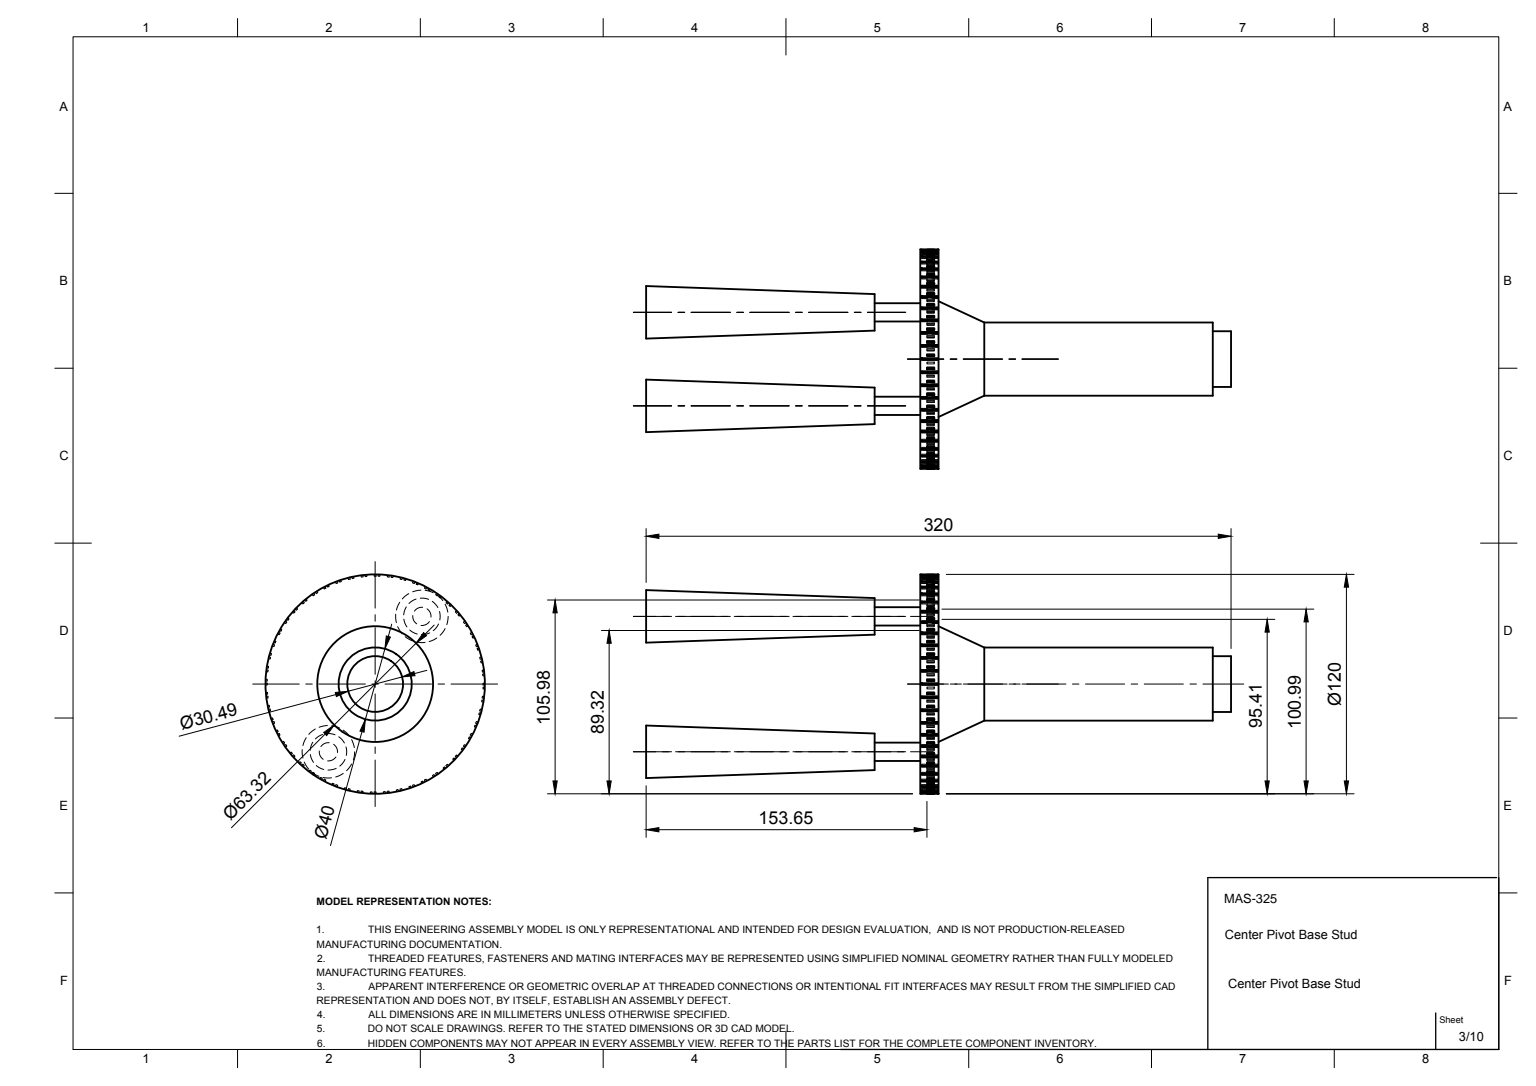
ISO-10303-21;
HEADER;
FILE_DESCRIPTION (('STEP AP214'),
    '1' );
FILE_NAME ('Center Pivot Base Stud.step',
    '2026-10-08T01:23:29',
    ( '' ),
    ( '' ),
    'SwSTEP 2.0',
    'SolidWorks 2025',
    '' );
FILE_SCHEMA (( 'AUTOMOTIVE_DESIGN' ));
ENDSEC;

DATA;
#6=EDGE_CURVE ( 'NONE', #30158, #26369, #45209, .T. ) ;
#7=DIRECTION ( 'NONE',  ( 1.000000000000000000, -0.000000000000000000, -0.000000000000000000 ) ) ;
#14=ORIENTED_EDGE ( 'NONE', *, *, #20809, .T. ) ;
#15=LINE ( 'NONE', #16057, #4072 ) ;
#25=CARTESIAN_POINT ( 'NONE',  ( -336.3521761649654422, -170.5607375887735770, 35.68215131113770155 ) ) ;
#29=DIRECTION ( 'NONE',  ( 0.000000000000000000, -0.3546048870425363986, -0.9350162426854146114 ) ) ;
#31=CARTESIAN_POINT ( 'NONE',  ( -339.1964088526558498, -131.1080185721124849, 58.50955523165764305 ) ) ;
#36=DIRECTION ( 'NONE',  ( -1.000000000000000000, -0.000000000000000000, -0.000000000000000000 ) ) ;
#38=( NAMED_UNIT ( * ) PLANE_ANGLE_UNIT ( ) SI_UNIT ( $, .RADIAN. ) );
#43=LINE ( 'NONE', #8442, #5592 ) ;
#45=ORIENTED_EDGE ( 'NONE', *, *, #35189, .T. ) ;
#47=FACE_OUTER_BOUND ( 'NONE', #8464, .T. ) ;
#52=DIRECTION ( 'NONE',  ( 0.000000000000000000, 1.341519488088730767E-14, -1.000000000000000000 ) ) ;
#54=AXIS2_PLACEMENT_3D ( 'NONE', #38179, #2187, #21657 ) ;
#55=CARTESIAN_POINT ( 'NONE',  ( -332.3517673607765914, -139.2044816956407089, -56.89493493766761389 ) ) ;
#59=CARTESIAN_POINT ( 'NONE',  ( -336.3521761649654422, -123.5000000000000284, 0.000000000000000000 ) ) ;
#60=CARTESIAN_POINT ( 'NONE',  ( -330.4913330509368166, -178.8432607619606358, 20.45418021416736565 ) ) ;
#64=ORIENTED_EDGE ( 'NONE', *, *, #9737, .T. ) ;
#65=CARTESIAN_POINT ( 'NONE',  ( -339.1964088526558498, -175.5095439275173135, 27.86139516340941213 ) ) ;
#66=CARTESIAN_POINT ( 'NONE',  ( -332.3517673607765914, -91.61526299123897843, -50.82679948493848343 ) ) ;
#69=VECTOR ( 'NONE', #22524, 1000.000000000000000 ) ;
#76=VERTEX_POINT ( 'NONE', #10211 ) ;
#77=VERTEX_POINT ( 'NONE', #49406 ) ;
#81=CARTESIAN_POINT ( 'NONE',  ( -330.4913330509368166, -183.4979166304964622, -0.4999999999999551470 ) ) ;
#87=LINE ( 'NONE', #8748, #33300 ) ;
#92=ORIENTED_EDGE ( 'NONE', *, *, #9964, .T. ) ;
#95=ORIENTED_EDGE ( 'NONE', *, *, #42836, .F. ) ;
#96=EDGE_CURVE ( 'NONE', #8568, #51994, #49908, .T. ) ;
#103=CARTESIAN_POINT ( 'NONE',  ( -336.3521761649654422, -123.5000000000000284, 0.000000000000000000 ) ) ;
#104=ORIENTED_EDGE ( 'NONE', *, *, #44978, .T. ) ;
#107=VECTOR ( 'NONE', #36864, 1000.000000000000000 ) ;
#110=DIRECTION ( 'NONE',  ( 1.000000000000000000, -0.000000000000000000, -0.000000000000000000 ) ) ;
#114=CARTESIAN_POINT ( 'NONE',  ( -339.1964088526558498, -122.9999999999993747, 59.00000000000002132 ) ) ;
#129=EDGE_LOOP ( 'NONE', ( #1022, #18617, #38243, #43508 ) ) ;
#135=ADVANCED_FACE ( 'NONE', ( #33613 ), #26232, .F. ) ;
#136=LINE ( 'NONE', #12733, #6804 ) ;
#141=EDGE_LOOP ( 'NONE', ( #33716, #13532, #31496, #14076 ) ) ;
#144=ADVANCED_FACE ( 'NONE', ( #30434 ), #14678, .T. ) ;
#146=DIRECTION ( 'NONE',  ( 0.000000000000000000, 0.000000000000000000, 1.000000000000000000 ) ) ;
#147=FACE_BOUND ( 'NONE', #3566, .T. ) ;
#149=EDGE_LOOP ( 'NONE', ( #37158, #34749, #12622, #8315 ) ) ;
#153=VERTEX_POINT ( 'NONE', #46748 ) ;
#154=CARTESIAN_POINT ( 'NONE',  ( -332.3517673607765914, -153.2494431741581025, -51.01861988938816950 ) ) ;
#155=EDGE_CURVE ( 'NONE', #5943, #22832, #22063, .T. ) ;
#160=ORIENTED_EDGE ( 'NONE', *, *, #6029, .T. ) ;
#161=LINE ( 'NONE', #28016, #26684 ) ;
#164=AXIS2_PLACEMENT_3D ( 'NONE', #24435, #20760, #36510 ) ;
#169=CARTESIAN_POINT ( 'NONE',  ( -336.3521761649654422, -161.4024510877913485, 45.24454186338643780 ) ) ;
#178=AXIS2_PLACEMENT_3D ( 'NONE', #15666, #4339, #31680 ) ;
#181=FACE_OUTER_BOUND ( 'NONE', #6191, .T. ) ;
#182=EDGE_CURVE ( 'NONE', #39742, #38924, #15463, .T. ) ;
#184=ADVANCED_FACE ( 'NONE', ( #15201 ), #27530, .F. ) ;
#186=VERTEX_POINT ( 'NONE', #51463 ) ;
#190=EDGE_LOOP ( 'NONE', ( #41506, #8467, #35219, #32996 ) ) ;
#191=AXIS2_PLACEMENT_3D ( 'NONE', #6779, #42505, #19123 ) ;
#197=ORIENTED_EDGE ( 'NONE', *, *, #15389, .T. ) ;
#198=ADVANCED_FACE ( 'NONE', ( #19392 ), #26495, .F. ) ;
#199=EDGE_LOOP ( 'NONE', ( #48171, #38497, #32246, #32492 ) ) ;
#200=DIRECTION ( 'NONE',  ( 0.000000000000000000, 0.2393156642875615969, 0.9709418174260511236 ) ) ;
#201=CARTESIAN_POINT ( 'NONE',  ( -339.1964088526558498, -180.9052250602809977, -13.63415328425247885 ) ) ;
#206=CARTESIAN_POINT ( 'NONE',  ( -332.3517673607765914, -86.34605966037949543, -45.90766452162698386 ) ) ;
#208=DIRECTION ( 'NONE',  ( 0.000000000000000000, 0.000000000000000000, 1.000000000000000000 ) ) ;
#214=CARTESIAN_POINT ( 'NONE',  ( -339.1964088526558498, -157.4273119900853146, -48.27201571435997352 ) ) ;
#216=CARTESIAN_POINT ( 'NONE',  ( -339.1964088526558498, -83.33976666098951114, 44.57752413667933666 ) ) ;
#217=ORIENTED_EDGE ( 'NONE', *, *, #6337, .T. ) ;
#222=DIRECTION ( 'NONE',  ( -0.000000000000000000, 0.2393156642875685636, 0.9709418174260492362 ) ) ;
#228=DIRECTION ( 'NONE',  ( 0.000000000000000000, 0.000000000000000000, 1.000000000000000000 ) ) ;
#232=VERTEX_POINT ( 'NONE', #18624 ) ;
#233=FACE_OUTER_BOUND ( 'NONE', #34259, .T. ) ;
#240=EDGE_CURVE ( 'NONE', #16530, #9197, #11238, .T. ) ;
#242=CYLINDRICAL_SURFACE ( 'NONE', #15746, 20.00000000000001066 ) ;
#256=DIRECTION ( 'NONE',  ( -0.000000000000000000, 0.8229838658936556861, -0.5680647467311569221 ) ) ;
#259=EDGE_CURVE ( 'NONE', #47910, #27371, #721, .T. ) ;
#260=CARTESIAN_POINT ( 'NONE',  ( -332.3517673607765914, -133.2247606357419443, -58.25253621232173629 ) ) ;
#261=ORIENTED_EDGE ( 'NONE', *, *, #51004, .T. ) ;
#264=EDGE_CURVE ( 'NONE', #15715, #30086, #23588, .T. ) ;
#269=ORIENTED_EDGE ( 'NONE', *, *, #12211, .F. ) ;
#276=ORIENTED_EDGE ( 'NONE', *, *, #30764, .F. ) ;
#284=LINE ( 'NONE', #32615, #29005 ) ;
#286=EDGE_CURVE ( 'NONE', #41564, #12706, #20162, .T. ) ;
#288=CARTESIAN_POINT ( 'NONE',  ( -332.3517673607765914, -139.4384828369889249, -57.84431488793872944 ) ) ;
#290=LINE ( 'NONE', #41018, #22829 ) ;
#298=CARTESIAN_POINT ( 'NONE',  ( -332.3517673607765914, -70.03480886230919111, 25.08789112700620194 ) ) ;
#301=ORIENTED_EDGE ( 'NONE', *, *, #17600, .T. ) ;
#304=VECTOR ( 'NONE', #6008, 999.9999999999998863 ) ;
#305=EDGE_CURVE ( 'NONE', #49014, #8114, #15730, .T. ) ;
#306=CARTESIAN_POINT ( 'NONE',  ( -305.0000000000000568, -71.64707600775140861, -30.18731974611341684 ) ) ;
#308=DIRECTION ( 'NONE',  ( -1.000000000000000000, 0.000000000000000000, 0.000000000000000000 ) ) ;
#315=LINE ( 'NONE', #15321, #378 ) ;
#316=CARTESIAN_POINT ( 'NONE',  ( -330.4913330509368166, -109.8658467157472813, -57.40522506028090532 ) ) ;
#325=DIRECTION ( 'NONE',  ( 0.000000000000000000, 0.2393156642875516049, -0.9709418174260534551 ) ) ;
#329=ORIENTED_EDGE ( 'NONE', *, *, #42921, .T. ) ;
#333=CARTESIAN_POINT ( 'NONE',  ( -330.4913330509368166, -75.22798428563987727, -33.92731199008506593 ) ) ;
#338=VECTOR ( 'NONE', #11663, 1000.000000000000000 ) ;
#339=ORIENTED_EDGE ( 'NONE', *, *, #31396, .F. ) ;
#340=CARTESIAN_POINT ( 'NONE',  ( -339.1964088526558498, -137.1341532842523065, 57.40522506028101901 ) ) ;
#343=CARTESIAN_POINT ( 'NONE',  ( -332.3517673607765914, -126.1322888500942270, -59.00000000000001421 ) ) ;
#344=DIRECTION ( 'NONE',  ( -1.000000000000000000, 0.000000000000000000, 0.000000000000000000 ) ) ;
#350=CARTESIAN_POINT ( 'NONE',  ( -332.3517673607765914, -65.24746378767824240, -9.724760635741734660 ) ) ;
#353=CARTESIAN_POINT ( 'NONE',  ( -332.3517673607765914, -135.2893155068536828, 58.83036664750491695 ) ) ;
#356=VECTOR ( 'NONE', #3324, 1000.000000000000000 ) ;
#358=ORIENTED_EDGE ( 'NONE', *, *, #16677, .F. ) ;
#359=DIRECTION ( 'NONE',  ( 1.000000000000000000, -0.000000000000000000, -0.000000000000000000 ) ) ;
#364=DIRECTION ( 'NONE',  ( -0.000000000000000000, -0.9350162426854132791, 0.3546048870425396182 ) ) ;
#365=CARTESIAN_POINT ( 'NONE',  ( -330.4913330509368166, -145.2430625708875880, -55.92172413327818958 ) ) ;
#366=DIRECTION ( 'NONE',  ( -8.718379230999707126E-17, 0.7485107481711024136, 0.6631226582407937498 ) ) ;
#368=EDGE_CURVE ( 'NONE', #39057, #30451, #5316, .T. ) ;
#369=LINE ( 'NONE', #36375, #20714 ) ;
#371=CARTESIAN_POINT ( 'NONE',  ( -336.3521761649654422, -135.0638248728647852, 57.91551518289418254 ) ) ;
#372=EDGE_LOOP ( 'NONE', ( #12308, #32950, #15983, #21673 ) ) ;
#373=ORIENTED_EDGE ( 'NONE', *, *, #33329, .T. ) ;
#374=DIRECTION ( 'NONE',  ( 0.000000000000000000, 0.7485107481711000821, -0.6631226582407965253 ) ) ;
#376=ORIENTED_EDGE ( 'NONE', *, *, #30512, .F. ) ;
#378=VECTOR ( 'NONE', #32371, 1000.000000000000114 ) ;
#379=EDGE_LOOP ( 'NONE', ( #7863, #48040, #19439, #9554 ) ) ;
#383=EDGE_LOOP ( 'NONE', ( #92, #27260, #27029, #39388 ) ) ;
#386=ORIENTED_EDGE ( 'NONE', *, *, #9915, .F. ) ;
#387=CARTESIAN_POINT ( 'NONE',  ( -339.1964088526558498, -123.5000000000000284, 0.000000000000000000 ) ) ;
#392=ORIENTED_EDGE ( 'NONE', *, *, #15989, .F. ) ;
#395=ORIENTED_EDGE ( 'NONE', *, *, #34509, .F. ) ;
#398=CARTESIAN_POINT ( 'NONE',  ( -332.3517673607765914, -174.5186198893880771, 29.74944317415823392 ) ) ;
#399=FACE_BOUND ( 'NONE', #32267, .T. ) ;
#400=DIRECTION ( 'NONE',  ( 0.000000000000000000, -0.8854560256532110207, -0.4647231720437664526 ) ) ;
#401=ORIENTED_EDGE ( 'NONE', *, *, #48751, .T. ) ;
#402=EDGE_CURVE ( 'NONE', #42461, #43377, #31986, .T. ) ;
#403=ORIENTED_EDGE ( 'NONE', *, *, #7972, .T. ) ;
#407=AXIS2_PLACEMENT_3D ( 'NONE', #634, #16408, #32423 ) ;
#412=CARTESIAN_POINT ( 'NONE',  ( -339.1964088526558498, -171.7720157143598669, 33.92731199008546383 ) ) ;
#422=DIRECTION ( 'NONE',  ( -0.000000000000000000, 0.2393156642875685636, 0.9709418174260492362 ) ) ;
#428=EDGE_CURVE ( 'NONE', #27513, #27045, #24890, .T. ) ;
#431=CARTESIAN_POINT ( 'NONE',  ( -305.0000000000000568, -104.7054247829104270, -56.98038208374144631 ) ) ;
#438=CARTESIAN_POINT ( 'NONE',  ( -332.3517673607765914, -64.87442053112221174, 12.76876783163883466 ) ) ;
#445=LINE ( 'NONE', #39606, #1079 ) ;
#446=ORIENTED_EDGE ( 'NONE', *, *, #50072, .F. ) ;
#448=VECTOR ( 'NONE', #9806, 999.9999999999998863 ) ;
#449=CIRCLE ( 'NONE', #45791, 60.00000000000000000 ) ;
#453=DIRECTION ( 'NONE',  ( -1.000000000000000000, -0.000000000000000000, 0.000000000000000000 ) ) ;
#458=LINE ( 'NONE', #21229, #24488 ) ;
#473=CARTESIAN_POINT ( 'NONE',  ( -305.0000000000000568, -150.9396941197155968, -53.35787839313373127 ) ) ;
#479=ORIENTED_EDGE ( 'NONE', *, *, #35123, .F. ) ;
#483=LINE ( 'NONE', #20735, #14074 ) ;
#491=DIRECTION ( 'NONE',  ( 0.000000000000000000, -0.4647231720437664526, 0.8854560256532110207 ) ) ;
#495=ORIENTED_EDGE ( 'NONE', *, *, #20083, .F. ) ;
#497=EDGE_CURVE ( 'NONE', #30653, #14763, #4477, .T. ) ;
#499=AXIS2_PLACEMENT_3D ( 'NONE', #42166, #25251, #24463 ) ;
#504=ORIENTED_EDGE ( 'NONE', *, *, #17516, .T. ) ;
#506=ORIENTED_EDGE ( 'NONE', *, *, #34160, .T. ) ;
#510=CARTESIAN_POINT ( 'NONE',  ( -336.3521761649654422, -87.81784868886214213, 47.06073758877343494 ) ) ;
#513=CARTESIAN_POINT ( 'NONE',  ( -330.4913330509368166, -89.82879061784696262, -49.66134974749687103 ) ) ;
#521=DIRECTION ( 'NONE',  ( 1.000000000000000000, -0.000000000000000000, -0.000000000000000000 ) ) ;
#522=AXIS2_PLACEMENT_3D ( 'NONE', #5834, #21590, #45254 ) ;
#526=LINE ( 'NONE', #16591, #33385 ) ;
#527=ORIENTED_EDGE ( 'NONE', *, *, #25028, .F. ) ;
#531=DIRECTION ( 'NONE',  ( 0.000000000000000000, 0.000000000000000000, -1.000000000000000000 ) ) ;
#534=DIRECTION ( 'NONE',  ( -1.000000000000000000, 0.000000000000000000, 0.000000000000000000 ) ) ;
#536=EDGE_LOOP ( 'NONE', ( #8280, #13076, #45536, #37068 ) ) ;
#538=ADVANCED_FACE ( 'NONE', ( #9385 ), #38000, .T. ) ;
#539=ADVANCED_FACE ( 'NONE', ( #1222 ), #33292, .T. ) ;
#544=CARTESIAN_POINT ( 'NONE',  ( -330.4913330509368166, -96.52406086224436876, -52.47426709956133806 ) ) ;
#548=DIRECTION ( 'NONE',  ( 0.000000000000000000, 1.156482317317871449E-14, 1.000000000000000000 ) ) ;
#549=CARTESIAN_POINT ( 'NONE',  ( -336.3521761649654422, -94.63601285149479736, 51.48334306143172512 ) ) ;
#552=EDGE_CURVE ( 'NONE', #15284, #26962, #8852, .T. ) ;
#557=ORIENTED_EDGE ( 'NONE', *, *, #40396, .F. ) ;
#559=EDGE_CURVE ( 'NONE', #4633, #10838, #13706, .T. ) ;
#566=AXIS2_PLACEMENT_3D ( 'NONE', #47062, #11037, #17979 ) ;
#567=VECTOR ( 'NONE', #28228, 1000.000000000000000 ) ;
#569=CARTESIAN_POINT ( 'NONE',  ( -339.1964088526558498, -84.75001853787809125, 44.49369547121489887 ) ) ;
#575=FACE_OUTER_BOUND ( 'NONE', #48196, .T. ) ;
#578=CARTESIAN_POINT ( 'NONE',  ( -330.4913330509368166, -157.4273119900845757, 48.27201571436049932 ) ) ;
#579=PLANE ( 'NONE',  #5256 ) ;
#582=VECTOR ( 'NONE', #15550, 1000.000000000000000 ) ;
#584=ORIENTED_EDGE ( 'NONE', *, *, #37671, .T. ) ;
#590=ORIENTED_EDGE ( 'NONE', *, *, #34142, .F. ) ;
#595=DIRECTION ( 'NONE',  ( -1.000000000000000000, 0.000000000000000000, -0.000000000000000000 ) ) ;
#607=CARTESIAN_POINT ( 'NONE',  ( -330.4913330509368166, -108.6560878169896256, 58.13482838284702581 ) ) ;
#617=EDGE_CURVE ( 'NONE', #30167, #21474, #51158, .T. ) ;
#619=CIRCLE ( 'NONE', #20770, 60.00000000000000000 ) ;
#620=ORIENTED_EDGE ( 'NONE', *, *, #35779, .F. ) ;
#623=CONICAL_SURFACE ( 'NONE', #29126, 10.00000000000000711, 0.03490658503988659789 ) ;
#625=EDGE_CURVE ( 'NONE', #8999, #27120, #46420, .T. ) ;
#626=EDGE_CURVE ( 'NONE', #50991, #48252, #50369, .T. ) ;
#629=DIRECTION ( 'NONE',  ( -1.000000000000000000, -0.000000000000000000, 0.000000000000000000 ) ) ;
#631=CARTESIAN_POINT ( 'NONE',  ( -365.0000000000001137, -78.50000000000002842, 0.000000000000000000 ) ) ;
#632=AXIS2_PLACEMENT_3D ( 'NONE', #7367, #43090, #14727 ) ;
#634=CARTESIAN_POINT ( 'NONE',  ( 0.000000000000000000, -162.6242368362065918, 44.16213414209531862 ) ) ;
#640=LINE ( 'NONE', #48731, #27621 ) ;
#647=DIRECTION ( 'NONE',  ( 0.000000000000000000, 0.1205366802553164696, -0.9927088740980548609 ) ) ;
#648=DIRECTION ( 'NONE',  ( 0.000000000000000000, 0.000000000000000000, -1.000000000000000000 ) ) ;
#658=ORIENTED_EDGE ( 'NONE', *, *, #5431, .T. ) ;
#660=DIRECTION ( 'NONE',  ( -0.000000000000000000, 0.6631226582407863113, -0.7485107481711089639 ) ) ;
#662=DIRECTION ( 'NONE',  ( -1.000000000000000000, 0.000000000000000000, -0.000000000000000000 ) ) ;
#663=VECTOR ( 'NONE', #44301, 1000.000000000000000 ) ;
#667=CARTESIAN_POINT ( 'NONE',  ( -330.4913330509368166, -150.4759391377553186, 52.47426709956150859 ) ) ;
#670=DIRECTION ( 'NONE',  ( -0.000000000000000000, 1.000000000000000000, -0.000000000000000000 ) ) ;
#674=VECTOR ( 'NONE', #17108, 1000.000000000000000 ) ;
#678=CARTESIAN_POINT ( 'NONE',  ( -305.0000000000000568, -123.5000000000000284, 0.000000000000000000 ) ) ;
#680=ORIENTED_EDGE ( 'NONE', *, *, #28374, .T. ) ;
#681=EDGE_CURVE ( 'NONE', #49313, #49622, #43755, .T. ) ;
#687=VECTOR ( 'NONE', #26344, 999.9999999999998863 ) ;
#693=VECTOR ( 'NONE', #26320, 1000.000000000000000 ) ;
#696=ORIENTED_EDGE ( 'NONE', *, *, #41387, .T. ) ;
#699=ORIENTED_EDGE ( 'NONE', *, *, #15129, .T. ) ;
#700=DIRECTION ( 'NONE',  ( 0.000000000000000000, -0.8854560256532093554, 0.4647231720437695057 ) ) ;
#706=CARTESIAN_POINT ( 'NONE',  ( -336.3521761649654422, -64.50000000000000000, -2.632288850093980503 ) ) ;
#711=LINE ( 'NONE', #28547, #40806 ) ;
#719=DIRECTION ( 'NONE',  ( 1.000000000000000000, 0.000000000000000000, 0.000000000000000000 ) ) ;
#720=ORIENTED_EDGE ( 'NONE', *, *, #4486, .T. ) ;
#721=LINE ( 'NONE', #24371, #22893 ) ;
#722=EDGE_LOOP ( 'NONE', ( #13255, #44779, #48049, #3646 ) ) ;
#724=AXIS2_PLACEMENT_3D ( 'NONE', #34745, #11088, #18732 ) ;
#725=VECTOR ( 'NONE', #35694, 1000.000000000000114 ) ;
#727=CARTESIAN_POINT ( 'NONE',  ( -330.4913330509368166, -131.1080185721124849, 58.50955523165764305 ) ) ;
#730=CARTESIAN_POINT ( 'NONE',  ( -332.3517673607765914, -170.5607375887735770, 35.68215131113770155 ) ) ;
#734=VECTOR ( 'NONE', #15159, 1000.000000000000000 ) ;
#739=DIRECTION ( 'NONE',  ( 1.000000000000000000, -7.719741424018441012E-17, 4.051632851310786670E-17 ) ) ;
#740=ADVANCED_FACE ( 'NONE', ( #35605 ), #3552, .F. ) ;
#748=ORIENTED_EDGE ( 'NONE', *, *, #46870, .F. ) ;
#750=EDGE_LOOP ( 'NONE', ( #47763, #48042, #43578, #36505 ) ) ;
#753=FACE_OUTER_BOUND ( 'NONE', #12516, .T. ) ;
#756=DIRECTION ( 'NONE',  ( 1.000000000000000000, -0.000000000000000000, 0.000000000000000000 ) ) ;
#759=ORIENTED_EDGE ( 'NONE', *, *, #12652, .T. ) ;
#761=CARTESIAN_POINT ( 'NONE',  ( -339.1964088526558498, -137.1341532842523065, 57.40522506028101901 ) ) ;
#764=CARTESIAN_POINT ( 'NONE',  ( -330.4913330509368166, -102.1108035431471279, 54.98865587491800255 ) ) ;
#771=LINE ( 'NONE', #21264, #26347 ) ;
#772=CARTESIAN_POINT ( 'NONE',  ( -339.1964088526558498, -79.66942718702493664, 39.49849221029193558 ) ) ;
#778=FACE_OUTER_BOUND ( 'NONE', #41872, .T. ) ;
#785=LINE ( 'NONE', #510, #16196 ) ;
#788=EDGE_CURVE ( 'NONE', #45751, #9248, #24559, .T. ) ;
#789=CARTESIAN_POINT ( 'NONE',  ( -330.4913330509368166, -183.1207326066167411, -6.735595255826296146 ) ) ;
#793=EDGE_CURVE ( 'NONE', #5683, #31493, #23789, .T. ) ;
#795=AXIS2_PLACEMENT_3D ( 'NONE', #19587, #662, #28498 ) ;
#798=VECTOR ( 'NONE', #3197, 1000.000000000000000 ) ;
#803=CARTESIAN_POINT ( 'NONE',  ( -332.3517673607765914, -100.1170788342122080, 54.23253582808833073 ) ) ;
#804=LINE ( 'NONE', #44961, #32554 ) ;
#809=VERTEX_POINT ( 'NONE', #15919 ) ;
#814=CARTESIAN_POINT ( 'NONE',  ( -339.1964088526558498, -175.9742670995615015, -26.97593913775538965 ) ) ;
#815=DIRECTION ( 'NONE',  ( -1.000000000000000000, -0.000000000000000000, -0.000000000000000000 ) ) ;
#816=ORIENTED_EDGE ( 'NONE', *, *, #28380, .T. ) ;
#820=DIRECTION ( 'NONE',  ( -0.000000000000000000, -0.9350162426854169428, -0.3546048870425300148 ) ) ;
#821=ORIENTED_EDGE ( 'NONE', *, *, #21477, .T. ) ;
#822=EDGE_CURVE ( 'NONE', #37318, #29662, #44017, .T. ) ;
#824=LINE ( 'NONE', #19745, #7267 ) ;
#825=FACE_OUTER_BOUND ( 'NONE', #25719, .T. ) ;
#826=ORIENTED_EDGE ( 'NONE', *, *, #45474, .F. ) ;
#830=CIRCLE ( 'NONE', #7550, 60.00000000000000000 ) ;
#831=LINE ( 'NONE', #36308, #22296 ) ;
#841=ORIENTED_EDGE ( 'NONE', *, *, #9249, .F. ) ;
#843=EDGE_CURVE ( 'NONE', #40953, #1071, #11946, .T. ) ;
#844=CARTESIAN_POINT ( 'NONE',  ( -336.3521761649654422, -123.5000000000000284, 0.000000000000000000 ) ) ;
#847=DIRECTION ( 'NONE',  ( 0.000000000000000000, 0.7485107481711089639, 0.6631226582407863113 ) ) ;
#852=EDGE_CURVE ( 'NONE', #6390, #47279, #33225, .T. ) ;
#855=ORIENTED_EDGE ( 'NONE', *, *, #4126, .F. ) ;
#857=EDGE_CURVE ( 'NONE', #42035, #39327, #29921, .T. ) ;
#862=VECTOR ( 'NONE', #6226, 1000.000000000000000 ) ;
#863=DIRECTION ( 'NONE',  ( 0.000000000000000000, 0.5680647467311540355, -0.8229838658936575735 ) ) ;
#865=DIRECTION ( 'NONE',  ( 0.000000000000000000, -0.8854560256532062468, 0.4647231720437755564 ) ) ;
#868=PLANE ( 'NONE',  #25728 ) ;
#872=ORIENTED_EDGE ( 'NONE', *, *, #17504, .T. ) ;
#873=FACE_OUTER_BOUND ( 'NONE', #29196, .T. ) ;
#879=FACE_BOUND ( 'NONE', #13817, .T. ) ;
#880=LINE ( 'NONE', #29514, #15543 ) ;
#884=PLANE ( 'NONE',  #11452 ) ;
#888=EDGE_LOOP ( 'NONE', ( #12030, #10347, #16731, #21899 ) ) ;
#892=DIRECTION ( 'NONE',  ( -0.000000000000000000, -0.1205366802553233113, -0.9927088740980538617 ) ) ;
#893=EDGE_LOOP ( 'NONE', ( #26823, #18504, #1153, #44757 ) ) ;
#898=VECTOR ( 'NONE', #3315, 1000.000000000000000 ) ;
#899=LINE ( 'NONE', #29006, #1687 ) ;
#900=CARTESIAN_POINT ( 'NONE',  ( -332.3517673607765914, -182.3871109312487420, -4.498567634386014369 ) ) ;
#901=EDGE_LOOP ( 'NONE', ( #1534, #46424, #46077, #38731 ) ) ;
#903=VERTEX_POINT ( 'NONE', #16950 ) ;
#907=ADVANCED_FACE ( 'NONE', ( #17209 ), #33746, .T. ) ;
#916=EDGE_CURVE ( 'NONE', #37855, #15026, #32709, .T. ) ;
#917=FACE_OUTER_BOUND ( 'NONE', #10592, .T. ) ;
#919=ORIENTED_EDGE ( 'NONE', *, *, #27607, .F. ) ;
#928=FACE_BOUND ( 'NONE', #50304, .T. ) ;
#931=ADVANCED_FACE ( 'NONE', ( #48753 ), #49009, .F. ) ;
#942=CARTESIAN_POINT ( 'NONE',  ( -365.0000000000001137, -78.50000000000002842, 0.000000000000000000 ) ) ;
#945=EDGE_LOOP ( 'NONE', ( #3380, #48657, #41462, #10623 ) ) ;
#957=AXIS2_PLACEMENT_3D ( 'NONE', #26370, #34508, #6419 ) ;
#960=ORIENTED_EDGE ( 'NONE', *, *, #47532, .T. ) ;
#965=ORIENTED_EDGE ( 'NONE', *, *, #13376, .F. ) ;
#966=EDGE_CURVE ( 'NONE', #23416, #47681, #16330, .T. ) ;
#969=VECTOR ( 'NONE', #7507, 1000.000000000000114 ) ;
#972=LINE ( 'NONE', #4397, #37714 ) ;
#977=ORIENTED_EDGE ( 'NONE', *, *, #49157, .F. ) ;
#978=VERTEX_POINT ( 'NONE', #36552 ) ;
#981=CARTESIAN_POINT ( 'NONE',  ( -339.1964088526558498, -137.3729703655840524, -58.37414404713467064 ) ) ;
#982=ADVANCED_FACE ( 'NONE', ( #8191 ), #44714, .F. ) ;
#988=VECTOR ( 'NONE', #34553, 1000.000000000000000 ) ;
#995=DIRECTION ( 'NONE',  ( -1.000000000000000000, -0.000000000000000000, -0.000000000000000000 ) ) ;
#1000=CARTESIAN_POINT ( 'NONE',  ( -336.3521761649654422, -77.59233547837267508, 37.15394033962009246 ) ) ;
#1001=VERTEX_POINT ( 'NONE', #8705 ) ;
#1003=DIRECTION ( 'NONE',  ( 0.000000000000000000, -0.7485107481711046340, -0.6631226582407911962 ) ) ;
#1008=ORIENTED_EDGE ( 'NONE', *, *, #2527, .F. ) ;
#1009=LINE ( 'NONE', #40954, #47226 ) ;
#1010=AXIS2_PLACEMENT_3D ( 'NONE', #24316, #19851, #28247 ) ;
#1016=DIRECTION ( 'NONE',  ( -0.000000000000000000, -0.6631226582407989678, -0.7485107481710977506 ) ) ;
#1021=CARTESIAN_POINT ( 'NONE',  ( -336.3521761649654422, -136.0347666902908372, 57.67619951860663718 ) ) ;
#1022=ORIENTED_EDGE ( 'NONE', *, *, #4950, .T. ) ;
#1023=AXIS2_PLACEMENT_3D ( 'NONE', #28600, #25706, #21511 ) ;
#1025=LINE ( 'NONE', #25468, #35362 ) ;
#1026=ORIENTED_EDGE ( 'NONE', *, *, #19388, .F. ) ;
#1027=EDGE_CURVE ( 'NONE', #12239, #8561, #37458, .T. ) ;
#1033=CARTESIAN_POINT ( 'NONE',  ( -336.3521761649653854, -167.3116148657362032, 40.99441916720376611 ) ) ;
#1036=DIRECTION ( 'NONE',  ( -1.000000000000000000, -0.000000000000000000, -0.000000000000000000 ) ) ;
#1046=VECTOR ( 'NONE', #42393, 999.9999999999998863 ) ;
#1049=DIRECTION ( 'NONE',  ( 1.000000000000000000, -0.000000000000000000, -0.000000000000000000 ) ) ;
#1050=CARTESIAN_POINT ( 'NONE',  ( 0.000000000000000000, -66.21443277186293130, -14.11962419296594362 ) ) ;
#1051=CARTESIAN_POINT ( 'NONE',  ( -330.4913330509368166, -138.1050951016791544, -57.16590939599326049 ) ) ;
#1053=DIRECTION ( 'NONE',  ( 0.000000000000000000, -0.9927088740980526405, 0.1205366802553337890 ) ) ;
#1054=ORIENTED_EDGE ( 'NONE', *, *, #47532, .F. ) ;
#1055=CARTESIAN_POINT ( 'NONE',  ( -330.4913330509368166, -162.9984922102926532, -43.83057281297441676 ) ) ;
#1056=ORIENTED_EDGE ( 'NONE', *, *, #35004, .T. ) ;
#1061=EDGE_CURVE ( 'NONE', #49231, #23542, #43, .T. ) ;
#1064=CYLINDRICAL_SURFACE ( 'NONE', #42444, 5.000000000000001776 ) ;
#1068=CARTESIAN_POINT ( 'NONE',  ( -339.1964088526558498, -64.50000000000000000, -0.5000000000000457412 ) ) ;
#1071=VERTEX_POINT ( 'NONE', #12382 ) ;
#1075=DIRECTION ( 'NONE',  ( 1.000000000000000000, 0.000000000000000000, -0.000000000000000000 ) ) ;
#1079=VECTOR ( 'NONE', #40641, 1000.000000000000000 ) ;
#1081=EDGE_CURVE ( 'NONE', #19973, #15758, #3891, .T. ) ;
#1085=FACE_OUTER_BOUND ( 'NONE', #1756, .T. ) ;
#1089=EDGE_CURVE ( 'NONE', #49077, #5683, #4772, .T. ) ;
#1091=ADVANCED_FACE ( 'NONE', ( #36295 ), #4248, .F. ) ;
#1096=AXIS2_PLACEMENT_3D ( 'NONE', #11928, #27966, #43997 ) ;
#1097=ORIENTED_EDGE ( 'NONE', *, *, #46194, .T. ) ;
#1100=CARTESIAN_POINT ( 'NONE',  ( -336.3521761649654422, -105.0395444947681369, -56.09938080879045685 ) ) ;
#1102=ORIENTED_EDGE ( 'NONE', *, *, #37849, .T. ) ;
#1103=EDGE_LOOP ( 'NONE', ( #16367, #2047, #5944, #42627, #29836, #15506, #24590, #45361, #42114, #27008, #14441, #17020 ) ) ;
#1105=EDGE_CURVE ( 'NONE', #9161, #6831, #824, .T. ) ;
#1107=DIRECTION ( 'NONE',  ( -0.000000000000000000, -0.2393156642875615969, -0.9709418174260511236 ) ) ;
#1113=AXIS2_PLACEMENT_3D ( 'NONE', #40879, #12244, #40608 ) ;
#1114=CARTESIAN_POINT ( 'NONE',  ( 0.000000000000000000, -89.98417994286192823, -48.55604808772582004 ) ) ;
#1128=VECTOR ( 'NONE', #19899, 1000.000000000000000 ) ;
#1133=CARTESIAN_POINT ( 'NONE',  ( -336.3521761649654422, -87.28260048324005993, 47.83617848703422482 ) ) ;
#1134=DIRECTION ( 'NONE',  ( 0.000000000000000000, 0.000000000000000000, 1.000000000000000000 ) ) ;
#1140=CARTESIAN_POINT ( 'NONE',  ( -332.3517673607765914, -158.3591674452439122, -47.62880233550485087 ) ) ;
#1143=PLANE ( 'NONE',  #12243 ) ;
#1145=LINE ( 'NONE', #9828, #29943 ) ;
#1148=CARTESIAN_POINT ( 'NONE',  ( -336.3521761649654422, -86.34605966037949543, -45.90766452162698386 ) ) ;
#1149=EDGE_CURVE ( 'NONE', #43162, #33480, #21057, .T. ) ;
#1152=ORIENTED_EDGE ( 'NONE', *, *, #33748, .T. ) ;
#1153=ORIENTED_EDGE ( 'NONE', *, *, #48129, .F. ) ;
#1154=EDGE_CURVE ( 'NONE', #5750, #45751, #25513, .T. ) ;
#1157=ORIENTED_EDGE ( 'NONE', *, *, #23110, .F. ) ;
#1158=EDGE_CURVE ( 'NONE', #13843, #41304, #13691, .T. ) ;
#1161=DIRECTION ( 'NONE',  ( 1.000000000000000000, -0.000000000000000000, -0.000000000000000000 ) ) ;
#1163=VERTEX_POINT ( 'NONE', #29709 ) ;
#1165=EDGE_LOOP ( 'NONE', ( #35019, #7711, #18752, #10228 ) ) ;
#1168=AXIS2_PLACEMENT_3D ( 'NONE', #5085, #48965, #865 ) ;
#1170=PLANE ( 'NONE',  #26072 ) ;
#1172=ORIENTED_EDGE ( 'NONE', *, *, #26251, .T. ) ;
#1173=ORIENTED_EDGE ( 'NONE', *, *, #32356, .T. ) ;
#1183=CARTESIAN_POINT ( 'NONE',  ( -339.1964088526558498, -179.7763290203209863, -20.80804632820157352 ) ) ;
#1188=EDGE_CURVE ( 'NONE', #36786, #30970, #9749, .T. ) ;
#1193=ORIENTED_EDGE ( 'NONE', *, *, #96, .F. ) ;
#1197=ORIENTED_EDGE ( 'NONE', *, *, #13985, .T. ) ;
#1199=EDGE_CURVE ( 'NONE', #48562, #22978, #48420, .T. ) ;
#1201=ORIENTED_EDGE ( 'NONE', *, *, #11281, .F. ) ;
#1202=ADVANCED_FACE ( 'NONE', ( #12902 ), #28923, .F. ) ;
#1203=VECTOR ( 'NONE', #7902, 1000.000000000000114 ) ;
#1204=VECTOR ( 'NONE', #27394, 1000.000000000000000 ) ;
#1205=CARTESIAN_POINT ( 'NONE',  ( -339.1964088526558498, -64.99044476834235695, 7.608018572112245970 ) ) ;
#1206=CARTESIAN_POINT ( 'NONE',  ( -330.4913330509368166, -102.6919536717981742, -56.27632902032085838 ) ) ;
#1207=CARTESIAN_POINT ( 'NONE',  ( -336.3521761649654422, -174.5186198893880771, 29.74944317415823392 ) ) ;
#1208=EDGE_CURVE ( 'NONE', #14314, #3375, #7100, .T. ) ;
#1209=DIRECTION ( 'NONE',  ( -0.000000000000000000, 0.9350162426854194964, 0.3546048870425235200 ) ) ;
#1210=CARTESIAN_POINT ( 'NONE',  ( -332.3517673607765914, -164.5945333327934463, -42.41660376256285048 ) ) ;
#1222=FACE_OUTER_BOUND ( 'NONE', #32568, .T. ) ;
#1227=DIRECTION ( 'NONE',  ( -0.000000000000000000, 0.9709418174260553425, 0.2393156642875449158 ) ) ;
#1231=ORIENTED_EDGE ( 'NONE', *, *, #40377, .F. ) ;
#1235=LINE ( 'NONE', #25936, #47834 ) ;
#1242=VECTOR ( 'NONE', #4530, 1000.000000000000000 ) ;
#1249=DIRECTION ( 'NONE',  ( -1.000000000000000000, 0.000000000000000000, 0.000000000000000000 ) ) ;
#1251=VERTEX_POINT ( 'NONE', #10783 ) ;
#1252=VECTOR ( 'NONE', #11527, 1000.000000000000000 ) ;
#1253=ORIENTED_EDGE ( 'NONE', *, *, #24527, .T. ) ;
#1257=EDGE_CURVE ( 'NONE', #33644, #3411, #30240, .T. ) ;
#1259=ADVANCED_FACE ( 'NONE', ( #22618 ), #14476, .T. ) ;
#1261=CARTESIAN_POINT ( 'NONE',  ( -339.1964088526558498, -84.75001853787809125, 44.49369547121489887 ) ) ;
#1266=EDGE_CURVE ( 'NONE', #28257, #8870, #18418, .T. ) ;
#1270=DIRECTION ( 'NONE',  ( 0.000000000000000000, -7.725301879683381348E-14, -1.000000000000000000 ) ) ;
#1271=CARTESIAN_POINT ( 'NONE',  ( 0.000000000000000000, -84.37576316379256980, 44.16213414209452992 ) ) ;
#1274=DIRECTION ( 'NONE',  ( 1.000000000000000000, -0.000000000000000000, -0.000000000000000000 ) ) ;
#1276=DIRECTION ( 'NONE',  ( 1.000000000000000000, -0.000000000000000000, -0.000000000000000000 ) ) ;
#1278=DIRECTION ( 'NONE',  ( 1.000000000000000000, 8.465038975556407387E-17, 2.086444717177515993E-17 ) ) ;
#1279=CARTESIAN_POINT ( 'NONE',  ( -336.3521761649654422, -152.3639871485048900, -51.48334306143194539 ) ) ;
#1283=ADVANCED_FACE ( 'NONE', ( #31006 ), #43091, .F. ) ;
#1285=AXIS2_PLACEMENT_3D ( 'NONE', #35926, #11741, #11484 ) ;
#1289=ORIENTED_EDGE ( 'NONE', *, *, #2143, .F. ) ;
#1293=EDGE_CURVE ( 'NONE', #32812, #28636, #36675, .T. ) ;
#1297=PLANE ( 'NONE',  #40483 ) ;
#1299=CIRCLE ( 'NONE', #39875, 60.00000000000000000 ) ;
#1308=VECTOR ( 'NONE', #44248, 1000.000000000000000 ) ;
#1310=ORIENTED_EDGE ( 'NONE', *, *, #47140, .T. ) ;
#1313=LINE ( 'NONE', #21035, #20954 ) ;
#1314=FACE_OUTER_BOUND ( 'NONE', #49501, .T. ) ;
#1318=ORIENTED_EDGE ( 'NONE', *, *, #36446, .T. ) ;
#1323=CARTESIAN_POINT ( 'NONE',  ( -332.3517673607765914, -180.4803820837415458, -18.79457521708939183 ) ) ;
#1325=CIRCLE ( 'NONE', #49993, 60.00000000000000000 ) ;
#1327=ADVANCED_FACE ( 'NONE', ( #28604 ), #15503, .F. ) ;
#1332=EDGE_LOOP ( 'NONE', ( #38979, #26674, #17451, #47872 ) ) ;
#1334=CARTESIAN_POINT ( 'NONE',  ( -339.1964088526558498, -109.8658467157473666, -57.40522506028092664 ) ) ;
#1335=LINE ( 'NONE', #41270, #48338 ) ;
#1338=DIRECTION ( 'NONE',  ( -1.000000000000000000, 0.000000000000000000, -0.000000000000000000 ) ) ;
#1342=CARTESIAN_POINT ( 'NONE',  ( -339.1964088526558498, -167.9936954712156592, -38.74998146212110584 ) ) ;
#1344=AXIS2_PLACEMENT_3D ( 'NONE', #32340, #36546, #548 ) ;
#1345=CARTESIAN_POINT ( 'NONE',  ( -332.3517673607765914, -133.2247606357419443, -58.25253621232173629 ) ) ;
#1348=CARTESIAN_POINT ( 'NONE',  ( -339.1964088526558498, -90.39567187580801999, 48.84008046109089918 ) ) ;
#1351=CARTESIAN_POINT ( 'NONE',  ( -336.3521761649654422, -125.1322888500942270, -59.00000000000002132 ) ) ;
#1354=DIRECTION ( 'NONE',  ( -0.000000000000000000, 0.7485107481711089639, 0.6631226582407863113 ) ) ;
#1359=DIRECTION ( 'NONE',  ( -0.000000000000000000, 0.9709418174260544543, 0.2393156642875482465 ) ) ;
#1360=DIRECTION ( 'NONE',  ( 0.000000000000000000, 0.000000000000000000, 1.000000000000000000 ) ) ;
#1361=DIRECTION ( 'NONE',  ( 0.000000000000000000, -0.5680647467311625842, -0.8229838658936516893 ) ) ;
#1366=PLANE ( 'NONE',  #33333 ) ;
#1367=DIRECTION ( 'NONE',  ( 0.000000000000000000, 0.000000000000000000, -1.000000000000000000 ) ) ;
#1373=ORIENTED_EDGE ( 'NONE', *, *, #19823, .T. ) ;
#1395=EDGE_CURVE ( 'NONE', #22171, #8674, #44653, .T. ) ;
#1396=VECTOR ( 'NONE', #49263, 1000.000000000000000 ) ;
#1401=ORIENTED_EDGE ( 'NONE', *, *, #39450, .F. ) ;
#1405=FACE_BOUND ( 'NONE', #49064, .T. ) ;
#1408=CARTESIAN_POINT ( 'NONE',  ( -330.4913330509368166, -70.14212160686619768, -27.43969411971537298 ) ) ;
#1412=VECTOR ( 'NONE', #14848, 1000.000000000000114 ) ;
#1429=LINE ( 'NONE', #46361, #45515 ) ;
#1436=VERTEX_POINT ( 'NONE', #7861 ) ;
#1439=DIRECTION ( 'NONE',  ( 1.000000000000000000, -0.000000000000000000, 0.000000000000000000 ) ) ;
#1440=DIRECTION ( 'NONE',  ( 1.000000000000000000, -0.000000000000000000, -0.000000000000000000 ) ) ;
#1445=ORIENTED_EDGE ( 'NONE', *, *, #36918, .F. ) ;
#1449=CARTESIAN_POINT ( 'NONE',  ( -336.3521761649654422, -158.3591674452439122, -47.62880233550485087 ) ) ;
#1450=DIRECTION ( 'NONE',  ( 0.000000000000000000, -0.6631226582408039638, -0.7485107481710934207 ) ) ;
#1453=VECTOR ( 'NONE', #27230, 1000.000000000000000 ) ;
#1457=EDGE_CURVE ( 'NONE', #13383, #6473, #40682, .T. ) ;
#1462=ORIENTED_EDGE ( 'NONE', *, *, #7208, .F. ) ;
#1463=DIRECTION ( 'NONE',  ( 1.043714542225393697E-14, 0.2393156642875652051, 0.9709418174260502354 ) ) ;
#1467=EDGE_CURVE ( 'NONE', #44354, #3275, #3933, .T. ) ;
#1468=DIRECTION ( 'NONE',  ( 1.000000000000000000, -0.000000000000000000, 0.000000000000000000 ) ) ;
#1470=CARTESIAN_POINT ( 'NONE',  ( -339.1964088526558498, -180.6659093959932250, 14.60509510167942437 ) ) ;
#1471=CARTESIAN_POINT ( 'NONE',  ( -305.0000000000000568, -136.2687678316390532, 58.62557946887775273 ) ) ;
#1475=EDGE_LOOP ( 'NONE', ( #14015, #32657, #16736, #7496 ) ) ;
#1477=VECTOR ( 'NONE', #36099, 1000.000000000000227 ) ;
#1481=AXIS2_PLACEMENT_3D ( 'NONE', #844, #9003, #25805 ) ;
#1483=DIRECTION ( 'NONE',  ( 0.000000000000000000, -0.9927088740980548609, -0.1205366802553164696 ) ) ;
#1487=DIRECTION ( 'NONE',  ( -0.000000000000000000, -1.000000000000000000, 3.491481338843133355E-15 ) ) ;
#1489=VECTOR ( 'NONE', #48761, 1000.000000000000000 ) ;
#1494=ORIENTED_EDGE ( 'NONE', *, *, #1571, .T. ) ;
#1495=AXIS2_PLACEMENT_3D ( 'NONE', #23370, #3637, #3381 ) ;
#1498=CARTESIAN_POINT ( 'NONE',  ( -332.3517673607765914, -123.5000000000000284, 0.000000000000000000 ) ) ;
#1505=VERTEX_POINT ( 'NONE', #7204 ) ;
#1506=DIRECTION ( 'NONE',  ( -0.000000000000000000, -0.9927088740980530845, 0.1205366802553303057 ) ) ;
#1507=AXIS2_PLACEMENT_3D ( 'NONE', #18467, #14795, #22151 ) ;
#1510=ORIENTED_EDGE ( 'NONE', *, *, #25715, .F. ) ;
#1514=LINE ( 'NONE', #48837, #36407 ) ;
#1520=DIRECTION ( 'NONE',  ( 0.000000000000000000, 1.137978600240785454E-13, -1.000000000000000000 ) ) ;
#1521=ORIENTED_EDGE ( 'NONE', *, *, #13723, .T. ) ;
#1522=DIRECTION ( 'NONE',  ( 0.000000000000000000, 0.000000000000000000, 1.000000000000000000 ) ) ;
#1525=VERTEX_POINT ( 'NONE', #6945 ) ;
#1527=VERTEX_POINT ( 'NONE', #43193 ) ;
#1531=ADVANCED_FACE ( 'NONE', ( #19302 ), #22974, .F. ) ;
#1534=ORIENTED_EDGE ( 'NONE', *, *, #21442, .F. ) ;
#1535=DIRECTION ( 'NONE',  ( 0.000000000000000000, 0.000000000000000000, -1.000000000000000000 ) ) ;
#1538=ORIENTED_EDGE ( 'NONE', *, *, #40564, .T. ) ;
#1541=FACE_OUTER_BOUND ( 'NONE', #22455, .T. ) ;
#1549=DIRECTION ( 'NONE',  ( 0.000000000000000000, 3.561965537339043690E-14, 1.000000000000000000 ) ) ;
#1552=VERTEX_POINT ( 'NONE', #11387 ) ;
#1553=VECTOR ( 'NONE', #42887, 1000.000000000000114 ) ;
#1560=ORIENTED_EDGE ( 'NONE', *, *, #31455, .F. ) ;
#1562=ORIENTED_EDGE ( 'NONE', *, *, #29542, .F. ) ;
#1563=EDGE_CURVE ( 'NONE', #29872, #35764, #38985, .T. ) ;
#1564=AXIS2_PLACEMENT_3D ( 'NONE', #7827, #453, #36733 ) ;
#1571=EDGE_CURVE ( 'NONE', #13360, #44682, #27937, .T. ) ;
#1573=EDGE_CURVE ( 'NONE', #16038, #8568, #35063, .T. ) ;
#1574=CARTESIAN_POINT ( 'NONE',  ( -339.1964088526558498, -182.5000000000000568, 0.5000000000000457412 ) ) ;
#1576=EDGE_CURVE ( 'NONE', #38828, #26805, #47678, .T. ) ;
#1578=CARTESIAN_POINT ( 'NONE',  ( -336.3521761649654422, -163.8460225846223466, -43.07972642080364523 ) ) ;
#1582=EDGE_CURVE ( 'NONE', #28072, #40574, #34159, .T. ) ;
#1586=EDGE_CURVE ( 'NONE', #7784, #2629, #11903, .T. ) ;
#1588=DIRECTION ( 'NONE',  ( -0.000000000000000000, 0.000000000000000000, 1.000000000000000000 ) ) ;
#1590=CARTESIAN_POINT ( 'NONE',  ( -330.4913330509368166, -101.7569374291120710, 55.92172413327804037 ) ) ;
#1591=CARTESIAN_POINT ( 'NONE',  ( -339.1964088526558498, -123.5000000000000284, 0.000000000000000000 ) ) ;
#1595=AXIS2_PLACEMENT_3D ( 'NONE', #25690, #45671, #48842 ) ;
#1597=ORIENTED_EDGE ( 'NONE', *, *, #23576, .F. ) ;
#1598=CARTESIAN_POINT ( 'NONE',  ( -339.1964088526558498, -138.1050951016792681, -57.16590939599323917 ) ) ;
#1604=CARTESIAN_POINT ( 'NONE',  ( -339.1964088526558498, -183.4979166304964622, 0.5000000000000457412 ) ) ;
#1606=VERTEX_POINT ( 'NONE', #4286 ) ;
#1607=ADVANCED_FACE ( 'NONE', ( #45295 ), #28189, .F. ) ;
#1625=CARTESIAN_POINT ( 'NONE',  ( -339.1964088526558498, -116.8846903019852164, -58.63009191191289915 ) ) ;
#1635=VECTOR ( 'NONE', #40333, 1000.000000000000114 ) ;
#1636=VERTEX_POINT ( 'NONE', #81 ) ;
#1646=ORIENTED_EDGE ( 'NONE', *, *, #11005, .T. ) ;
#1653=PLANE ( 'NONE',  #16580 ) ;
#1662=DIRECTION ( 'NONE',  ( 0.000000000000000000, 0.000000000000000000, -1.000000000000000000 ) ) ;
#1663=EDGE_CURVE ( 'NONE', #6375, #21742, #5341, .T. ) ;
#1674=ORIENTED_EDGE ( 'NONE', *, *, #37092, .F. ) ;
#1675=DIRECTION ( 'NONE',  ( 1.000000000000000000, 0.000000000000000000, -0.000000000000000000 ) ) ;
#1676=ORIENTED_EDGE ( 'NONE', *, *, #27684, .T. ) ;
#1679=FACE_OUTER_BOUND ( 'NONE', #11462, .T. ) ;
#1687=VECTOR ( 'NONE', #13517, 999.9999999999998863 ) ;
#1689=EDGE_LOOP ( 'NONE', ( #8500, #18459, #42674, #33934 ) ) ;
#1695=EDGE_CURVE ( 'NONE', #32525, #6745, #4548, .T. ) ;
#1701=PLANE ( 'NONE',  #14933 ) ;
#1704=CARTESIAN_POINT ( 'NONE',  ( -339.1964088526558498, -162.2499814621209850, 44.49369547121574442 ) ) ;
#1707=LINE ( 'NONE', #33763, #11529 ) ;
#1708=CARTESIAN_POINT ( 'NONE',  ( -336.3521761649654422, -135.0638248728647852, 57.91551518289418254 ) ) ;
#1709=ADVANCED_FACE ( 'NONE', ( #24267 ), #623, .T. ) ;
#1714=VECTOR ( 'NONE', #20843, 1000.000000000000114 ) ;
#1717=DIRECTION ( 'NONE',  ( 1.000000000000000000, 0.000000000000000000, 0.000000000000000000 ) ) ;
#1719=ORIENTED_EDGE ( 'NONE', *, *, #6024, .F. ) ;
#1722=CARTESIAN_POINT ( 'NONE',  ( -332.3517673607765914, -164.5945333327934463, -42.41660376256285048 ) ) ;
#1737=CARTESIAN_POINT ( 'NONE',  ( -336.3521761649654422, -67.40061919120938683, 18.46045550523129819 ) ) ;
#1744=ORIENTED_EDGE ( 'NONE', *, *, #17339, .T. ) ;
#1746=VERTEX_POINT ( 'NONE', #45540 ) ;
#1750=ADVANCED_FACE ( 'NONE', ( #6121 ), #6370, .F. ) ;
#1752=DIRECTION ( 'NONE',  ( 0.000000000000000000, -0.5680647467311626952, -0.8229838658936516893 ) ) ;
#1756=EDGE_LOOP ( 'NONE', ( #15179, #20096, #4669, #44013 ) ) ;
#1759=ORIENTED_EDGE ( 'NONE', *, *, #9446, .T. ) ;
#1760=ORIENTED_EDGE ( 'NONE', *, *, #31097, .T. ) ;
#1765=DIRECTION ( 'NONE',  ( 0.000000000000000000, 0.4647231720437604574, -0.8854560256532141294 ) ) ;
#1766=CARTESIAN_POINT ( 'NONE',  ( -305.0000000000000568, -63.99980407363855761, 7.728304129923848187 ) ) ;
#1767=DIRECTION ( 'NONE',  ( -0.000000000000000000, -3.491481338843133355E-15, -1.000000000000000000 ) ) ;
#1768=ORIENTED_EDGE ( 'NONE', *, *, #15904, .T. ) ;
#1769=CARTESIAN_POINT ( 'NONE',  ( -336.3521761649654422, -148.5878911270064009, 53.46519113769075204 ) ) ;
#1770=DIRECTION ( 'NONE',  ( 1.000000000000000000, 0.000000000000000000, 0.000000000000000000 ) ) ;
#1779=CARTESIAN_POINT ( 'NONE',  ( -305.0000000000000568, -183.0001959263613855, 7.728304129924832289 ) ) ;
#1784=VECTOR ( 'NONE', #46616, 1000.000000000000000 ) ;
#1788=VECTOR ( 'NONE', #41619, 1000.000000000000000 ) ;
#1789=LINE ( 'NONE', #50165, #49053 ) ;
#1801=ORIENTED_EDGE ( 'NONE', *, *, #43259, .F. ) ;
#1802=AXIS2_PLACEMENT_3D ( 'NONE', #13725, #45792, #25814 ) ;
#1809=ORIENTED_EDGE ( 'NONE', *, *, #19299, .F. ) ;
#1810=EDGE_CURVE ( 'NONE', #4093, #30219, #10056, .T. ) ;
#1812=EDGE_CURVE ( 'NONE', #51297, #50020, #30526, .T. ) ;
#1813=CARTESIAN_POINT ( 'NONE',  ( -336.3521761649654422, -74.01670616005314685, 32.17247266903214609 ) ) ;
#1815=AXIS2_PLACEMENT_3D ( 'NONE', #21198, #8582, #37481 ) ;
#1834=DIRECTION ( 'NONE',  ( 1.000000000000000000, -0.000000000000000000, -0.000000000000000000 ) ) ;
#1835=ORIENTED_EDGE ( 'NONE', *, *, #45833, .F. ) ;
#1837=DIRECTION ( 'NONE',  ( 0.000000000000000000, -0.9709418174260553425, -0.2393156642875449158 ) ) ;
#1839=CARTESIAN_POINT ( 'NONE',  ( -336.3521761649654422, -72.48138011061176655, -29.74944317415788930 ) ) ;
#1841=DIRECTION ( 'NONE',  ( 1.000000000000000000, -0.000000000000000000, 0.000000000000000000 ) ) ;
#1842=CARTESIAN_POINT ( 'NONE',  ( -339.1964088526558498, -123.5000000000000284, 0.000000000000000000 ) ) ;
#1846=CARTESIAN_POINT ( 'NONE',  ( -339.1964088526558498, -71.02573290043878274, -26.97593913775585506 ) ) ;
#1851=DIRECTION ( 'NONE',  ( 1.000000000000000000, 0.000000000000000000, -1.043714542225393381E-14 ) ) ;
#1855=LINE ( 'NONE', #17898, #8115 ) ;
#1856=ADVANCED_FACE ( 'NONE', ( #21628 ), #1653, .F. ) ;
#1859=ADVANCED_FACE ( 'NONE', ( #35241 ), #42873, .F. ) ;
#1861=DIRECTION ( 'NONE',  ( -1.000000000000000000, 0.000000000000000000, 0.000000000000000000 ) ) ;
#1864=VECTOR ( 'NONE', #21546, 1000.000000000000000 ) ;
#1867=CARTESIAN_POINT ( 'NONE',  ( -336.3521761649653854, -179.0013928959018301, 22.79463504017430253 ) ) ;
#1868=ADVANCED_FACE ( 'NONE', ( #3439 ), #7408, .F. ) ;
#1870=CARTESIAN_POINT ( 'NONE',  ( -332.3517673607765914, -73.44864141332200802, 31.34948880313848107 ) ) ;
#1871=CARTESIAN_POINT ( 'NONE',  ( -332.3517673607765914, -77.59233547837267508, 37.15394033962009246 ) ) ;
#1878=AXIS2_PLACEMENT_3D ( 'NONE', #2232, #25370, #49811 ) ;
#1879=EDGE_CURVE ( 'NONE', #46919, #4457, #35494, .T. ) ;
#1883=ORIENTED_EDGE ( 'NONE', *, *, #7669, .F. ) ;
#1886=EDGE_CURVE ( 'NONE', #28559, #24027, #39439, .T. ) ;
#1904=DIRECTION ( 'NONE',  ( -0.000000000000000000, 0.8854560256532157947, 0.4647231720437573488 ) ) ;
#1908=CARTESIAN_POINT ( 'NONE',  ( -336.3521761649654422, -93.75055682584159911, 51.01861988938794923 ) ) ;
#1912=EDGE_CURVE ( 'NONE', #27843, #10230, #39684, .T. ) ;
#1913=AXIS2_PLACEMENT_3D ( 'NONE', #1737, #10140, #42450 ) ;
#1916=CARTESIAN_POINT ( 'NONE',  ( -339.1964088526558498, -123.5000000000000284, 0.000000000000000000 ) ) ;
#1920=EDGE_CURVE ( 'NONE', #17726, #14905, #18228, .T. ) ;
#1923=LINE ( 'NONE', #21903, #35115 ) ;
#1927=EDGE_CURVE ( 'NONE', #47587, #12138, #10824, .T. ) ;
#1928=ORIENTED_EDGE ( 'NONE', *, *, #26949, .T. ) ;
#1929=DIRECTION ( 'NONE',  ( -1.000000000000000000, 0.000000000000000000, 0.000000000000000000 ) ) ;
#1930=EDGE_LOOP ( 'NONE', ( #40310, #22970, #23601, #11830 ) ) ;
#1936=LINE ( 'NONE', #46607, #14327 ) ;
#1939=LINE ( 'NONE', #2902, #37484 ) ;
#1940=VECTOR ( 'NONE', #19020, 1000.000000000000000 ) ;
#1947=VERTEX_POINT ( 'NONE', #15814 ) ;
#1948=ADVANCED_FACE ( 'NONE', ( #34993 ), #19234, .T. ) ;
#1950=AXIS2_PLACEMENT_3D ( 'NONE', #27832, #15510, #34947 ) ;
#1951=CIRCLE ( 'NONE', #31311, 60.00000000000000000 ) ;
#1953=CARTESIAN_POINT ( 'NONE',  ( 0.000000000000000000, -157.0158200571384555, -48.55604808772557845 ) ) ;
#1954=AXIS2_PLACEMENT_3D ( 'NONE', #18171, #34197, #50244 ) ;
#1956=DIRECTION ( 'NONE',  ( 0.000000000000000000, -0.6631226582408016323, -0.7485107481710953081 ) ) ;
#1959=FACE_OUTER_BOUND ( 'NONE', #33108, .T. ) ;
#1962=DIRECTION ( 'NONE',  ( 0.000000000000000000, -0.7485107481711069655, -0.6631226582407885317 ) ) ;
#1965=ORIENTED_EDGE ( 'NONE', *, *, #42964, .T. ) ;
#1970=VECTOR ( 'NONE', #18162, 1000.000000000000000 ) ;
#1973=VERTEX_POINT ( 'NONE', #25 ) ;
#1974=CARTESIAN_POINT ( 'NONE',  ( -332.3517673607765914, -155.3847370087607374, 50.82679948493869659 ) ) ;
#1977=PLANE ( 'NONE',  #35888 ) ;
#1979=ADVANCED_FACE ( 'NONE', ( #44168 ), #48117, .F. ) ;
#1980=LINE ( 'NONE', #18021, #12520 ) ;
#1981=EDGE_CURVE ( 'NONE', #42791, #45363, #44962, .T. ) ;
#1983=LINE ( 'NONE', #50091, #17513 ) ;
#1987=VECTOR ( 'NONE', #34606, 1000.000000000000000 ) ;
#1999=AXIS2_PLACEMENT_3D ( 'NONE', #25208, #41218, #22033 ) ;
#2000=ORIENTED_EDGE ( 'NONE', *, *, #44753, .F. ) ;
#2002=EDGE_LOOP ( 'NONE', ( #49489, #38026, #38115, #8416 ) ) ;
#2004=ADVANCED_FACE ( 'NONE', ( #8171 ), #21038, .T. ) ;
#2005=CARTESIAN_POINT ( 'NONE',  ( -336.3521761649654422, -148.5878911270064009, 53.46519113769075204 ) ) ;
#2007=CARTESIAN_POINT ( 'NONE',  ( -305.0000000000000568, -73.21199843436539823, 32.72792230702599170 ) ) ;
#2008=VERTEX_POINT ( 'NONE', #24990 ) ;
#2009=CARTESIAN_POINT ( 'NONE',  ( -336.3521761649654422, -123.5000000000000284, 0.000000000000000000 ) ) ;
#2010=EDGE_CURVE ( 'NONE', #11472, #15531, #36026, .T. ) ;
#2011=DIRECTION ( 'NONE',  ( -1.000000000000000000, -0.000000000000000000, -0.000000000000000000 ) ) ;
#2013=DIRECTION ( 'NONE',  ( -0.000000000000000000, 0.8854560256532093554, -0.4647231720437695057 ) ) ;
#2021=DIRECTION ( 'NONE',  ( 0.000000000000000000, 0.000000000000000000, -1.000000000000000000 ) ) ;
#2022=ORIENTED_EDGE ( 'NONE', *, *, #31396, .T. ) ;
#2023=EDGE_CURVE ( 'NONE', #10439, #23203, #48650, .T. ) ;
#2029=DIRECTION ( 'NONE',  ( 1.000000000000000000, 0.000000000000000000, -0.000000000000000000 ) ) ;
#2033=ORIENTED_EDGE ( 'NONE', *, *, #3479, .F. ) ;
#2034=VECTOR ( 'NONE', #30484, 1000.000000000000000 ) ;
#2047=ORIENTED_EDGE ( 'NONE', *, *, #28252, .T. ) ;
#2048=DIRECTION ( 'NONE',  ( -0.000000000000000000, 0.4647231720437755564, 0.8854560256532062468 ) ) ;
#2057=DIRECTION ( 'NONE',  ( -1.000000000000000000, 0.000000000000000000, 0.000000000000000000 ) ) ;
#2059=EDGE_CURVE ( 'NONE', #15758, #21929, #28386, .T. ) ;
#2060=DIRECTION ( 'NONE',  ( -1.000000000000000000, 0.000000000000000000, 0.000000000000000000 ) ) ;
#2074=PLANE ( 'NONE',  #46633 ) ;
#2075=ORIENTED_EDGE ( 'NONE', *, *, #7715, .F. ) ;
#2078=STYLED_ITEM ( 'NONE', ( #51484 ), #2369 ) ;
#2092=ORIENTED_EDGE ( 'NONE', *, *, #21148, .F. ) ;
#2093=EDGE_CURVE ( 'NONE', #37313, #33085, #526, .T. ) ;
#2095=CARTESIAN_POINT ( 'NONE',  ( -330.4913330509368166, -71.49045607248213230, 27.86139516340826461 ) ) ;
#2104=AXIS2_PLACEMENT_3D ( 'NONE', #5999, #22023, #30171 ) ;
#2111=VECTOR ( 'NONE', #28589, 1000.000000000000000 ) ;
#2113=VECTOR ( 'NONE', #18607, 1000.000000000000000 ) ;
#2115=LINE ( 'NONE', #17402, #1970 ) ;
#2119=EDGE_LOOP ( 'NONE', ( #36419, #24935 ) ) ;
#2120=PLANE ( 'NONE',  #5513 ) ;
#2121=DIRECTION ( 'NONE',  ( 0.000000000000000000, 3.491481338843133355E-15, 1.000000000000000000 ) ) ;
#2133=CARTESIAN_POINT ( 'NONE',  ( -336.3521761649654422, -66.60506506233235768, -15.70448169564047092 ) ) ;
#2143=EDGE_CURVE ( 'NONE', #31995, #28202, #33114, .T. ) ;
#2145=EDGE_CURVE ( 'NONE', #34105, #6023, #6050, .T. ) ;
#2150=PLANE ( 'NONE',  #41044 ) ;
#2154=ORIENTED_EDGE ( 'NONE', *, *, #14509, .T. ) ;
#2155=EDGE_CURVE ( 'NONE', #39056, #30801, #46817, .T. ) ;
#2157=EDGE_CURVE ( 'NONE', #34413, #28554, #5812, .T. ) ;
#2159=DIRECTION ( 'NONE',  ( -1.000000000000000000, 0.000000000000000000, 0.000000000000000000 ) ) ;
#2161=CARTESIAN_POINT ( 'NONE',  ( -330.4913330509368166, -63.50208336950359467, -0.4999999999999549249 ) ) ;
#2162=ORIENTED_EDGE ( 'NONE', *, *, #16135, .T. ) ;
#2163=CARTESIAN_POINT ( 'NONE',  ( -339.1964088526558498, -66.33409060400650503, 14.60509510167813474 ) ) ;
#2164=ADVANCED_FACE ( 'NONE', ( #21825 ), #9473, .F. ) ;
#2165=AXIS2_PLACEMENT_3D ( 'NONE', #19048, #2497, #27168 ) ;
#2167=PLANE ( 'NONE',  #13173 ) ;
#2168=ADVANCED_FACE ( 'NONE', ( #26260 ), #45735, .F. ) ;
#2171=VERTEX_POINT ( 'NONE', #49677 ) ;
#2179=FACE_BOUND ( 'NONE', #2531, .T. ) ;
#2185=VECTOR ( 'NONE', #26743, 1000.000000000000000 ) ;
#2187=DIRECTION ( 'NONE',  ( 1.000000000000000000, 0.000000000000000000, -0.000000000000000000 ) ) ;
#2188=ORIENTED_EDGE ( 'NONE', *, *, #47808, .F. ) ;
#2191=LINE ( 'NONE', #19002, #2203 ) ;
#2192=DIRECTION ( 'NONE',  ( 0.000000000000000000, 0.000000000000000000, 1.000000000000000000 ) ) ;
#2196=DIRECTION ( 'NONE',  ( -0.000000000000000000, -0.2393156642875516049, 0.9709418174260534551 ) ) ;
#2199=CARTESIAN_POINT ( 'NONE',  ( -180.0000000000000568, -108.2550424820446295, 0.000000000000000000 ) ) ;
#2200=CARTESIAN_POINT ( 'NONE',  ( -339.1964088526558498, -68.51134412508183402, -21.38919645685240312 ) ) ;
#2201=DIRECTION ( 'NONE',  ( 1.000000000000000000, 0.000000000000000000, 0.000000000000000000 ) ) ;
#2202=ORIENTED_EDGE ( 'NONE', *, *, #39930, .F. ) ;
#2203=VECTOR ( 'NONE', #18484, 1000.000000000000000 ) ;
#2210=CARTESIAN_POINT ( 'NONE',  ( -336.3521761649653854, -69.63373947859463442, 26.42775013958025454 ) ) ;
#2211=ORIENTED_EDGE ( 'NONE', *, *, #30393, .T. ) ;
#2216=EDGE_CURVE ( 'NONE', #24027, #4633, #37320, .T. ) ;
#2221=DIRECTION ( 'NONE',  ( -8.718379230999705894E-17, 0.1205366802553233113, 0.9927088740980539727 ) ) ;
#2225=VERTEX_POINT ( 'NONE', #45231 ) ;
#2226=LINE ( 'NONE', #18267, #50162 ) ;
#2229=VECTOR ( 'NONE', #51703, 999.9999999999998863 ) ;
#2231=EDGE_CURVE ( 'NONE', #3375, #11938, #14976, .T. ) ;
#2232=CARTESIAN_POINT ( 'NONE',  ( -336.3521761649654422, -123.5000000000000284, 0.000000000000000000 ) ) ;
#2233=CARTESIAN_POINT ( 'NONE',  ( -330.4913330509368166, -171.7720157143599238, 33.92731199008539278 ) ) ;
#2238=EDGE_CURVE ( 'NONE', #49593, #17654, #22597, .T. ) ;
#2240=DIRECTION ( 'NONE',  ( -0.000000000000000000, 0.8854560256532141294, 0.4647231720437604574 ) ) ;
#2241=VERTEX_POINT ( 'NONE', #14708 ) ;
#2245=VECTOR ( 'NONE', #49696, 1000.000000000000000 ) ;
#2250=CARTESIAN_POINT ( 'NONE',  ( -330.4913330509368166, -74.65991953890876687, -33.10432812419148263 ) ) ;
#2252=ORIENTED_EDGE ( 'NONE', *, *, #23754, .F. ) ;
#2255=ORIENTED_EDGE ( 'NONE', *, *, #31948, .T. ) ;
#2260=DIRECTION ( 'NONE',  ( 1.000000000000000000, -0.000000000000000000, -0.000000000000000000 ) ) ;
#2265=CARTESIAN_POINT ( 'NONE',  ( -336.3521761649654422, -65.12692710742291524, -8.732051761643681687 ) ) ;
#2270=VECTOR ( 'NONE', #4526, 1000.000000000000000 ) ;
#2271=LINE ( 'NONE', #34324, #9966 ) ;
#2273=VECTOR ( 'NONE', #50562, 999.9999999999998863 ) ;
#2278=VECTOR ( 'NONE', #33516, 1000.000000000000114 ) ;
#2283=CARTESIAN_POINT ( 'NONE',  ( -339.1964088526558498, -181.8741440471348483, -13.87297036558331520 ) ) ;
#2286=ADVANCED_FACE ( 'NONE', ( #31495 ), #6574, .F. ) ;
#2289=CARTESIAN_POINT ( 'NONE',  ( -336.3521761649654422, -126.1322888500942270, -59.00000000000001421 ) ) ;
#2291=EDGE_LOOP ( 'NONE', ( #40818, #35669, #44827, #5786 ) ) ;
#2294=VECTOR ( 'NONE', #6582, 1000.000000000000114 ) ;
#2297=LINE ( 'NONE', #45937, #22604 ) ;
#2300=ORIENTED_EDGE ( 'NONE', *, *, #37534, .T. ) ;
#2301=FACE_OUTER_BOUND ( 'NONE', #27373, .T. ) ;
#2302=ORIENTED_EDGE ( 'NONE', *, *, #8732, .T. ) ;
#2304=ORIENTED_EDGE ( 'NONE', *, *, #9191, .T. ) ;
#2308=FACE_OUTER_BOUND ( 'NONE', #28245, .T. ) ;
#2315=CARTESIAN_POINT ( 'NONE',  ( -336.3521761649654422, -182.5000000000000568, 2.632288850093980503 ) ) ;
#2326=DIRECTION ( 'NONE',  ( 1.000000000000000000, -0.000000000000000000, -0.000000000000000000 ) ) ;
#2329=CARTESIAN_POINT ( 'NONE',  ( -330.4913330509368166, -175.5095439275173419, 27.86139516340933042 ) ) ;
#2330=CARTESIAN_POINT ( 'NONE',  ( -336.3521761649654422, -182.5000000000000568, 1.632288850093980725 ) ) ;
#2331=CARTESIAN_POINT ( 'NONE',  ( -336.3521761649654422, -65.58448481710581746, 11.56382487286456140 ) ) ;
#2333=AXIS2_PLACEMENT_3D ( 'NONE', #48336, #4193, #32029 ) ;
#2335=LINE ( 'NONE', #18363, #24656 ) ;
#2346=CARTESIAN_POINT ( 'NONE',  ( 0.000000000000000000, -79.33786585790510060, -39.12423683620700388 ) ) ;
#2347=VECTOR ( 'NONE', #35707, 1000.000000000000000 ) ;
#2349=DIRECTION ( 'NONE',  ( -0.000000000000000000, -0.7485107481711046340, -0.6631226582407911962 ) ) ;
#2351=DIRECTION ( 'NONE',  ( -0.000000000000000000, 0.000000000000000000, -1.000000000000000000 ) ) ;
#2352=EDGE_CURVE ( 'NONE', #2690, #11626, #43071, .T. ) ;
#2353=DIRECTION ( 'NONE',  ( -1.000000000000000000, -4.850383327711956209E-15, -9.241633304753555563E-15 ) ) ;
#2354=ORIENTED_EDGE ( 'NONE', *, *, #19015, .F. ) ;
#2355=DIRECTION ( 'NONE',  ( 0.000000000000000000, 0.7485107481711046340, 0.6631226582407911962 ) ) ;
#2357=DIRECTION ( 'NONE',  ( 0.000000000000000000, -0.5680647467311540355, 0.8229838658936575735 ) ) ;
#2362=CARTESIAN_POINT ( 'NONE',  ( -332.3517673607765914, -182.5000000000000568, 1.632288850093980725 ) ) ;
#2364=ORIENTED_EDGE ( 'NONE', *, *, #28169, .F. ) ;
#2369=MANIFOLD_SOLID_BREP ( 'CirPattern2', #43848 ) ;
#2373=ORIENTED_EDGE ( 'NONE', *, *, #28707, .F. ) ;
#2375=DIRECTION ( 'NONE',  ( 0.000000000000000000, 0.3546048870425267951, -0.9350162426854181641 ) ) ;
#2379=DIRECTION ( 'NONE',  ( -0.000000000000000000, 0.8854560256532093554, -0.4647231720437695057 ) ) ;
#2382=FACE_OUTER_BOUND ( 'NONE', #48470, .T. ) ;
#2386=CARTESIAN_POINT ( 'NONE',  ( -332.3517673607765914, -142.8954717479169574, 55.74477592174805096 ) ) ;
#2387=FACE_OUTER_BOUND ( 'NONE', #33565, .T. ) ;
#2399=CARTESIAN_POINT ( 'NONE',  ( -339.1964088526558498, -172.3400804610910200, 33.10432812419180948 ) ) ;
#2400=CARTESIAN_POINT ( 'NONE',  ( -330.4913330509368166, -96.06030588028409056, 53.35787839313353231 ) ) ;
#2401=EDGE_CURVE ( 'NONE', #5376, #7178, #22844, .T. ) ;
#2406=ADVANCED_FACE ( 'NONE', ( #24150 ), #28328, .F. ) ;
#2408=CARTESIAN_POINT ( 'NONE',  ( -339.1964088526558498, -123.5000000000000284, 0.000000000000000000 ) ) ;
#2411=EDGE_CURVE ( 'NONE', #44450, #14966, #12990, .T. ) ;
#2412=DIRECTION ( 'NONE',  ( -0.000000000000000000, 0.9709418174260519008, -0.2393156642875582940 ) ) ;
#2413=ADVANCED_FACE ( 'NONE', ( #20189 ), #44382, .F. ) ;
#2415=ORIENTED_EDGE ( 'NONE', *, *, #3504, .T. ) ;
#2416=VECTOR ( 'NONE', #22994, 1000.000000000000000 ) ;
#2417=ORIENTED_EDGE ( 'NONE', *, *, #27189, .T. ) ;
#2419=VECTOR ( 'NONE', #49094, 1000.000000000000000 ) ;
#2423=DIRECTION ( 'NONE',  ( 0.000000000000000000, 0.000000000000000000, 1.000000000000000000 ) ) ;
#2434=ORIENTED_EDGE ( 'NONE', *, *, #47338, .T. ) ;
#2435=PLANE ( 'NONE',  #3718 ) ;
#2438=LINE ( 'NONE', #50784, #43914 ) ;
#2444=ORIENTED_EDGE ( 'NONE', *, *, #2059, .F. ) ;
#2447=ORIENTED_EDGE ( 'NONE', *, *, #9720, .T. ) ;
#2448=FACE_BOUND ( 'NONE', #44907, .T. ) ;
#2452=EDGE_LOOP ( 'NONE', ( #5930, #14011, #3673, #38104 ) ) ;
#2453=VECTOR ( 'NONE', #3108, 1000.000000000000000 ) ;
#2455=CARTESIAN_POINT ( 'NONE',  ( -305.0000000000000568, -177.7994952405510389, -25.52576769896207409 ) ) ;
#2458=LINE ( 'NONE', #26361, #47528 ) ;
#2461=DIRECTION ( 'NONE',  ( -0.000000000000000000, 0.8229838658936556861, -0.5680647467311569221 ) ) ;
#2468=CARTESIAN_POINT ( 'NONE',  ( -365.0000000000001137, -78.50000000000002842, 10.00000000000000711 ) ) ;
#2469=EDGE_LOOP ( 'NONE', ( #25496, #25820, #13141, #4705 ) ) ;
#2470=ORIENTED_EDGE ( 'NONE', *, *, #37212, .F. ) ;
#2473=ADVANCED_FACE ( 'NONE', ( #8618 ), #40662, .F. ) ;
#2475=LINE ( 'NONE', #10869, #39680 ) ;
#2484=CARTESIAN_POINT ( 'NONE',  ( -332.3517673607765914, -153.2494431741581025, -51.01861988938816950 ) ) ;
#2491=DIRECTION ( 'NONE',  ( -1.000000000000000000, 0.000000000000000000, 0.000000000000000000 ) ) ;
#2495=VERTEX_POINT ( 'NONE', #7839 ) ;
#2496=ORIENTED_EDGE ( 'NONE', *, *, #2352, .F. ) ;
#2497=DIRECTION ( 'NONE',  ( 1.000000000000000000, 0.000000000000000000, -0.000000000000000000 ) ) ;
#2500=DIRECTION ( 'NONE',  ( -1.000000000000000000, -0.000000000000000000, 0.000000000000000000 ) ) ;
#2503=DIRECTION ( 'NONE',  ( -1.000000000000000000, 0.000000000000000000, 0.000000000000000000 ) ) ;
#2507=VERTEX_POINT ( 'NONE', #4961 ) ;
#2514=PLANE ( 'NONE',  #44018 ) ;
#2518=ADVANCED_FACE ( 'NONE', ( #33831 ), #25949, .F. ) ;
#2519=CARTESIAN_POINT ( 'NONE',  ( -336.3521761649654422, -181.1761995186066088, -12.53476669029101842 ) ) ;
#2525=ORIENTED_EDGE ( 'NONE', *, *, #11768, .T. ) ;
#2527=EDGE_CURVE ( 'NONE', #44388, #35955, #51650, .T. ) ;
#2530=CARTESIAN_POINT ( 'NONE',  ( -339.1964088526558498, -123.5000000000000284, 0.000000000000000000 ) ) ;
#2531=EDGE_LOOP ( 'NONE', ( #1201, #45244, #13783, #20748 ) ) ;
#2534=PLANE ( 'NONE',  #11165 ) ;
#2537=ADVANCED_FACE ( 'NONE', ( #49871 ), #18068, .F. ) ;
#2543=VECTOR ( 'NONE', #46906, 1000.000000000000000 ) ;
#2549=DIRECTION ( 'NONE',  ( 0.000000000000000000, 0.5680647467311510379, -0.8229838658936596829 ) ) ;
#2556=CARTESIAN_POINT ( 'NONE',  ( -330.4913330509368166, -116.8846903019842927, 58.63009191191280678 ) ) ;
#2562=LINE ( 'NONE', #50400, #3133 ) ;
#2573=LINE ( 'NONE', #2329, #4743 ) ;
#2574=DIRECTION ( 'NONE',  ( -0.000000000000000000, -1.000000000000000000, -0.000000000000000000 ) ) ;
#2576=EDGE_CURVE ( 'NONE', #32690, #4224, #9411, .T. ) ;
#2577=LINE ( 'NONE', #30677, #17965 ) ;
#2578=DIRECTION ( 'NONE',  ( 0.000000000000000000, 0.9350162426854107256, -0.3546048870425463906 ) ) ;
#2582=VECTOR ( 'NONE', #32320, 1000.000000000000000 ) ;
#2585=EDGE_CURVE ( 'NONE', #48198, #41229, #13603, .T. ) ;
#2586=FACE_OUTER_BOUND ( 'NONE', #750, .T. ) ;
#2588=CARTESIAN_POINT ( 'NONE',  ( -339.1964088526558498, -175.9742670995610752, 26.97593913775620678 ) ) ;
#2594=AXIS2_PLACEMENT_3D ( 'NONE', #32463, #36929, #16183 ) ;
#2597=LINE ( 'NONE', #42796, #48093 ) ;
#2599=LINE ( 'NONE', #25996, #3345 ) ;
#2601=EDGE_CURVE ( 'NONE', #25289, #18828, #36550, .T. ) ;
#2602=CARTESIAN_POINT ( 'NONE',  ( -336.3521761649654422, -168.7445418633863596, -37.90245108779149064 ) ) ;
#2603=ORIENTED_EDGE ( 'NONE', *, *, #4774, .T. ) ;
#2604=DIRECTION ( 'NONE',  ( -1.000000000000000000, 0.000000000000000000, 0.000000000000000000 ) ) ;
#2615=LINE ( 'NONE', #18652, #31489 ) ;
#2622=VERTEX_POINT ( 'NONE', #10697 ) ;
#2629=VERTEX_POINT ( 'NONE', #26977 ) ;
#2633=LINE ( 'NONE', #10265, #5839 ) ;
#2635=VERTEX_POINT ( 'NONE', #26455 ) ;
#2639=CARTESIAN_POINT ( 'NONE',  ( -336.3521761649654422, -178.6135371030394481, 23.71704087764532431 ) ) ;
#2648=VECTOR ( 'NONE', #51030, 1000.000000000000114 ) ;
#2657=DIRECTION ( 'NONE',  ( 0.000000000000000000, 1.000000000000000000, -3.491481338843133355E-15 ) ) ;
#2662=CARTESIAN_POINT ( 'NONE',  ( -330.4913330509368166, -131.1080185721124849, 58.50955523165764305 ) ) ;
#2670=DIRECTION ( 'NONE',  ( 1.000000000000000000, 0.000000000000000000, -0.000000000000000000 ) ) ;
#2672=LINE ( 'NONE', #10058, #24754 ) ;
#2676=VERTEX_POINT ( 'NONE', #27498 ) ;
#2682=VECTOR ( 'NONE', #38905, 1000.000000000000000 ) ;
#2685=CARTESIAN_POINT ( 'NONE',  ( -305.0000000000000568, -123.5000000000000284, 15.24495751795539000 ) ) ;
#2688=DIRECTION ( 'NONE',  ( -0.000000000000000000, -0.3546048870425363986, -0.9350162426854146114 ) ) ;
#2689=DIRECTION ( 'NONE',  ( 0.000000000000000000, 0.3546048870425300148, -0.9350162426854169428 ) ) ;
#2690=VERTEX_POINT ( 'NONE', #38557 ) ;
#2692=FACE_BOUND ( 'NONE', #13303, .T. ) ;
#2693=VECTOR ( 'NONE', #29787, 1000.000000000000000 ) ;
#2699=EDGE_CURVE ( 'NONE', #32359, #21474, #10428, .T. ) ;
#2702=CARTESIAN_POINT ( 'NONE',  ( -332.3517673607765914, -104.1045282520827300, -55.74477592174792306 ) ) ;
#2703=ORIENTED_EDGE ( 'NONE', *, *, #43271, .F. ) ;
#2706=DIRECTION ( 'NONE',  ( -0.000000000000000000, -0.9709418174260502354, 0.2393156642875652051 ) ) ;
#2714=ORIENTED_EDGE ( 'NONE', *, *, #182, .F. ) ;
#2715=AXIS2_PLACEMENT_3D ( 'NONE', #26473, #6527, #22557 ) ;
#2717=CARTESIAN_POINT ( 'NONE',  ( -330.4913330509368166, -130.1153096980145563, 58.63009191191294178 ) ) ;
#2719=LINE ( 'NONE', #15092, #1940 ) ;
#2722=ORIENTED_EDGE ( 'NONE', *, *, #49646, .F. ) ;
#2727=ORIENTED_EDGE ( 'NONE', *, *, #17980, .F. ) ;
#2730=CIRCLE ( 'NONE', #21197, 60.00000000000000000 ) ;
#2735=VECTOR ( 'NONE', #3422, 1000.000000000000000 ) ;
#2737=LINE ( 'NONE', #18274, #6269 ) ;
#2743=CARTESIAN_POINT ( 'NONE',  ( -336.3521761649653854, -75.06648993880729392, -35.41461708323759439 ) ) ;
#2746=DIRECTION ( 'NONE',  ( 0.000000000000000000, -0.2393156642875449158, 0.9709418174260553425 ) ) ;
#2747=CARTESIAN_POINT ( 'NONE',  ( -339.1964088526558498, -71.49045607248255862, -27.86139516340906397 ) ) ;
#2749=DIRECTION ( 'NONE',  ( 1.000000000000000000, 0.000000000000000000, -0.000000000000000000 ) ) ;
#2757=VECTOR ( 'NONE', #51275, 1000.000000000000114 ) ;
#2760=EDGE_CURVE ( 'NONE', #39742, #26732, #3330, .T. ) ;
#2761=DIRECTION ( 'NONE',  ( 0.000000000000000000, 1.000000000000000000, -3.491481338843133355E-15 ) ) ;
#2767=CARTESIAN_POINT ( 'NONE',  ( -336.3521761649654422, -132.2320517616439020, -58.37307289257706344 ) ) ;
#2770=ORIENTED_EDGE ( 'NONE', *, *, #43974, .T. ) ;
#2771=VECTOR ( 'NONE', #46047, 1000.000000000000000 ) ;
#2774=ORIENTED_EDGE ( 'NONE', *, *, #45659, .F. ) ;
#2779=CARTESIAN_POINT ( 'NONE',  ( -332.3517673607765914, -181.4155151828941825, -11.56382487286496463 ) ) ;
#2782=FACE_OUTER_BOUND ( 'NONE', #43636, .T. ) ;
#2784=CARTESIAN_POINT ( 'NONE',  ( -305.0000000000000568, -138.3439121830091665, 58.13482838284733845 ) ) ;
#2785=VECTOR ( 'NONE', #43097, 999.9999999999998863 ) ;
#2787=LINE ( 'NONE', #42474, #39957 ) ;
#2788=ORIENTED_EDGE ( 'NONE', *, *, #21136, .T. ) ;
#2791=ORIENTED_EDGE ( 'NONE', *, *, #22489, .F. ) ;
#2792=DIRECTION ( 'NONE',  ( 1.000000000000000000, 0.000000000000000000, -0.000000000000000000 ) ) ;
#2793=CARTESIAN_POINT ( 'NONE',  ( -330.4913330509368166, -71.02573290043841325, 26.97593913775512320 ) ) ;
#2799=EDGE_CURVE ( 'NONE', #6394, #32153, #22260, .T. ) ;
#2801=VECTOR ( 'NONE', #39200, 1000.000000000000000 ) ;
#2806=ORIENTED_EDGE ( 'NONE', *, *, #30325, .T. ) ;
#2807=CIRCLE ( 'NONE', #7828, 60.00000000000000000 ) ;
#2811=ADVANCED_FACE ( 'NONE', ( #7537 ), #11726, .T. ) ;
#2813=PLANE ( 'NONE',  #4386 ) ;
#2817=CARTESIAN_POINT ( 'NONE',  ( -332.3517673607765914, -81.78065195202965754, 43.12187378178632002 ) ) ;
#2820=EDGE_LOOP ( 'NONE', ( #11563, #23286, #40592, #821 ) ) ;
#2823=ADVANCED_FACE ( 'NONE', ( #3582 ), #36685, .F. ) ;
#2831=DIRECTION ( 'NONE',  ( 0.000000000000000000, 0.000000000000000000, 1.000000000000000000 ) ) ;
#2832=CARTESIAN_POINT ( 'NONE',  ( -339.1964088526558498, -123.5000000000000284, 0.000000000000000000 ) ) ;
#2836=VECTOR ( 'NONE', #47077, 1000.000000000000000 ) ;
#2841=ORIENTED_EDGE ( 'NONE', *, *, #31650, .F. ) ;
#2848=DIRECTION ( 'NONE',  ( -1.000000000000000000, 0.000000000000000000, 0.000000000000000000 ) ) ;
#2849=CARTESIAN_POINT ( 'NONE',  ( -336.3521761649654422, -141.9604555052315220, 56.09938080879057765 ) ) ;
#2853=DIRECTION ( 'NONE',  ( -1.000000000000000000, 0.000000000000000000, 0.000000000000000000 ) ) ;
#2856=VECTOR ( 'NONE', #32400, 1000.000000000000000 ) ;
#2859=ADVANCED_FACE ( 'NONE', ( #16198 ), #32214, .F. ) ;
#2860=EDGE_CURVE ( 'NONE', #33085, #41706, #44322, .T. ) ;
#2863=CARTESIAN_POINT ( 'NONE',  ( -330.4913330509368166, -64.99044476834247064, -7.608018572113060429 ) ) ;
#2867=FILL_AREA_STYLE ('',( #38863 ) ) ;
#2876=CARTESIAN_POINT ( 'NONE',  ( -339.1964088526558498, -79.66942718702493664, 39.49849221029193558 ) ) ;
#2877=FACE_OUTER_BOUND ( 'NONE', #9899, .T. ) ;
#2879=AXIS2_PLACEMENT_3D ( 'NONE', #4892, #20919, #8809 ) ;
#2880=ORIENTED_EDGE ( 'NONE', *, *, #42682, .T. ) ;
#2881=LINE ( 'NONE', #18913, #13957 ) ;
#2884=PLANE ( 'NONE',  #25669 ) ;
#2885=ADVANCED_FACE ( 'NONE', ( #5413 ), #49565, .F. ) ;
#2888=PLANE ( 'NONE',  #9864 ) ;
#2891=PLANE ( 'NONE',  #28210 ) ;
#2899=DIRECTION ( 'NONE',  ( -0.000000000000000000, 1.047444401652940007E-14, 1.000000000000000000 ) ) ;
#2902=CARTESIAN_POINT ( 'NONE',  ( -339.1964088526558498, -95.63860483659040312, 52.00954392751717847 ) ) ;
#2906=EDGE_LOOP ( 'NONE', ( #26695, #12208, #32985, #5534, #29970 ) ) ;
#2907=VECTOR ( 'NONE', #5897, 1000.000000000000000 ) ;
#2911=CARTESIAN_POINT ( 'NONE',  ( -339.1964088526558498, -103.0458197858333165, -55.34326076196084188 ) ) ;
#2918=ORIENTED_EDGE ( 'NONE', *, *, #27844, .F. ) ;
#2920=EDGE_LOOP ( 'NONE', ( #46963, #47101, #2188, #41222 ) ) ;
#2921=DIRECTION ( 'NONE',  ( 1.000000000000000000, 0.000000000000000000, 0.000000000000000000 ) ) ;
#2922=EDGE_CURVE ( 'NONE', #24837, #50461, #41647, .T. ) ;
#2925=VERTEX_POINT ( 'NONE', #37971 ) ;
#2927=DIRECTION ( 'NONE',  ( -0.000000000000000000, 0.9709418174260492362, -0.2393156642875685636 ) ) ;
#2930=ORIENTED_EDGE ( 'NONE', *, *, #39774, .F. ) ;
#2932=AXIS2_PLACEMENT_3D ( 'NONE', #1000, #49620, #17055 ) ;
#2942=ORIENTED_EDGE ( 'NONE', *, *, #20563, .F. ) ;
#2945=ORIENTED_EDGE ( 'NONE', *, *, #37713, .F. ) ;
#2951=ORIENTED_EDGE ( 'NONE', *, *, #48129, .T. ) ;
#2952=FACE_BOUND ( 'NONE', #22178, .T. ) ;
#2953=AXIS2_PLACEMENT_3D ( 'NONE', #41258, #5284, #5543 ) ;
#2958=LINE ( 'NONE', #18994, #12322 ) ;
#2959=VERTEX_POINT ( 'NONE', #1183 ) ;
#2960=PLANE ( 'NONE',  #14770 ) ;
#2962=ORIENTED_EDGE ( 'NONE', *, *, #49101, .T. ) ;
#2964=PLANE ( 'NONE',  #28054 ) ;
#2968=VECTOR ( 'NONE', #11030, 1000.000000000000000 ) ;
#2971=DIRECTION ( 'NONE',  ( 0.000000000000000000, 0.2393156642875652051, 0.9709418174260502354 ) ) ;
#2972=VERTEX_POINT ( 'NONE', #1974 ) ;
#2978=ORIENTED_EDGE ( 'NONE', *, *, #37892, .F. ) ;
#2981=VECTOR ( 'NONE', #18582, 1000.000000000000114 ) ;
#2983=CARTESIAN_POINT ( 'NONE',  ( -332.3517673607765914, -64.50000000000000000, -2.632288850093980503 ) ) ;
#2989=LINE ( 'NONE', #43463, #43400 ) ;
#2990=ORIENTED_EDGE ( 'NONE', *, *, #34656, .F. ) ;
#2992=ORIENTED_EDGE ( 'NONE', *, *, #24458, .F. ) ;
#2995=CARTESIAN_POINT ( 'NONE',  ( -339.1964088526558498, -156.6043281241909426, 48.84008046109164525 ) ) ;
#3000=ADVANCED_FACE ( 'NONE', ( #37720 ), #5154, .F. ) ;
#3001=CARTESIAN_POINT ( 'NONE',  ( -339.1964088526558498, -79.00630452878414189, 38.74998146212082162 ) ) ;
#3004=AXIS2_PLACEMENT_3D ( 'NONE', #32821, #20744, #45447 ) ;
#3007=ADVANCED_FACE ( 'NONE', ( #13808 ), #18015, .F. ) ;
#3008=DIRECTION ( 'NONE',  ( -0.000000000000000000, 0.4647231720437664526, -0.8854560256532110207 ) ) ;
#3010=VECTOR ( 'NONE', #24179, 1000.000000000000000 ) ;
#3015=CARTESIAN_POINT ( 'NONE',  ( -339.1964088526558498, -144.8891964568517778, 54.98865587491845730 ) ) ;
#3020=VERTEX_POINT ( 'NONE', #29824 ) ;
#3027=LINE ( 'NONE', #42189, #16908 ) ;
#3033=EDGE_CURVE ( 'NONE', #43448, #13360, #9867, .T. ) ;
#3037=EDGE_CURVE ( 'NONE', #14966, #49846, #4895, .T. ) ;
#3041=VERTEX_POINT ( 'NONE', #7658 ) ;
#3043=DIRECTION ( 'NONE',  ( -0.000000000000000000, -0.4647231720437604574, 0.8854560256532141294 ) ) ;
#3045=CARTESIAN_POINT ( 'NONE',  ( -332.3517673607765914, -107.5615171630107056, 57.84431488793861575 ) ) ;
#3047=EDGE_CURVE ( 'NONE', #43162, #44157, #43415, .T. ) ;
#3048=CARTESIAN_POINT ( 'NONE',  ( -305.0000000000000568, -140.4009141470556870, -57.57047073799078873 ) ) ;
#3049=LINE ( 'NONE', #34835, #29053 ) ;
#3056=VECTOR ( 'NONE', #23259, 1000.000000000000000 ) ;
#3066=ORIENTED_EDGE ( 'NONE', *, *, #38478, .F. ) ;
#3071=AXIS2_PLACEMENT_3D ( 'NONE', #45732, #46260, #18129 ) ;
#3084=CARTESIAN_POINT ( 'NONE',  ( -339.1964088526558498, -137.1341532842523065, 57.40522506028101901 ) ) ;
#3085=ORIENTED_EDGE ( 'NONE', *, *, #25013, .F. ) ;
#3086=CARTESIAN_POINT ( 'NONE',  ( -332.3517673607765914, -94.63601285149479736, 51.48334306143172512 ) ) ;
#3089=DIRECTION ( 'NONE',  ( 0.000000000000000000, 0.2393156642875449158, -0.9709418174260553425 ) ) ;
#3091=ORIENTED_EDGE ( 'NONE', *, *, #39404, .T. ) ;
#3094=PLANE ( 'NONE',  #22383 ) ;
#3095=ORIENTED_EDGE ( 'NONE', *, *, #6975, .T. ) ;
#3102=EDGE_CURVE ( 'NONE', #15715, #19072, #27102, .T. ) ;
#3106=ORIENTED_EDGE ( 'NONE', *, *, #33863, .F. ) ;
#3107=VECTOR ( 'NONE', #25503, 1000.000000000000000 ) ;
#3108=DIRECTION ( 'NONE',  ( -0.000000000000000000, 0.4647231720437664526, -0.8854560256532110207 ) ) ;
#3115=EDGE_CURVE ( 'NONE', #7946, #37313, #3452, .T. ) ;
#3118=AXIS2_PLACEMENT_3D ( 'NONE', #4623, #48537, #24855 ) ;
#3120=ADVANCED_FACE ( 'NONE', ( #15052 ), #51302, .F. ) ;
#3125=CARTESIAN_POINT ( 'NONE',  ( -330.4913330509368166, -150.4759391377553186, 52.47426709956150859 ) ) ;
#3131=VECTOR ( 'NONE', #15151, 1000.000000000000000 ) ;
#3133=VECTOR ( 'NONE', #14392, 1000.000000000000000 ) ;
#3140=VERTEX_POINT ( 'NONE', #19736 ) ;
#3141=LINE ( 'NONE', #2095, #48429 ) ;
#3143=ORIENTED_EDGE ( 'NONE', *, *, #36585, .F. ) ;
#3148=CARTESIAN_POINT ( 'NONE',  ( -336.3521761649653854, -73.21199843436539823, 32.72792230702599170 ) ) ;
#3153=DIRECTION ( 'NONE',  ( 1.000000000000000000, 0.000000000000000000, -0.000000000000000000 ) ) ;
#3154=CARTESIAN_POINT ( 'NONE',  ( -332.3517673607765914, -107.7955183043589500, 56.89493493766750731 ) ) ;
#3155=VERTEX_POINT ( 'NONE', #10122 ) ;
#3161=ORIENTED_EDGE ( 'NONE', *, *, #35392, .F. ) ;
#3165=CARTESIAN_POINT ( 'NONE',  ( -332.3517673607765914, -104.7054247829104270, -56.98038208374144631 ) ) ;
#3171=CARTESIAN_POINT ( 'NONE',  ( -336.3521761649654422, -152.3639871485048900, -51.48334306143194539 ) ) ;
#3173=EDGE_CURVE ( 'NONE', #28688, #50802, #8052, .T. ) ;
#3175=EDGE_CURVE ( 'NONE', #22773, #77, #32382, .T. ) ;
#3177=CARTESIAN_POINT ( 'NONE',  ( -336.3521761649654422, -121.8677111499054320, 59.00000000000001421 ) ) ;
#3181=DIRECTION ( 'NONE',  ( 0.000000000000000000, 0.8229838658936556861, -0.5680647467311569221 ) ) ;
#3182=AXIS2_PLACEMENT_3D ( 'NONE', #14593, #2749, #7219 ) ;
#3184=EDGE_CURVE ( 'NONE', #13909, #51040, #17118, .T. ) ;
#3186=EDGE_CURVE ( 'NONE', #41791, #50590, #40225, .T. ) ;
#3189=ORIENTED_EDGE ( 'NONE', *, *, #22689, .F. ) ;
#3190=EDGE_CURVE ( 'NONE', #39518, #23810, #284, .T. ) ;
#3192=CARTESIAN_POINT ( 'NONE',  ( -332.3517673607765914, -119.0014323656137947, -58.88711093124865670 ) ) ;
#3197=DIRECTION ( 'NONE',  ( -1.000000000000000000, 0.000000000000000000, 0.000000000000000000 ) ) ;
#3198=PLANE ( 'NONE',  #46230 ) ;
#3199=( GEOMETRIC_REPRESENTATION_CONTEXT ( 3 ) GLOBAL_UNCERTAINTY_ASSIGNED_CONTEXT ( ( #15360 ) ) GLOBAL_UNIT_ASSIGNED_CONTEXT ( ( #35774, #38, #28405 ) ) REPRESENTATION_CONTEXT ( 'NONE', 'WORKASPACE' ) );
#3200=CARTESIAN_POINT ( 'NONE',  ( -330.4913330509368166, -103.0458197858332312, -55.34326076196081345 ) ) ;
#3201=CARTESIAN_POINT ( 'NONE',  ( -339.1964088526558498, -156.6043281241916816, -48.84008046109114076 ) ) ;
#3207=AXIS2_PLACEMENT_3D ( 'NONE', #40724, #13407, #49155 ) ;
#3209=LINE ( 'NONE', #43136, #41701 ) ;
#3211=DIRECTION ( 'NONE',  ( 1.000000000000000000, 0.000000000000000000, 0.000000000000000000 ) ) ;
#3219=DIRECTION ( 'NONE',  ( -1.000000000000000000, 0.000000000000000000, 0.000000000000000000 ) ) ;
#3225=FACE_BOUND ( 'NONE', #17860, .T. ) ;
#3226=CARTESIAN_POINT ( 'NONE',  ( -339.1964088526558498, -68.15673923803898049, 20.45418021416614351 ) ) ;
#3249=CIRCLE ( 'NONE', #41845, 60.00000000000000000 ) ;
#3252=DIRECTION ( 'NONE',  ( 0.000000000000000000, -0.5680647467311596976, -0.8229838658936536877 ) ) ;
#3254=CIRCLE ( 'NONE', #29282, 15.24495751795539000 ) ;
#3257=EDGE_LOOP ( 'NONE', ( #43605, #39198, #6591, #16806 ) ) ;
#3260=CARTESIAN_POINT ( 'NONE',  ( -336.3521761649654422, -88.64083255475578937, 47.62880233550460218 ) ) ;
#3264=ADVANCED_FACE ( 'NONE', ( #21048 ), #1064, .T. ) ;
#3265=ORIENTED_EDGE ( 'NONE', *, *, #14125, .T. ) ;
#3266=VECTOR ( 'NONE', #51190, 1000.000000000000000 ) ;
#3267=DIRECTION ( 'NONE',  ( -0.000000000000000000, -0.8854560256532062468, 0.4647231720437755564 ) ) ;
#3268=CARTESIAN_POINT ( 'NONE',  ( -330.4913330509368166, -84.00150778970767362, -43.83057281297470098 ) ) ;
#3270=LINE ( 'NONE', #35561, #11916 ) ;
#3275=VERTEX_POINT ( 'NONE', #45242 ) ;
#3276=EDGE_LOOP ( 'NONE', ( #38813, #42717, #9615, #49268 ) ) ;
#3279=VECTOR ( 'NONE', #7, 1000.000000000000000 ) ;
#3283=CARTESIAN_POINT ( 'NONE',  ( -339.1964088526558498, -178.8432607619609485, -20.45418021416653076 ) ) ;
#3284=PLANE ( 'NONE',  #41894 ) ;
#3285=ORIENTED_EDGE ( 'NONE', *, *, #6170, .F. ) ;
#3286=CARTESIAN_POINT ( 'NONE',  ( -339.1964088526558498, -182.1300919119128423, 6.615309698015510165 ) ) ;
#3289=AXIS2_PLACEMENT_3D ( 'NONE', #28565, #4663, #36726 ) ;
#3291=EDGE_LOOP ( 'NONE', ( #31198, #37745, #12549, #584 ) ) ;
#3292=CARTESIAN_POINT ( 'NONE',  ( -305.0000000000000568, -96.06030588028410477, 53.35787839313353942 ) ) ;
#3293=CARTESIAN_POINT ( 'NONE',  ( -336.3521761649654422, -182.6878972721721084, 9.838334030658060669 ) ) ;
#3294=CARTESIAN_POINT ( 'NONE',  ( -339.1964088526558498, -116.8846903019842927, 58.63009191191280678 ) ) ;
#3299=EDGE_LOOP ( 'NONE', ( #46716, #35466, #17869, #16288 ) ) ;
#3302=PLANE ( 'NONE',  #30453 ) ;
#3303=ORIENTED_EDGE ( 'NONE', *, *, #47683, .T. ) ;
#3304=ORIENTED_EDGE ( 'NONE', *, *, #26166, .T. ) ;
#3306=PLANE ( 'NONE',  #9209 ) ;
#3307=ORIENTED_EDGE ( 'NONE', *, *, #46155, .T. ) ;
#3308=VECTOR ( 'NONE', #30906, 1000.000000000000000 ) ;
#3310=DIRECTION ( 'NONE',  ( -1.000000000000000000, 9.758900497077107825E-15, -3.701062773504986041E-15 ) ) ;
#3311=ADVANCED_FACE ( 'NONE', ( #34170 ), #29699, .F. ) ;
#3315=DIRECTION ( 'NONE',  ( -0.000000000000000000, -0.4647231720437631775, 0.8854560256532126861 ) ) ;
#3319=ORIENTED_EDGE ( 'NONE', *, *, #29800, .T. ) ;
#3320=FACE_OUTER_BOUND ( 'NONE', #40402, .T. ) ;
#3324=DIRECTION ( 'NONE',  ( -1.000000000000000000, 0.000000000000000000, 0.000000000000000000 ) ) ;
#3328=CARTESIAN_POINT ( 'NONE',  ( -339.1964088526558498, -68.15673923803898049, 20.45418021416614351 ) ) ;
#3330=LINE ( 'NONE', #19362, #48305 ) ;
#3341=EDGE_CURVE ( 'NONE', #49982, #31272, #38096, .T. ) ;
#3345=VECTOR ( 'NONE', #2353, 1000.000000000000000 ) ;
#3350=DIRECTION ( 'NONE',  ( 0.000000000000000000, -9.251858538542971828E-16, -1.000000000000000000 ) ) ;
#3362=DIRECTION ( 'NONE',  ( 0.000000000000000000, -0.9350162426854132791, 0.3546048870425396182 ) ) ;
#3366=DIRECTION ( 'NONE',  ( 1.000000000000000000, 0.000000000000000000, 0.000000000000000000 ) ) ;
#3371=EDGE_LOOP ( 'NONE', ( #48236, #17245, #46757, #11428 ) ) ;
#3375=VERTEX_POINT ( 'NONE', #22334 ) ;
#3380=ORIENTED_EDGE ( 'NONE', *, *, #42330, .T. ) ;
#3381=DIRECTION ( 'NONE',  ( 0.000000000000000000, 0.1205366802553130001, -0.9927088740980551940 ) ) ;
#3383=VERTEX_POINT ( 'NONE', #1604 ) ;
#3387=EDGE_LOOP ( 'NONE', ( #6035, #27977, #39490, #33390 ) ) ;
#3388=ADVANCED_FACE ( 'NONE', ( #17640 ), #33647, .F. ) ;
#3390=CARTESIAN_POINT ( 'NONE',  ( -339.1964088526558498, -68.15673923803898049, 20.45418021416614351 ) ) ;
#3393=DIRECTION ( 'NONE',  ( 0.000000000000000000, 1.047444401652940007E-14, 1.000000000000000000 ) ) ;
#3395=AXIS2_PLACEMENT_3D ( 'NONE', #12085, #47612, #11592 ) ;
#3396=VECTOR ( 'NONE', #43940, 1000.000000000000000 ) ;
#3399=DIRECTION ( 'NONE',  ( -0.000000000000000000, 0.9350162426854146114, -0.3546048870425363986 ) ) ;
#3401=DIRECTION ( 'NONE',  ( 1.000000000000000000, 0.000000000000000000, 0.000000000000000000 ) ) ;
#3404=FACE_OUTER_BOUND ( 'NONE', #15358, .T. ) ;
#3406=EDGE_CURVE ( 'NONE', #46459, #8474, #36736, .T. ) ;
#3408=DIRECTION ( 'NONE',  ( 1.000000000000000000, 0.000000000000000000, 0.000000000000000000 ) ) ;
#3411=VERTEX_POINT ( 'NONE', #49945 ) ;
#3416=ADVANCED_FACE ( 'NONE', ( #2877 ), #34673, .F. ) ;
#3421=ORIENTED_EDGE ( 'NONE', *, *, #12545, .F. ) ;
#3422=DIRECTION ( 'NONE',  ( -0.000000000000000000, -0.4647231720437604574, 0.8854560256532141294 ) ) ;
#3426=VECTOR ( 'NONE', #34753, 999.9999999999998863 ) ;
#3427=ORIENTED_EDGE ( 'NONE', *, *, #27561, .F. ) ;
#3431=ORIENTED_EDGE ( 'NONE', *, *, #7986, .T. ) ;
#3436=CARTESIAN_POINT ( 'NONE',  ( -330.4913330509368166, -64.99044476834235695, 7.608018572112246858 ) ) ;
#3437=PLANE ( 'NONE',  #41171 ) ;
#3439=FACE_OUTER_BOUND ( 'NONE', #15433, .T. ) ;
#3447=EDGE_CURVE ( 'NONE', #978, #42791, #38875, .T. ) ;
#3451=DIRECTION ( 'NONE',  ( 0.000000000000000000, 0.000000000000000000, -1.000000000000000000 ) ) ;
#3452=LINE ( 'NONE', #47624, #35728 ) ;
#3459=EDGE_CURVE ( 'NONE', #28559, #14905, #39387, .T. ) ;
#3461=AXIS2_PLACEMENT_3D ( 'NONE', #44854, #17534, #33547 ) ;
#3464=LINE ( 'NONE', #15838, #49439 ) ;
#3465=ADVANCED_FACE ( 'NONE', ( #7851 ), #14716, .F. ) ;
#3468=ORIENTED_EDGE ( 'NONE', *, *, #40786, .F. ) ;
#3472=CARTESIAN_POINT ( 'NONE',  ( -336.3521761649654422, -64.61288906875131488, 4.498567634385603142 ) ) ;
#3474=ADVANCED_FACE ( 'NONE', ( #26791 ), #27813, .F. ) ;
#3477=LINE ( 'NONE', #31077, #20716 ) ;
#3479=EDGE_CURVE ( 'NONE', #20894, #30266, #11543, .T. ) ;
#3480=CARTESIAN_POINT ( 'NONE',  ( -339.1964088526558498, -123.5000000000000284, 0.000000000000000000 ) ) ;
#3481=VECTOR ( 'NONE', #19868, 1000.000000000000000 ) ;
#3487=LINE ( 'NONE', #35538, #45911 ) ;
#3489=CARTESIAN_POINT ( 'NONE',  ( -336.3521761649654422, -123.5000000000000284, 0.000000000000000000 ) ) ;
#3490=EDGE_LOOP ( 'NONE', ( #22008, #24921, #2727, #5005 ) ) ;
#3491=ORIENTED_EDGE ( 'NONE', *, *, #37226, .T. ) ;
#3494=CARTESIAN_POINT ( 'NONE',  ( -330.4913330509368166, -168.7406467949208491, -39.41172259083864304 ) ) ;
#3496=AXIS2_PLACEMENT_3D ( 'NONE', #50222, #31000, #46789 ) ;
#3500=ORIENTED_EDGE ( 'NONE', *, *, #50402, .F. ) ;
#3502=VECTOR ( 'NONE', #15020, 1000.000000000000000 ) ;
#3504=EDGE_CURVE ( 'NONE', #17026, #15537, #23119, .T. ) ;
#3513=EDGE_CURVE ( 'NONE', #8223, #41791, #3650, .T. ) ;
#3516=LINE ( 'NONE', #15363, #4729 ) ;
#3524=DIRECTION ( 'NONE',  ( 0.000000000000000000, 0.000000000000000000, 1.000000000000000000 ) ) ;
#3526=ORIENTED_EDGE ( 'NONE', *, *, #49473, .T. ) ;
#3527=CARTESIAN_POINT ( 'NONE',  ( -330.4913330509368166, -123.5000000000000284, 0.000000000000000000 ) ) ;
#3529=FACE_OUTER_BOUND ( 'NONE', #18600, .T. ) ;
#3530=ORIENTED_EDGE ( 'NONE', *, *, #3037, .T. ) ;
#3532=ORIENTED_EDGE ( 'NONE', *, *, #5088, .T. ) ;
#3533=CARTESIAN_POINT ( 'NONE',  ( -330.4913330509368166, -172.3400804610915031, -33.10432812419114157 ) ) ;
#3538=EDGE_CURVE ( 'NONE', #40265, #21496, #4186, .T. ) ;
#3540=DIRECTION ( 'NONE',  ( 0.000000000000000000, 0.000000000000000000, -1.000000000000000000 ) ) ;
#3545=CARTESIAN_POINT ( 'NONE',  ( -305.0000000000000568, -102.6919536717979184, -56.27632902032075890 ) ) ;
#3547=VERTEX_POINT ( 'NONE', #32552 ) ;
#3548=CARTESIAN_POINT ( 'NONE',  ( -339.1964088526558498, -131.1080185721124849, 58.50955523165764305 ) ) ;
#3550=EDGE_LOOP ( 'NONE', ( #720, #32785, #16918, #35231 ) ) ;
#3551=ORIENTED_EDGE ( 'NONE', *, *, #4791, .T. ) ;
#3552=PLANE ( 'NONE',  #34659 ) ;
#3553=VECTOR ( 'NONE', #33873, 1000.000000000000000 ) ;
#3554=AXIS2_PLACEMENT_3D ( 'NONE', #23508, #629, #4057 ) ;
#3558=ORIENTED_EDGE ( 'NONE', *, *, #26310, .F. ) ;
#3559=DIRECTION ( 'NONE',  ( -0.000000000000000000, -0.5680647467311569221, -0.8229838658936556861 ) ) ;
#3562=CARTESIAN_POINT ( 'NONE',  ( -339.1964088526558498, -143.9541802141663709, 55.34326076196097688 ) ) ;
#3563=DIRECTION ( 'NONE',  ( 1.000000000000000000, 0.000000000000000000, -0.000000000000000000 ) ) ;
#3566=EDGE_LOOP ( 'NONE', ( #46580, #2918, #43455, #41000 ) ) ;
#3567=EDGE_LOOP ( 'NONE', ( #42805, #46246, #43625, #13778 ) ) ;
#3575=VECTOR ( 'NONE', #48792, 1000.000000000000114 ) ;
#3578=EDGE_CURVE ( 'NONE', #18160, #44807, #12042, .T. ) ;
#3581=EDGE_LOOP ( 'NONE', ( #29738, #22166, #15045, #4362 ) ) ;
#3582=FACE_OUTER_BOUND ( 'NONE', #7751, .T. ) ;
#3596=DIRECTION ( 'NONE',  ( -0.000000000000000000, 0.7485107481711089639, 0.6631226582407863113 ) ) ;
#3605=ORIENTED_EDGE ( 'NONE', *, *, #18593, .F. ) ;
#3607=DIRECTION ( 'NONE',  ( 1.000000000000000000, -0.000000000000000000, 0.000000000000000000 ) ) ;
#3608=EDGE_CURVE ( 'NONE', #8376, #42588, #35046, .T. ) ;
#3614=ORIENTED_EDGE ( 'NONE', *, *, #26310, .T. ) ;
#3620=LINE ( 'NONE', #28312, #46412 ) ;
#3626=VERTEX_POINT ( 'NONE', #8892 ) ;
#3628=VECTOR ( 'NONE', #8719, 1000.000000000000000 ) ;
#3629=EDGE_LOOP ( 'NONE', ( #49421, #45910, #36646, #26374 ) ) ;
#3634=PLANE ( 'NONE',  #30093 ) ;
#3637=DIRECTION ( 'NONE',  ( 0.000000000000000000, -0.9927088740980551940, -0.1205366802553130001 ) ) ;
#3638=( NAMED_UNIT ( * ) PLANE_ANGLE_UNIT ( ) SI_UNIT ( $, .RADIAN. ) );
#3640=EDGE_CURVE ( 'NONE', #21717, #19973, #48601, .T. ) ;
#3646=ORIENTED_EDGE ( 'NONE', *, *, #45292, .T. ) ;
#3649=PLANE ( 'NONE',  #39999 ) ;
#3650=LINE ( 'NONE', #19677, #34226 ) ;
#3653=CARTESIAN_POINT ( 'NONE',  ( -336.3521761649654422, -173.5513585866778214, -31.34948880313881503 ) ) ;
#3655=DIRECTION ( 'NONE',  ( -1.000000000000000000, 0.000000000000000000, -0.000000000000000000 ) ) ;
#3657=EDGE_CURVE ( 'NONE', #16597, #12335, #31708, .T. ) ;
#3662=ADVANCED_FACE ( 'NONE', ( #12832 ), #32277, .F. ) ;
#3665=VECTOR ( 'NONE', #41584, 1000.000000000000000 ) ;
#3672=DIRECTION ( 'NONE',  ( 0.000000000000000000, 0.9927088740980530845, -0.1205366802553303057 ) ) ;
#3673=ORIENTED_EDGE ( 'NONE', *, *, #11166, .F. ) ;
#3676=CARTESIAN_POINT ( 'NONE',  ( -332.3517673607765914, -97.52665284734005979, -53.00046796564681983 ) ) ;
#3677=CARTESIAN_POINT ( 'NONE',  ( -336.3521761649653854, -97.07224986041923387, -53.86626052140510978 ) ) ;
#3679=DIRECTION ( 'NONE',  ( 0.000000000000000000, 0.000000000000000000, 1.000000000000000000 ) ) ;
#3680=VECTOR ( 'NONE', #49391, 999.9999999999998863 ) ;
#3693=VERTEX_POINT ( 'NONE', #28853 ) ;
#3699=DIRECTION ( 'NONE',  ( 0.000000000000000000, -0.8229838658936596829, -0.5680647467311510379 ) ) ;
#3707=DIRECTION ( 'NONE',  ( -0.000000000000000000, -0.9350162426854121689, 0.3546048870425426158 ) ) ;
#3711=ORIENTED_EDGE ( 'NONE', *, *, #34319, .T. ) ;
#3712=PLANE ( 'NONE',  #39068 ) ;
#3714=CARTESIAN_POINT ( 'NONE',  ( 0.000000000000000000, 0.000000000000000000, 0.000000000000000000 ) ) ;
#3716=LINE ( 'NONE', #23690, #24076 ) ;
#3717=CARTESIAN_POINT ( 'NONE',  ( -336.3521761649654422, -81.08339623743702873, -41.09453333279329712 ) ) ;
#3718=AXIS2_PLACEMENT_3D ( 'NONE', #6883, #50523, #22662 ) ;
#3727=ORIENTED_EDGE ( 'NONE', *, *, #36804, .F. ) ;
#3728=DIRECTION ( 'NONE',  ( 0.000000000000000000, -7.100801428331730794E-14, -1.000000000000000000 ) ) ;
#3729=PLANE ( 'NONE',  #33747 ) ;
#3735=DIRECTION ( 'NONE',  ( 0.000000000000000000, 0.3546048870425300148, -0.9350162426854169428 ) ) ;
#3738=ORIENTED_EDGE ( 'NONE', *, *, #17339, .F. ) ;
#3739=EDGE_CURVE ( 'NONE', #33568, #23872, #49883, .T. ) ;
#3740=EDGE_LOOP ( 'NONE', ( #42913, #12181, #40442, #47807 ) ) ;
#3741=EDGE_CURVE ( 'NONE', #48449, #15810, #25449, .T. ) ;
#3745=CARTESIAN_POINT ( 'NONE',  ( -339.1964088526558498, -103.0458197858324496, 55.34326076196052213 ) ) ;
#3746=EDGE_LOOP ( 'NONE', ( #32481, #9702, #34359, #32484 ) ) ;
#3747=VERTEX_POINT ( 'NONE', #41736 ) ;
#3748=VECTOR ( 'NONE', #26090, 1000.000000000000000 ) ;
#3750=FACE_OUTER_BOUND ( 'NONE', #23349, .T. ) ;
#3757=CARTESIAN_POINT ( 'NONE',  ( -332.3517673607765914, -85.59754891220836726, -45.24454186338619621 ) ) ;
#3763=FACE_OUTER_BOUND ( 'NONE', #33948, .T. ) ;
#3764=LINE ( 'NONE', #15351, #11756 ) ;
#3765=DIRECTION ( 'NONE',  ( 1.000000000000000000, -0.000000000000000000, 0.000000000000000000 ) ) ;
#3766=EDGE_CURVE ( 'NONE', #44930, #38472, #30060, .T. ) ;
#3773=ADVANCED_FACE ( 'NONE', ( #34367 ), #46026, .T. ) ;
#3774=PRODUCT_DEFINITION_CONTEXT ( 'detailed design', #13556, 'design' ) ;
#3776=CARTESIAN_POINT ( 'NONE',  ( -332.3517673607765914, -64.73342574900661361, 5.491276508483657892 ) ) ;
#3777=CARTESIAN_POINT ( 'NONE',  ( -305.0000000000000568, -78.25935320507912252, 39.41172259083855778 ) ) ;
#3782=DIRECTION ( 'NONE',  ( -0.000000000000000000, 0.9709418174260519008, -0.2393156642875582940 ) ) ;
#3784=LINE ( 'NONE', #50857, #18185 ) ;
#3785=DIRECTION ( 'NONE',  ( -0.000000000000000000, 0.000000000000000000, 1.000000000000000000 ) ) ;
#3786=DIRECTION ( 'NONE',  ( 0.000000000000000000, -0.9927088740980548609, -0.1205366802553164696 ) ) ;
#3787=VERTEX_POINT ( 'NONE', #13615 ) ;
#3788=DIRECTION ( 'NONE',  ( -1.000000000000000000, -0.000000000000000000, 0.000000000000000000 ) ) ;
#3790=ORIENTED_EDGE ( 'NONE', *, *, #42697, .T. ) ;
#3795=CARTESIAN_POINT ( 'NONE',  ( -336.3521761649654422, -66.51961791625839737, 18.79457521708899392 ) ) ;
#3802=LINE ( 'NONE', #114, #45082 ) ;
#3804=ORIENTED_EDGE ( 'NONE', *, *, #20858, .F. ) ;
#3812=ORIENTED_EDGE ( 'NONE', *, *, #28375, .T. ) ;
#3814=EDGE_CURVE ( 'NONE', #32843, #16440, #7545, .T. ) ;
#3818=DIRECTION ( 'NONE',  ( 0.000000000000000000, -0.9709418174260492362, 0.2393156642875685636 ) ) ;
#3826=ADVANCED_FACE ( 'NONE', ( #27240 ), #39336, .F. ) ;
#3827=CARTESIAN_POINT ( 'NONE',  ( -336.3521761649654422, -123.5000000000000284, 0.000000000000000000 ) ) ;
#3828=ORIENTED_EDGE ( 'NONE', *, *, #10318, .F. ) ;
#3834=ORIENTED_EDGE ( 'NONE', *, *, #35036, .F. ) ;
#3843=AXIS2_PLACEMENT_3D ( 'NONE', #29254, #10068, #21108 ) ;
#3844=LINE ( 'NONE', #11451, #3481 ) ;
#3847=VECTOR ( 'NONE', #21598, 1000.000000000000000 ) ;
#3857=CARTESIAN_POINT ( 'NONE',  ( -339.1964088526558498, -79.00630452878473875, -38.74998146212148953 ) ) ;
#3865=ADVANCED_FACE ( 'NONE', ( #26986 ), #26733, .T. ) ;
#3874=PLANE ( 'NONE',  #10434 ) ;
#3875=DIRECTION ( 'NONE',  ( 1.043714542225393697E-14, 0.3546048870425426158, 0.9350162426854121689 ) ) ;
#3877=VERTEX_POINT ( 'NONE', #2817 ) ;
#3879=CIRCLE ( 'NONE', #34113, 60.00000000000000000 ) ;
#3880=DIRECTION ( 'NONE',  ( 1.043714542225393381E-14, -0.9927088740980535286, 0.1205366802553268502 ) ) ;
#3885=VERTEX_POINT ( 'NONE', #14928 ) ;
#3889=DIRECTION ( 'NONE',  ( 0.000000000000000000, 0.000000000000000000, -1.000000000000000000 ) ) ;
#3891=CIRCLE ( 'NONE', #24856, 60.00000000000000000 ) ;
#3897=FACE_OUTER_BOUND ( 'NONE', #9797, .T. ) ;
#3903=EDGE_CURVE ( 'NONE', #4422, #49846, #20395, .T. ) ;
#3907=LINE ( 'NONE', #27556, #19184 ) ;
#3912=ORIENTED_EDGE ( 'NONE', *, *, #17738, .F. ) ;
#3913=CIRCLE ( 'NONE', #23241, 60.00000000000000000 ) ;
#3917=ORIENTED_EDGE ( 'NONE', *, *, #822, .F. ) ;
#3918=PLANE ( 'NONE',  #28953 ) ;
#3919=VERTEX_POINT ( 'NONE', #4129 ) ;
#3923=DIRECTION ( 'NONE',  ( 0.000000000000000000, -0.8854560256532126861, -0.4647231720437631775 ) ) ;
#3924=DIRECTION ( 'NONE',  ( 0.000000000000000000, 3.469446951953614189E-15, -1.000000000000000000 ) ) ;
#3925=ORIENTED_EDGE ( 'NONE', *, *, #31055, .T. ) ;
#3927=LINE ( 'NONE', #8384, #19475 ) ;
#3932=CARTESIAN_POINT ( 'NONE',  ( -330.4913330509368166, -156.6043281241909995, 48.84008046109159551 ) ) ;
#3933=LINE ( 'NONE', #11554, #34979 ) ;
#3939=CIRCLE ( 'NONE', #23224, 5.000000000000001776 ) ;
#3941=DIRECTION ( 'NONE',  ( -1.000000000000000000, 0.000000000000000000, -0.000000000000000000 ) ) ;
#3942=CIRCLE ( 'NONE', #21583, 60.00000000000000000 ) ;
#3947=LINE ( 'NONE', #36501, #12339 ) ;
#3949=EDGE_CURVE ( 'NONE', #41391, #40574, #51970, .T. ) ;
#3951=EDGE_LOOP ( 'NONE', ( #7313, #36599, #49069, #20628 ) ) ;
#3952=AXIS2_PLACEMENT_3D ( 'NONE', #33214, #44528, #648 ) ;
#3955=CARTESIAN_POINT ( 'NONE',  ( -339.1964088526558498, -167.9936954712150339, 38.74998146212178796 ) ) ;
#3958=ORIENTED_EDGE ( 'NONE', *, *, #28314, .F. ) ;
#3960=ORIENTED_EDGE ( 'NONE', *, *, #41705, .F. ) ;
#3962=VECTOR ( 'NONE', #17438, 1000.000000000000000 ) ;
#3964=ADVANCED_FACE ( 'NONE', ( #8825 ), #28530, .F. ) ;
#3967=VECTOR ( 'NONE', #19528, 1000.000000000000000 ) ;
#3969=AXIS2_PLACEMENT_3D ( 'NONE', #12831, #756, #4696 ) ;
#3974=VERTEX_POINT ( 'NONE', #15958 ) ;
#3981=FACE_OUTER_BOUND ( 'NONE', #22537, .T. ) ;
#3982=LINE ( 'NONE', #49944, #44221 ) ;
#3986=VECTOR ( 'NONE', #35379, 1000.000000000000000 ) ;
#3993=AXIS2_PLACEMENT_3D ( 'NONE', #29672, #23539, #2351 ) ;
#3998=CARTESIAN_POINT ( 'NONE',  ( -339.1964088526558498, -172.3400804610910200, 33.10432812419180948 ) ) ;
#4001=CARTESIAN_POINT ( 'NONE',  ( -330.4913330509368166, -64.50000000000000000, -0.4999999999999549249 ) ) ;
#4002=ORIENTED_EDGE ( 'NONE', *, *, #29985, .T. ) ;
#4003=VECTOR ( 'NONE', #22707, 1000.000000000000114 ) ;
#4004=CARTESIAN_POINT ( 'NONE',  ( -332.3517673607765914, -123.5000000000000284, 0.000000000000000000 ) ) ;
#4005=VECTOR ( 'NONE', #12619, 1000.000000000000000 ) ;
#4007=VECTOR ( 'NONE', #22208, 1000.000000000000114 ) ;
#4010=DIRECTION ( 'NONE',  ( 0.000000000000000000, 0.4647231720437573488, -0.8854560256532157947 ) ) ;
#4013=EDGE_CURVE ( 'NONE', #19121, #23268, #161, .T. ) ;
#4015=VECTOR ( 'NONE', #50518, 1000.000000000000000 ) ;
#4019=CARTESIAN_POINT ( 'NONE',  ( -336.3521761649654422, -182.2665742509934148, -5.491276508484069119 ) ) ;
#4024=ORIENTED_EDGE ( 'NONE', *, *, #40394, .F. ) ;
#4027=EDGE_LOOP ( 'NONE', ( #37946, #446, #36105, #51740 ) ) ;
#4028=ORIENTED_EDGE ( 'NONE', *, *, #1089, .T. ) ;
#4029=ADVANCED_FACE ( 'NONE', ( #24597 ), #36954, .F. ) ;
#4034=CARTESIAN_POINT ( 'NONE',  ( -330.4913330509368166, -151.3613951634091848, -52.00954392751743427 ) ) ;
#4036=VERTEX_POINT ( 'NONE', #35919 ) ;
#4038=CARTESIAN_POINT ( 'NONE',  ( -336.3521761649654422, -104.1045282520827300, -55.74477592174792306 ) ) ;
#4043=CARTESIAN_POINT ( 'NONE',  ( -339.1964088526558498, -151.8251501453687808, -52.89315522108996248 ) ) ;
#4044=ORIENTED_EDGE ( 'NONE', *, *, #51658, .F. ) ;
#4047=CARTESIAN_POINT ( 'NONE',  ( -339.1964088526558498, -183.4979166304964622, -0.4999999999999543698 ) ) ;
#4049=VECTOR ( 'NONE', #44692, 1000.000000000000000 ) ;
#4053=DIRECTION ( 'NONE',  ( 0.000000000000000000, 0.5680647467311656929, 0.8229838658936495799 ) ) ;
#4056=CARTESIAN_POINT ( 'NONE',  ( -339.1964088526558498, -123.5000000000000284, 0.000000000000000000 ) ) ;
#4057=DIRECTION ( 'NONE',  ( 0.000000000000000000, 0.000000000000000000, 1.000000000000000000 ) ) ;
#4064=CARTESIAN_POINT ( 'NONE',  ( -339.1964088526558498, -151.3613951634092700, -52.00954392751739164 ) ) ;
#4072=VECTOR ( 'NONE', #47339, 1000.000000000000000 ) ;
#4078=EDGE_CURVE ( 'NONE', #11822, #17726, #24863, .T. ) ;
#4081=ORIENTED_EDGE ( 'NONE', *, *, #19897, .F. ) ;
#4085=DIRECTION ( 'NONE',  ( 0.000000000000000000, 1.410908427127803051E-14, 1.000000000000000000 ) ) ;
#4092=CARTESIAN_POINT ( 'NONE',  ( -332.3517673607765914, -72.48138011061176655, -29.74944317415788930 ) ) ;
#4093=VERTEX_POINT ( 'NONE', #18023 ) ;
#4094=DIRECTION ( 'NONE',  ( 0.000000000000000000, -0.5680647467311596976, -0.8229838658936536877 ) ) ;
#4099=CARTESIAN_POINT ( 'NONE',  ( -339.1964088526558498, -151.3613951634092700, -52.00954392751739164 ) ) ;
#4108=VECTOR ( 'NONE', #7835, 1000.000000000000114 ) ;
#4110=FACE_BOUND ( 'NONE', #36909, .T. ) ;
#4111=DIRECTION ( 'NONE',  ( -0.000000000000000000, 0.5680647467311540355, -0.8229838658936575735 ) ) ;
#4115=EDGE_CURVE ( 'NONE', #28748, #46482, #22532, .T. ) ;
#4119=AXIS2_PLACEMENT_3D ( 'NONE', #32780, #48825, #12794 ) ;
#4124=DIRECTION ( 'NONE',  ( -1.000000000000000000, -0.000000000000000000, 0.000000000000000000 ) ) ;
#4126=EDGE_CURVE ( 'NONE', #29121, #21483, #42624, .T. ) ;
#4129=CARTESIAN_POINT ( 'NONE',  ( -330.4913330509368166, -181.8741440471348483, -13.87297036558341112 ) ) ;
#4132=AXIS2_PLACEMENT_3D ( 'NONE', #9612, #29833, #6464 ) ;
#4133=EDGE_LOOP ( 'NONE', ( #40928, #699, #8104, #34171 ) ) ;
#4136=DIRECTION ( 'NONE',  ( 1.000000000000000000, 8.654812430365571674E-17, -1.050884489711693973E-17 ) ) ;
#4141=VERTEX_POINT ( 'NONE', #49044 ) ;
#4142=LINE ( 'NONE', #23837, #1128 ) ;
#4146=VERTEX_POINT ( 'NONE', #21711 ) ;
#4148=AXIS2_PLACEMENT_3D ( 'NONE', #38844, #43572, #3889 ) ;
#4150=VECTOR ( 'NONE', #32730, 1000.000000000000000 ) ;
#4151=CARTESIAN_POINT ( 'NONE',  ( -332.3517673607765914, -93.75055682584159911, 51.01861988938794923 ) ) ;
#4159=CARTESIAN_POINT ( 'NONE',  ( -330.4913330509368166, -178.4886558749184076, -21.38919645685194837 ) ) ;
#4161=CARTESIAN_POINT ( 'NONE',  ( -330.4913330509368166, -180.6659093959934523, -14.60509510167853442 ) ) ;
#4163=EDGE_LOOP ( 'NONE', ( #18885, #29308, #26466, #37742 ) ) ;
#4168=CARTESIAN_POINT ( 'NONE',  ( -336.3521761649654422, -155.6724726690323450, 49.48329383994676078 ) ) ;
#4169=CARTESIAN_POINT ( 'NONE',  ( -336.3521761649654422, -153.2494431741581025, -51.01861988938816950 ) ) ;
#4170=CARTESIAN_POINT ( 'NONE',  ( 0.000000000000000000, -150.9186671505818822, 52.24190551353965617 ) ) ;
#4173=FACE_OUTER_BOUND ( 'NONE', #5086, .T. ) ;
#4181=EDGE_CURVE ( 'NONE', #31384, #23160, #1983, .T. ) ;
#4186=LINE ( 'NONE', #44115, #32528 ) ;
#4188=EDGE_CURVE ( 'NONE', #23304, #17396, #31382, .T. ) ;
#4192=DIRECTION ( 'NONE',  ( 1.000000000000000000, 0.000000000000000000, 0.000000000000000000 ) ) ;
#4193=DIRECTION ( 'NONE',  ( 1.000000000000000000, 0.000000000000000000, 0.000000000000000000 ) ) ;
#4194=DIRECTION ( 'NONE',  ( 0.000000000000000000, -0.2393156642875547968, 0.9709418174260527890 ) ) ;
#4195=PLANE ( 'NONE',  #35643 ) ;
#4198=CARTESIAN_POINT ( 'NONE',  ( -339.1964088526558498, -123.9999999999993747, 59.00000000000002132 ) ) ;
#4199=CARTESIAN_POINT ( 'NONE',  ( -336.3521761649654422, -142.8954717479169574, 55.74477592174805096 ) ) ;
#4205=EDGE_CURVE ( 'NONE', #41934, #19363, #10382, .T. ) ;
#4208=ORIENTED_EDGE ( 'NONE', *, *, #40350, .F. ) ;
#4212=PLANE ( 'NONE',  #19223 ) ;
#4213=VECTOR ( 'NONE', #10804, 1000.000000000000114 ) ;
#4216=LINE ( 'NONE', #28626, #28711 ) ;
#4224=VERTEX_POINT ( 'NONE', #3286 ) ;
#4227=LINE ( 'NONE', #24714, #24207 ) ;
#4236=EDGE_CURVE ( 'NONE', #14358, #34438, #19058, .T. ) ;
#4240=CARTESIAN_POINT ( 'NONE',  ( -336.3521761649654422, -107.7955183043589500, 56.89493493766750731 ) ) ;
#4242=ORIENTED_EDGE ( 'NONE', *, *, #33719, .T. ) ;
#4248=PLANE ( 'NONE',  #39140 ) ;
#4252=CARTESIAN_POINT ( 'NONE',  ( -339.1964088526558498, -108.6560878169904640, -58.13482838284724608 ) ) ;
#4255=ORIENTED_EDGE ( 'NONE', *, *, #21099, .F. ) ;
#4262=PLANE ( 'NONE',  #50931 ) ;
#4263=EDGE_CURVE ( 'NONE', #5724, #16640, #38747, .T. ) ;
#4267=LINE ( 'NONE', #36316, #24740 ) ;
#4269=ORIENTED_EDGE ( 'NONE', *, *, #4188, .F. ) ;
#4273=VERTEX_POINT ( 'NONE', #43213 ) ;
#4278=PLANE ( 'NONE',  #37027 ) ;
#4286=CARTESIAN_POINT ( 'NONE',  ( -339.1964088526558498, -183.0001959263613287, 7.728304129925186672 ) ) ;
#4295=EDGE_CURVE ( 'NONE', #49438, #12239, #42955, .T. ) ;
#4300=ORIENTED_EDGE ( 'NONE', *, *, #25418, .T. ) ;
#4305=VECTOR ( 'NONE', #35872, 1000.000000000000000 ) ;
#4319=VERTEX_POINT ( 'NONE', #18287 ) ;
#4320=CARTESIAN_POINT ( 'NONE',  ( -330.4913330509368166, -144.8891964568525452, -54.98865587491815177 ) ) ;
#4321=DIRECTION ( 'NONE',  ( 0.000000000000000000, 0.000000000000000000, -1.000000000000000000 ) ) ;
#4328=LINE ( 'NONE', #20351, #23513 ) ;
#4329=LINE ( 'NONE', #49270, #21945 ) ;
#4336=CARTESIAN_POINT ( 'NONE',  ( -339.1964088526558498, -162.2499814621216672, -44.49369547121515467 ) ) ;
#4338=DIRECTION ( 'NONE',  ( 0.000000000000000000, 0.000000000000000000, -1.000000000000000000 ) ) ;
#4339=DIRECTION ( 'NONE',  ( 1.000000000000000000, 0.000000000000000000, -0.000000000000000000 ) ) ;
#4344=ADVANCED_FACE ( 'NONE', ( #16680 ), #32685, .T. ) ;
#4345=LINE ( 'NONE', #48515, #27752 ) ;
#4349=ORIENTED_EDGE ( 'NONE', *, *, #21738, .T. ) ;
#4354=CARTESIAN_POINT ( 'NONE',  ( -330.4913330509368166, -182.0095552316576573, -7.608018572112656308 ) ) ;
#4355=FACE_BOUND ( 'NONE', #45889, .T. ) ;
#4362=ORIENTED_EDGE ( 'NONE', *, *, #38670, .F. ) ;
#4366=LINE ( 'NONE', #20391, #29171 ) ;
#4368=DIRECTION ( 'NONE',  ( 0.000000000000000000, -0.8229838658936516893, 0.5680647467311626952 ) ) ;
#4369=DIRECTION ( 'NONE',  ( -1.000000000000000000, -0.000000000000000000, -0.000000000000000000 ) ) ;
#4370=ORIENTED_EDGE ( 'NONE', *, *, #4499, .F. ) ;
#4371=DIRECTION ( 'NONE',  ( -0.000000000000000000, 0.3546048870425463906, 0.9350162426854107256 ) ) ;
#4373=VERTEX_POINT ( 'NONE', #39525 ) ;
#4377=LINE ( 'NONE', #33006, #40397 ) ;
#4379=DIRECTION ( 'NONE',  ( 1.000000000000000000, 0.000000000000000000, 0.000000000000000000 ) ) ;
#4381=CARTESIAN_POINT ( 'NONE',  ( -305.0000000000000568, -123.9999999999999147, -59.99791663049643375 ) ) ;
#4382=ORIENTED_EDGE ( 'NONE', *, *, #3186, .F. ) ;
#4385=VECTOR ( 'NONE', #9772, 1000.000000000000000 ) ;
#4386=AXIS2_PLACEMENT_3D ( 'NONE', #7790, #30934, #19117 ) ;
#4387=CARTESIAN_POINT ( 'NONE',  ( -339.1964088526558498, -168.0775241366794717, 40.16023333901038228 ) ) ;
#4389=ORIENTED_EDGE ( 'NONE', *, *, #37153, .F. ) ;
#4390=AXIS2_PLACEMENT_3D ( 'NONE', #34627, #2578, #42782 ) ;
#4392=DIRECTION ( 'NONE',  ( -0.000000000000000000, 0.6631226582407937498, -0.7485107481711024136 ) ) ;
#4393=PLANE ( 'NONE',  #39546 ) ;
#4394=EDGE_LOOP ( 'NONE', ( #11410, #25988, #2714, #17981 ) ) ;
#4397=CARTESIAN_POINT ( 'NONE',  ( -305.0000000000000568, -181.8741440471347630, -13.87297036558366692 ) ) ;
#4403=EDGE_CURVE ( 'NONE', #6831, #15659, #4570, .T. ) ;
#4404=ADVANCED_FACE ( 'NONE', ( #44262 ), #11679, .F. ) ;
#4407=ADVANCED_FACE ( 'NONE', ( #43992 ), #31905, .T. ) ;
#4408=VECTOR ( 'NONE', #25531, 1000.000000000000000 ) ;
#4409=ORIENTED_EDGE ( 'NONE', *, *, #16364, .F. ) ;
#4416=ADVANCED_FACE ( 'NONE', ( #16407 ), #39772, .F. ) ;
#4418=VECTOR ( 'NONE', #25132, 1000.000000000000000 ) ;
#4419=EDGE_CURVE ( 'NONE', #49836, #2507, #12698, .T. ) ;
#4420=FACE_OUTER_BOUND ( 'NONE', #20953, .T. ) ;
#4422=VERTEX_POINT ( 'NONE', #24023 ) ;
#4423=CARTESIAN_POINT ( 'NONE',  ( -339.1964088526558498, -162.9984922102927385, -43.83057281297435992 ) ) ;
#4424=CARTESIAN_POINT ( 'NONE',  ( -330.4913330509368166, -162.2499814621210419, 44.49369547121568758 ) ) ;
#4428=ORIENTED_EDGE ( 'NONE', *, *, #47132, .T. ) ;
#4429=EDGE_CURVE ( 'NONE', #32690, #1606, #40037, .T. ) ;
#4433=VERTEX_POINT ( 'NONE', #20081 ) ;
#4435=LINE ( 'NONE', #473, #44798 ) ;
#4439=LINE ( 'NONE', #44114, #37558 ) ;
#4443=CARTESIAN_POINT ( 'NONE',  ( -332.3517673607765914, -129.1091364105427317, 59.73723787327234191 ) ) ;
#4446=DIRECTION ( 'NONE',  ( -1.000000000000000000, -0.000000000000000000, 0.000000000000000000 ) ) ;
#4449=FACE_OUTER_BOUND ( 'NONE', #50031, .T. ) ;
#4452=DIRECTION ( 'NONE',  ( 0.000000000000000000, 0.3546048870425363986, 0.9350162426854146114 ) ) ;
#4454=LINE ( 'NONE', #44408, #25664 ) ;
#4456=CARTESIAN_POINT ( 'NONE',  ( -336.3521761649654422, -93.75055682584159911, 51.01861988938794923 ) ) ;
#4457=VERTEX_POINT ( 'NONE', #9299 ) ;
#4464=ORIENTED_EDGE ( 'NONE', *, *, #49929, .F. ) ;
#4468=AXIS2_PLACEMENT_3D ( 'NONE', #59, #48159, #7934 ) ;
#4472=VERTEX_POINT ( 'NONE', #30041 ) ;
#4475=FACE_OUTER_BOUND ( 'NONE', #11489, .T. ) ;
#4476=EDGE_CURVE ( 'NONE', #29838, #9298, #37669, .T. ) ;
#4477=CIRCLE ( 'NONE', #19586, 20.00000000000001776 ) ;
#4482=EDGE_LOOP ( 'NONE', ( #15533, #11596, #13300, #16661 ) ) ;
#4486=EDGE_CURVE ( 'NONE', #24719, #7018, #21114, .T. ) ;
#4488=LINE ( 'NONE', #27619, #7412 ) ;
#4495=ORIENTED_EDGE ( 'NONE', *, *, #20183, .F. ) ;
#4496=FACE_OUTER_BOUND ( 'NONE', #12150, .T. ) ;
#4498=ORIENTED_EDGE ( 'NONE', *, *, #37863, .T. ) ;
#4499=EDGE_CURVE ( 'NONE', #15154, #22921, #1923, .T. ) ;
#4505=ORIENTED_EDGE ( 'NONE', *, *, #46571, .F. ) ;
#4506=EDGE_CURVE ( 'NONE', #26366, #37592, #10776, .T. ) ;
#4514=VERTEX_POINT ( 'NONE', #1133 ) ;
#4521=DIRECTION ( 'NONE',  ( -0.000000000000000000, -0.8229838658936516893, 0.5680647467311626952 ) ) ;
#4526=DIRECTION ( 'NONE',  ( -0.000000000000000000, -0.5680647467311485954, 0.8229838658936613482 ) ) ;
#4528=CARTESIAN_POINT ( 'NONE',  ( -336.3521761649654422, -82.40546666720629787, 42.41660376256258047 ) ) ;
#4529=DIRECTION ( 'NONE',  ( -0.000000000000000000, -0.5680647467311485954, 0.8229838658936613482 ) ) ;
#4530=DIRECTION ( 'NONE',  ( 0.000000000000000000, 0.7485107481710977506, -0.6631226582407989678 ) ) ;
#4531=CARTESIAN_POINT ( 'NONE',  ( -336.3521761649654422, -160.6539403396202772, 45.90766452162722544 ) ) ;
#4535=ADVANCED_FACE ( 'NONE', ( #49247, #33974, #879, #13242, #21376, #16922, #25323, #50023, #29260, #5359, #24801, #1405, #17460, #6900, #38168, #31321, #22676, #2179, #26089, #42117, #35266, #6141, #39216, #6395, #42379, #43153, #18221, #3225, #42893, #34492, #38688, #26351, #2448, #10328, #38943, #22422, #51316, #34243, #38441, #2952, #26861, #19259, #46341, #22158, #26612, #2692, #7158, #35015, #18991, #42646, #46862, #47111 ), #23198, .T. ) ;
#4543=CARTESIAN_POINT ( 'NONE',  ( -336.3521761649654422, -105.0395444947681369, -56.09938080879045685 ) ) ;
#4545=ORIENTED_EDGE ( 'NONE', *, *, #37759, .T. ) ;
#4547=CARTESIAN_POINT ( 'NONE',  ( -332.3517673607765914, -107.7955183043589500, 56.89493493766750731 ) ) ;
#4548=LINE ( 'NONE', #4822, #47602 ) ;
#4559=DIRECTION ( 'NONE',  ( 0.000000000000000000, 2.937465085987393136E-14, 1.000000000000000000 ) ) ;
#4560=VECTOR ( 'NONE', #2706, 1000.000000000000000 ) ;
#4566=ORIENTED_EDGE ( 'NONE', *, *, #35933, .T. ) ;
#4570=LINE ( 'NONE', #19563, #48567 ) ;
#4573=ORIENTED_EDGE ( 'NONE', *, *, #32378, .F. ) ;
#4574=LINE ( 'NONE', #48729, #43361 ) ;
#4582=DIRECTION ( 'NONE',  ( 0.000000000000000000, -0.7485107481711024136, -0.6631226582407937498 ) ) ;
#4589=EDGE_LOOP ( 'NONE', ( #20479, #13086, #51843, #40986 ) ) ;
#4591=VECTOR ( 'NONE', #1016, 1000.000000000000000 ) ;
#4594=EDGE_CURVE ( 'NONE', #32153, #3411, #16686, .T. ) ;
#4595=VECTOR ( 'NONE', #46478, 1000.000000000000000 ) ;
#4596=LINE ( 'NONE', #21926, #6966 ) ;
#4597=CARTESIAN_POINT ( 'NONE',  ( -339.1964088526558498, -172.3400804610915600, -33.10432812419107051 ) ) ;
#4602=LINE ( 'NONE', #20907, #1489 ) ;
#4604=DIRECTION ( 'NONE',  ( -0.000000000000000000, -0.6631226582407885317, 0.7485107481711069655 ) ) ;
#4605=VECTOR ( 'NONE', #50778, 1000.000000000000000 ) ;
#4607=EDGE_LOOP ( 'NONE', ( #39024, #8177, #27221, #7287 ) ) ;
#4610=DIRECTION ( 'NONE',  ( 0.000000000000000000, 0.000000000000000000, -1.000000000000000000 ) ) ;
#4613=FACE_BOUND ( 'NONE', #18387, .T. ) ;
#4614=FACE_BOUND ( 'NONE', #41051, .T. ) ;
#4618=DIRECTION ( 'NONE',  ( -0.000000000000000000, -0.7485107481711046340, -0.6631226582407911962 ) ) ;
#4619=ORIENTED_EDGE ( 'NONE', *, *, #50811, .F. ) ;
#4623=CARTESIAN_POINT ( 'NONE',  ( -339.1964088526558498, -68.51134412508183402, -21.38919645685240312 ) ) ;
#4627=CARTESIAN_POINT ( 'NONE',  ( -305.0000000000000568, -155.3847370087607374, 50.82679948493869659 ) ) ;
#4632=VECTOR ( 'NONE', #44351, 999.9999999999998863 ) ;
#4633=VERTEX_POINT ( 'NONE', #6657 ) ;
#4634=CARTESIAN_POINT ( 'NONE',  ( -332.3517673607765914, -179.5993808087905279, -18.46045550523168899 ) ) ;
#4636=FACE_OUTER_BOUND ( 'NONE', #47867, .T. ) ;
#4638=AXIS2_PLACEMENT_3D ( 'NONE', #49799, #33507, #41372 ) ;
#4639=LINE ( 'NONE', #16478, #7950 ) ;
#4642=DIRECTION ( 'NONE',  ( -0.000000000000000000, -0.2393156642875516049, 0.9709418174260534551 ) ) ;
#4643=VERTEX_POINT ( 'NONE', #30816 ) ;
#4644=VECTOR ( 'NONE', #42288, 1000.000000000000000 ) ;
#4645=CARTESIAN_POINT ( 'NONE',  ( -339.1964088526558498, -180.9052250602809977, -13.63415328425247885 ) ) ;
#4646=DIRECTION ( 'NONE',  ( -0.000000000000000000, 0.7485107481710934207, -0.6631226582408039638 ) ) ;
#4649=VECTOR ( 'NONE', #10999, 1000.000000000000000 ) ;
#4655=VERTEX_POINT ( 'NONE', #47367 ) ;
#4662=AXIS2_PLACEMENT_3D ( 'NONE', #15567, #15839, #16088 ) ;
#4663=DIRECTION ( 'NONE',  ( -1.000000000000000000, 0.000000000000000000, 0.000000000000000000 ) ) ;
#4665=ORIENTED_EDGE ( 'NONE', *, *, #21636, .T. ) ;
#4666=AXIS2_PLACEMENT_3D ( 'NONE', #1916, #13748, #50018 ) ;
#4669=ORIENTED_EDGE ( 'NONE', *, *, #10521, .T. ) ;
#4678=CARTESIAN_POINT ( 'NONE',  ( -336.3521761649654422, -64.73342574900661361, 5.491276508483657892 ) ) ;
#4682=CARTESIAN_POINT ( 'NONE',  ( -330.4913330509368166, -179.7763290203206452, 20.80804632820240840 ) ) ;
#4684=ORIENTED_EDGE ( 'NONE', *, *, #49713, .F. ) ;
#4686=CARTESIAN_POINT ( 'NONE',  ( -339.1964088526558498, -143.9541802141663709, 55.34326076196097688 ) ) ;
#4689=PLANE ( 'NONE',  #26504 ) ;
#4691=DIRECTION ( 'NONE',  ( 0.000000000000000000, -0.9709418174260492362, 0.2393156642875685636 ) ) ;
#4692=ORIENTED_EDGE ( 'NONE', *, *, #26584, .F. ) ;
#4696=DIRECTION ( 'NONE',  ( 0.000000000000000000, -9.251858538542971828E-16, 1.000000000000000000 ) ) ;
#4699=ORIENTED_EDGE ( 'NONE', *, *, #29231, .T. ) ;
#4700=LINE ( 'NONE', #29123, #19513 ) ;
#4703=CARTESIAN_POINT ( 'NONE',  ( -339.1964088526558498, -64.50000000000000000, -0.5000000000000457412 ) ) ;
#4705=ORIENTED_EDGE ( 'NONE', *, *, #45842, .F. ) ;
#4707=LINE ( 'NONE', #25204, #27232 ) ;
#4709=EDGE_CURVE ( 'NONE', #31272, #15810, #3464, .T. ) ;
#4717=VERTEX_POINT ( 'NONE', #36298 ) ;
#4720=VECTOR ( 'NONE', #364, 1000.000000000000000 ) ;
#4721=LINE ( 'NONE', #16563, #47899 ) ;
#4724=ORIENTED_EDGE ( 'NONE', *, *, #6680, .F. ) ;
#4729=VECTOR ( 'NONE', #46648, 1000.000000000000000 ) ;
#4730=CARTESIAN_POINT ( 'NONE',  ( -332.3517673607765914, -70.03480886230919111, 25.08789112700620194 ) ) ;
#4732=CARTESIAN_POINT ( 'NONE',  ( -336.3521761649654422, -72.48138011061176655, -29.74944317415788930 ) ) ;
#4733=CARTESIAN_POINT ( 'NONE',  ( -340.0000000000000568, -123.5000000000000284, 0.000000000000000000 ) ) ;
#4739=ORIENTED_EDGE ( 'NONE', *, *, #37885, .F. ) ;
#4740=CARTESIAN_POINT ( 'NONE',  ( -336.3521761649654422, -88.64083255475578937, 47.62880233550460218 ) ) ;
#4742=AXIS2_PLACEMENT_3D ( 'NONE', #33545, #12531, #48556 ) ;
#4743=VECTOR ( 'NONE', #2048, 1000.000000000000000 ) ;
#4746=VECTOR ( 'NONE', #34437, 1000.000000000000000 ) ;
#4747=DIRECTION ( 'NONE',  ( 0.000000000000000000, 0.000000000000000000, -1.000000000000000000 ) ) ;
#4748=DIRECTION ( 'NONE',  ( 1.043714542225393381E-14, -0.9350162426854132791, 0.3546048870425396182 ) ) ;
#4749=DIRECTION ( 'NONE',  ( 0.000000000000000000, 0.6631226582407964143, 0.7485107481710999711 ) ) ;
#4752=AXIS2_PLACEMENT_3D ( 'NONE', #6958, #27953, #7985 ) ;
#4757=ORIENTED_EDGE ( 'NONE', *, *, #32273, .F. ) ;
#4759=DIRECTION ( 'NONE',  ( -0.000000000000000000, 0.000000000000000000, -1.000000000000000000 ) ) ;
#4763=DIRECTION ( 'NONE',  ( -0.000000000000000000, 0.8229838658936556861, -0.5680647467311569221 ) ) ;
#4764=EDGE_LOOP ( 'NONE', ( #51388, #22551, #42688, #31227 ) ) ;
#4769=PLANE ( 'NONE',  #29868 ) ;
#4772=LINE ( 'NONE', #28407, #13118 ) ;
#4774=EDGE_CURVE ( 'NONE', #8596, #50621, #39970, .T. ) ;
#4782=VECTOR ( 'NONE', #48998, 1000.000000000000000 ) ;
#4784=CARTESIAN_POINT ( 'NONE',  ( -332.3517673607765914, -123.5000000000000284, 0.000000000000000000 ) ) ;
#4787=AXIS2_PLACEMENT_3D ( 'NONE', #19284, #26641, #39241 ) ;
#4791=EDGE_CURVE ( 'NONE', #30259, #26571, #13373, .T. ) ;
#4793=DIRECTION ( 'NONE',  ( -0.000000000000000000, -0.9709418174260534551, -0.2393156642875516327 ) ) ;
#4796=VECTOR ( 'NONE', #24671, 999.9999999999998863 ) ;
#4797=CARTESIAN_POINT ( 'NONE',  ( -339.1964088526558498, -108.8949048983204051, 57.16590939599314680 ) ) ;
#4805=LINE ( 'NONE', #48946, #27467 ) ;
#4807=ADVANCED_FACE ( 'NONE', ( #13892 ), #33597, .F. ) ;
#4808=VECTOR ( 'NONE', #44705, 1000.000000000000000 ) ;
#4809=LINE ( 'NONE', #1100, #18779 ) ;
#4815=DIRECTION ( 'NONE',  ( 0.000000000000000000, -1.410908427127803051E-14, -1.000000000000000000 ) ) ;
#4816=ORIENTED_EDGE ( 'NONE', *, *, #14898, .T. ) ;
#4817=VERTEX_POINT ( 'NONE', #17587 ) ;
#4822=CARTESIAN_POINT ( 'NONE',  ( -339.1964088526558498, -178.4886558749180949, 21.38919645685277970 ) ) ;
#4828=VECTOR ( 'NONE', #26503, 999.9999999999998863 ) ;
#4829=ORIENTED_EDGE ( 'NONE', *, *, #39321, .T. ) ;
#4830=DIRECTION ( 'NONE',  ( 1.000000000000000000, -0.000000000000000000, 0.000000000000000000 ) ) ;
#4835=ORIENTED_EDGE ( 'NONE', *, *, #22337, .F. ) ;
#4843=EDGE_CURVE ( 'NONE', #8199, #2225, #2573, .T. ) ;
#4847=CIRCLE ( 'NONE', #42604, 60.00000000000000000 ) ;
#4848=CARTESIAN_POINT ( 'NONE',  ( -305.0000000000000568, -115.7716958700755470, -59.50019592636139265 ) ) ;
#4853=CARTESIAN_POINT ( 'NONE',  ( -330.4913330509368166, -123.5000000000000284, 0.000000000000000000 ) ) ;
#4855=CARTESIAN_POINT ( 'NONE',  ( -332.3517673607765914, -92.15051119686104641, -50.05135858667769355 ) ) ;
#4856=ORIENTED_EDGE ( 'NONE', *, *, #1266, .T. ) ;
#4859=CARTESIAN_POINT ( 'NONE',  ( -332.3517673607765914, -65.65568511206123503, -15.93848283698870105 ) ) ;
#4860=CARTESIAN_POINT ( 'NONE',  ( -305.0000000000000568, -182.6878972721721084, 9.838334030658062446 ) ) ;
#4863=ORIENTED_EDGE ( 'NONE', *, *, #5697, .T. ) ;
#4873=DIRECTION ( 'NONE',  ( -1.000000000000000000, 7.812315528781795159E-15, -6.921107616850865492E-15 ) ) ;
#4878=PLANE ( 'NONE',  #18889 ) ;
#4879=VERTEX_POINT ( 'NONE', #6003 ) ;
#4882=PLANE ( 'NONE',  #2594 ) ;
#4884=ORIENTED_EDGE ( 'NONE', *, *, #40643, .T. ) ;
#4886=ORIENTED_EDGE ( 'NONE', *, *, #21660, .F. ) ;
#4892=CARTESIAN_POINT ( 'NONE',  ( -339.1964088526558498, -178.8432607619606358, 20.45418021416736565 ) ) ;
#4895=LINE ( 'NONE', #24852, #44983 ) ;
#4909=DIRECTION ( 'NONE',  ( -1.000000000000000000, 0.000000000000000000, 0.000000000000000000 ) ) ;
#4910=ORIENTED_EDGE ( 'NONE', *, *, #2601, .F. ) ;
#4914=DIRECTION ( 'NONE',  ( -0.000000000000000000, 0.9927088740980556381, 0.1205366802553095307 ) ) ;
#4919=EDGE_LOOP ( 'NONE', ( #12716, #6157, #18491, #35139 ) ) ;
#4920=DIRECTION ( 'NONE',  ( 0.000000000000000000, 0.000000000000000000, 1.000000000000000000 ) ) ;
#4921=LINE ( 'NONE', #1210, #47546 ) ;
#4922=AXIS2_PLACEMENT_3D ( 'NONE', #30473, #1841, #17884 ) ;
#4923=DIRECTION ( 'NONE',  ( 1.000000000000000000, 0.000000000000000000, 0.000000000000000000 ) ) ;
#4926=ORIENTED_EDGE ( 'NONE', *, *, #7852, .T. ) ;
#4929=ORIENTED_EDGE ( 'NONE', *, *, #49046, .T. ) ;
#4935=FACE_OUTER_BOUND ( 'NONE', #16729, .T. ) ;
#4937=VECTOR ( 'NONE', #15751, 1000.000000000000000 ) ;
#4939=LINE ( 'NONE', #20962, #32135 ) ;
#4942=EDGE_CURVE ( 'NONE', #48950, #1552, #14663, .T. ) ;
#4944=ORIENTED_EDGE ( 'NONE', *, *, #48824, .F. ) ;
#4946=ORIENTED_EDGE ( 'NONE', *, *, #21031, .F. ) ;
#4948=AXIS2_PLACEMENT_3D ( 'NONE', #17035, #49079, #41441 ) ;
#4950=EDGE_CURVE ( 'NONE', #43377, #19283, #10971, .T. ) ;
#4956=EDGE_CURVE ( 'NONE', #26038, #49256, #18606, .T. ) ;
#4957=CARTESIAN_POINT ( 'NONE',  ( -332.3517673607765914, -169.4076645216271402, -37.15394033962039089 ) ) ;
#4958=LINE ( 'NONE', #29104, #40756 ) ;
#4961=CARTESIAN_POINT ( 'NONE',  ( -336.3521761649653854, -143.2422018649890276, 56.65902810251888155 ) ) ;
#4967=VERTEX_POINT ( 'NONE', #3086 ) ;
#4968=DIRECTION ( 'NONE',  ( 0.000000000000000000, -0.2393156642875482742, 0.9709418174260544543 ) ) ;
#4977=CARTESIAN_POINT ( 'NONE',  ( -339.1964088526558498, -150.9396941197147726, 53.35787839313415759 ) ) ;
#4978=VECTOR ( 'NONE', #26764, 1000.000000000000000 ) ;
#4979=CARTESIAN_POINT ( 'NONE',  ( -332.3517673607765914, -153.6873197461136442, -51.85292399224849902 ) ) ;
#4982=VECTOR ( 'NONE', #45100, 999.9999999999998863 ) ;
#4988=LINE ( 'NONE', #24678, #50854 ) ;
#4990=VECTOR ( 'NONE', #12276, 1000.000000000000000 ) ;
#4993=ADVANCED_FACE ( 'NONE', ( #47765 ), #11740, .F. ) ;
#4999=ORIENTED_EDGE ( 'NONE', *, *, #11407, .F. ) ;
#5000=VECTOR ( 'NONE', #51137, 1000.000000000000000 ) ;
#5005=ORIENTED_EDGE ( 'NONE', *, *, #41431, .T. ) ;
#5006=DIRECTION ( 'NONE',  ( 0.000000000000000000, 5.157911135237706217E-14, -1.000000000000000000 ) ) ;
#5007=ORIENTED_EDGE ( 'NONE', *, *, #31948, .F. ) ;
#5009=ORIENTED_EDGE ( 'NONE', *, *, #21442, .T. ) ;
#5017=DIRECTION ( 'NONE',  ( -0.000000000000000000, 0.6631226582408039638, 0.7485107481710934207 ) ) ;
#5022=ORIENTED_EDGE ( 'NONE', *, *, #10158, .F. ) ;
#5028=EDGE_CURVE ( 'NONE', #21361, #25289, #6784, .T. ) ;
#5032=ORIENTED_EDGE ( 'NONE', *, *, #46874, .T. ) ;
#5033=EDGE_CURVE ( 'NONE', #16704, #49741, #45003, .T. ) ;
#5034=VECTOR ( 'NONE', #8037, 1000.000000000000000 ) ;
#5035=CARTESIAN_POINT ( 'NONE',  ( -336.3521761649654422, -179.2447759217480154, -19.39547174791710660 ) ) ;
#5045=ORIENTED_EDGE ( 'NONE', *, *, #44887, .F. ) ;
#5051=CARTESIAN_POINT ( 'NONE',  ( -332.3517673607765914, -71.15086438280971493, -29.31839013542551342 ) ) ;
#5056=LINE ( 'NONE', #21863, #37115 ) ;
#5059=EDGE_LOOP ( 'NONE', ( #46114, #4300, #33440, #28529 ) ) ;
#5060=LINE ( 'NONE', #41835, #19892 ) ;
#5061=AXIS2_PLACEMENT_3D ( 'NONE', #2995, #18005, #10886 ) ;
#5065=EDGE_LOOP ( 'NONE', ( #16560, #8801, #35858, #4829 ) ) ;
#5071=ADVANCED_FACE ( 'NONE', ( #51200 ), #15186, .F. ) ;
#5076=EDGE_CURVE ( 'NONE', #32067, #22651, #3879, .T. ) ;
#5077=CARTESIAN_POINT ( 'NONE',  ( -332.3517673607765914, -182.6878972721721084, 9.838334030658062446 ) ) ;
#5085=CARTESIAN_POINT ( 'NONE',  ( -339.1964088526558498, -175.5095439275173135, 27.86139516340941213 ) ) ;
#5086=EDGE_LOOP ( 'NONE', ( #11415, #8588, #17385, #34730 ) ) ;
#5088=EDGE_CURVE ( 'NONE', #45420, #36303, #16214, .T. ) ;
#5089=DIRECTION ( 'NONE',  ( -0.000000000000000000, 0.9709418174260553425, 0.2393156642875449158 ) ) ;
#5092=ORIENTED_EDGE ( 'NONE', *, *, #20266, .T. ) ;
#5110=LINE ( 'NONE', #12965, #22060 ) ;
#5118=EDGE_LOOP ( 'NONE', ( #17205, #8368, #34996, #10046 ) ) ;
#5121=EDGE_LOOP ( 'NONE', ( #8622, #11437, #47841, #17475 ) ) ;
#5123=CARTESIAN_POINT ( 'NONE',  ( -330.4913330509368166, -89.00580675195338642, -49.09328500076577484 ) ) ;
#5124=CARTESIAN_POINT ( 'NONE',  ( -336.3521761649654422, -148.5878911270064009, 53.46519113769075204 ) ) ;
#5129=LINE ( 'NONE', #9070, #13684 ) ;
#5141=DIRECTION ( 'NONE',  ( -1.000000000000000000, 0.000000000000000000, 0.000000000000000000 ) ) ;
#5142=ORIENTED_EDGE ( 'NONE', *, *, #18952, .F. ) ;
#5144=EDGE_CURVE ( 'NONE', #45713, #51152, #11993, .T. ) ;
#5145=CIRCLE ( 'NONE', #35319, 20.00000000000000355 ) ;
#5147=FACE_OUTER_BOUND ( 'NONE', #18775, .T. ) ;
#5149=CARTESIAN_POINT ( 'NONE',  ( -330.0000000000000568, -91.84230854612501105, 0.000000000000000000 ) ) ;
#5150=FACE_BOUND ( 'NONE', #22354, .T. ) ;
#5153=ORIENTED_EDGE ( 'NONE', *, *, #34955, .T. ) ;
#5154=PLANE ( 'NONE',  #39095 ) ;
#5156=ORIENTED_EDGE ( 'NONE', *, *, #44885, .T. ) ;
#5157=CIRCLE ( 'NONE', #1802, 60.00000000000000000 ) ;
#5164=CARTESIAN_POINT ( 'NONE',  ( -336.3521761649654422, -179.5993808087905279, -18.46045550523168899 ) ) ;
#5167=ORIENTED_EDGE ( 'NONE', *, *, #25581, .T. ) ;
#5170=CARTESIAN_POINT ( 'NONE',  ( -305.0000000000000568, -146.2946350401741711, -55.50139289590185854 ) ) ;
#5172=DIRECTION ( 'NONE',  ( -0.000000000000000000, -0.2393156642875482742, 0.9709418174260544543 ) ) ;
#5174=CIRCLE ( 'NONE', #25305, 60.00000000000000000 ) ;
#5175=CARTESIAN_POINT ( 'NONE',  ( -330.4913330509368166, -67.57827586672146936, 21.74306257088659677 ) ) ;
#5178=ORIENTED_EDGE ( 'NONE', *, *, #1586, .F. ) ;
#5179=DIRECTION ( 'NONE',  ( 1.000000000000000000, -0.000000000000000000, -0.000000000000000000 ) ) ;
#5180=VECTOR ( 'NONE', #422, 1000.000000000000114 ) ;
#5189=ORIENTED_EDGE ( 'NONE', *, *, #626, .F. ) ;
#5190=DIRECTION ( 'NONE',  ( 0.000000000000000000, 0.8229838658936633466, 0.5680647467311457088 ) ) ;
#5191=ORIENTED_EDGE ( 'NONE', *, *, #32233, .F. ) ;
#5194=VECTOR ( 'NONE', #34847, 1000.000000000000000 ) ;
#5195=CARTESIAN_POINT ( 'NONE',  ( -332.3517673607765914, -73.44864141332200802, 31.34948880313848107 ) ) ;
#5200=CARTESIAN_POINT ( 'NONE',  ( -332.3517673607765914, -180.1556192733800117, 16.67542351306693149 ) ) ;
#5205=DIRECTION ( 'NONE',  ( 0.000000000000000000, 0.000000000000000000, 1.000000000000000000 ) ) ;
#5213=VECTOR ( 'NONE', #38448, 1000.000000000000000 ) ;
#5215=LINE ( 'NONE', #4957, #51948 ) ;
#5216=LINE ( 'NONE', #52014, #34867 ) ;
#5217=VERTEX_POINT ( 'NONE', #42850 ) ;
#5218=LINE ( 'NONE', #32797, #29886 ) ;
#5219=DIRECTION ( 'NONE',  ( 1.043714542225393697E-14, -0.2393156642875516604, 0.9709418174260535661 ) ) ;
#5220=ORIENTED_EDGE ( 'NONE', *, *, #7819, .T. ) ;
#5221=EDGE_LOOP ( 'NONE', ( #40776, #24432, #19603, #46434 ) ) ;
#5222=ADVANCED_FACE ( 'NONE', ( #27337 ), #22887, .F. ) ;
#5224=ORIENTED_EDGE ( 'NONE', *, *, #5328, .T. ) ;
#5225=PLANE ( 'NONE',  #49132 ) ;
#5233=EDGE_CURVE ( 'NONE', #43120, #38762, #11934, .T. ) ;
#5244=CARTESIAN_POINT ( 'NONE',  ( -336.3521761649654422, -123.5000000000000284, 0.000000000000000000 ) ) ;
#5246=DIRECTION ( 'NONE',  ( 1.000000000000000000, 0.000000000000000000, -0.000000000000000000 ) ) ;
#5251=DIRECTION ( 'NONE',  ( 0.000000000000000000, -0.9927088740980553050, -0.1205366802553130001 ) ) ;
#5256=AXIS2_PLACEMENT_3D ( 'NONE', #17671, #32640, #12658 ) ;
#5259=LINE ( 'NONE', #4732, #22004 ) ;
#5260=FACE_OUTER_BOUND ( 'NONE', #16892, .T. ) ;
#5261=DIRECTION ( 'NONE',  ( -0.000000000000000000, 0.1205366802553199113, -0.9927088740980544168 ) ) ;
#5266=VECTOR ( 'NONE', #38907, 1000.000000000000000 ) ;
#5274=ORIENTED_EDGE ( 'NONE', *, *, #21158, .F. ) ;
#5278=PLANE ( 'NONE',  #23544 ) ;
#5280=CARTESIAN_POINT ( 'NONE',  ( -336.3521761649654422, -176.9651911376907094, -25.08789112700655721 ) ) ;
#5282=ORIENTED_EDGE ( 'NONE', *, *, #15225, .T. ) ;
#5284=DIRECTION ( 'NONE',  ( 0.000000000000000000, 0.8854560256532141294, 0.4647231720437604574 ) ) ;
#5287=AXIS2_PLACEMENT_3D ( 'NONE', #21960, #26408, #22496 ) ;
#5302=FACE_OUTER_BOUND ( 'NONE', #28951, .T. ) ;
#5308=LINE ( 'NONE', #8711, #34163 ) ;
#5310=VECTOR ( 'NONE', #4793, 1000.000000000000114 ) ;
#5311=DIRECTION ( 'NONE',  ( 0.000000000000000000, 0.9350162426854157216, 0.3546048870425330679 ) ) ;
#5314=EDGE_CURVE ( 'NONE', #26602, #39066, #8773, .T. ) ;
#5315=CARTESIAN_POINT ( 'NONE',  ( -330.4913330509368166, -90.39567187580871632, -48.84008046109136814 ) ) ;
#5316=CIRCLE ( 'NONE', #20407, 60.00000000000000000 ) ;
#5318=EDGE_CURVE ( 'NONE', #47080, #28486, #44526, .T. ) ;
#5320=DIRECTION ( 'NONE',  ( -1.000000000000000000, 0.000000000000000000, 0.000000000000000000 ) ) ;
#5322=ORIENTED_EDGE ( 'NONE', *, *, #31274, .T. ) ;
#5323=VECTOR ( 'NONE', #29453, 1000.000000000000000 ) ;
#5328=EDGE_CURVE ( 'NONE', #13273, #42367, #22369, .T. ) ;
#5329=AXIS2_PLACEMENT_3D ( 'NONE', #33932, #40778, #1367 ) ;
#5337=CARTESIAN_POINT ( 'NONE',  ( -339.1964088526558498, -178.8432607619609485, -20.45418021416653076 ) ) ;
#5340=CARTESIAN_POINT ( 'NONE',  ( -339.1964088526558498, -123.5000000000000284, 0.000000000000000000 ) ) ;
#5341=LINE ( 'NONE', #37117, #50980 ) ;
#5342=ORIENTED_EDGE ( 'NONE', *, *, #36627, .T. ) ;
#5344=LINE ( 'NONE', #6123, #5449 ) ;
#5348=CARTESIAN_POINT ( 'NONE',  ( -330.4913330509368166, -115.7716958700747085, 59.50019592636128607 ) ) ;
#5350=DIRECTION ( 'NONE',  ( 0.000000000000000000, 0.4647231720437789981, 0.8854560256532044704 ) ) ;
#5352=ORIENTED_EDGE ( 'NONE', *, *, #51010, .T. ) ;
#5355=VERTEX_POINT ( 'NONE', #4859 ) ;
#5357=AXIS2_PLACEMENT_3D ( 'NONE', #21003, #5246, #1549 ) ;
#5359=FACE_BOUND ( 'NONE', #39863, .T. ) ;
#5360=CARTESIAN_POINT ( 'NONE',  ( -336.3521761649654422, -140.1754235130667610, -56.65561927338005432 ) ) ;
#5363=DIRECTION ( 'NONE',  ( 0.000000000000000000, 0.000000000000000000, 1.000000000000000000 ) ) ;
#5364=EDGE_LOOP ( 'NONE', ( #44418, #14828, #27757, #36654 ) ) ;
#5369=FACE_OUTER_BOUND ( 'NONE', #39839, .T. ) ;
#5373=EDGE_CURVE ( 'NONE', #49836, #42173, #32943, .T. ) ;
#5376=VERTEX_POINT ( 'NONE', #44004 ) ;
#5379=ORIENTED_EDGE ( 'NONE', *, *, #33037, .F. ) ;
#5383=ADVANCED_FACE ( 'NONE', ( #48996 ), #12972, .F. ) ;
#5384=EDGE_LOOP ( 'NONE', ( #26424, #5498, #21444, #49488 ) ) ;
#5389=ORIENTED_EDGE ( 'NONE', *, *, #23139, .T. ) ;
#5390=ADVANCED_FACE ( 'NONE', ( #9562 ), #29779, .F. ) ;
#5395=AXIS2_PLACEMENT_3D ( 'NONE', #8840, #8578, #24611 ) ;
#5398=CARTESIAN_POINT ( 'NONE',  ( -339.1964088526558498, -138.1050951016792681, -57.16590939599323917 ) ) ;
#5403=EDGE_LOOP ( 'NONE', ( #696, #1538, #13803, #32807 ) ) ;
#5404=PLANE ( 'NONE',  #47600 ) ;
#5413=FACE_OUTER_BOUND ( 'NONE', #12856, .T. ) ;
#5419=LINE ( 'NONE', #40347, #43101 ) ;
#5427=CARTESIAN_POINT ( 'NONE',  ( -332.3517673607765914, -179.5993808087905279, -18.46045550523168899 ) ) ;
#5431=EDGE_CURVE ( 'NONE', #28470, #44354, #1145, .T. ) ;
#5435=DIRECTION ( 'NONE',  ( -0.000000000000000000, -0.9927088740980544168, -0.1205366802553199251 ) ) ;
#5438=DIRECTION ( 'NONE',  ( 0.000000000000000000, -0.2393156642875582940, -0.9709418174260519008 ) ) ;
#5441=LINE ( 'NONE', #21459, #21098 ) ;
#5442=LINE ( 'NONE', #21461, #5596 ) ;
#5446=ORIENTED_EDGE ( 'NONE', *, *, #23615, .T. ) ;
#5449=VECTOR ( 'NONE', #22660, 1000.000000000000000 ) ;
#5450=ORIENTED_EDGE ( 'NONE', *, *, #16291, .F. ) ;
#5452=CARTESIAN_POINT ( 'NONE',  ( -332.3517673607765914, -174.9833430614318388, 28.86398714850502856 ) ) ;
#5457=ADVANCED_FACE ( 'NONE', ( #46355 ), #10339, .F. ) ;
#5461=ADVANCED_FACE ( 'NONE', ( #37684 ), #17977, .F. ) ;
#5465=AXIS2_PLACEMENT_3D ( 'NONE', #39585, #12448, #40817 ) ;
#5467=DIRECTION ( 'NONE',  ( 1.000000000000000000, 0.000000000000000000, 0.000000000000000000 ) ) ;
#5478=CARTESIAN_POINT ( 'NONE',  ( -490.0000000000001137, -78.50000000000002842, 0.000000000000000000 ) ) ;
#5479=VERTEX_POINT ( 'NONE', #14815 ) ;
#5480=ORIENTED_EDGE ( 'NONE', *, *, #42728, .F. ) ;
#5484=FACE_OUTER_BOUND ( 'NONE', #38565, .T. ) ;
#5486=ORIENTED_EDGE ( 'NONE', *, *, #50907, .F. ) ;
#5487=DIRECTION ( 'NONE',  ( 1.043714542225393223E-14, 0.9709418174260544543, 0.2393156642875482742 ) ) ;
#5498=ORIENTED_EDGE ( 'NONE', *, *, #14342, .F. ) ;
#5506=CARTESIAN_POINT ( 'NONE',  ( 0.000000000000000000, -116.3883358649361526, -58.56982357178523557 ) ) ;
#5507=LINE ( 'NONE', #5774, #21471 ) ;
#5513=AXIS2_PLACEMENT_3D ( 'NONE', #45265, #17134, #5311 ) ;
#5516=ORIENTED_EDGE ( 'NONE', *, *, #27962, .F. ) ;
#5520=DIRECTION ( 'NONE',  ( 1.000000000000000000, -0.000000000000000000, -0.000000000000000000 ) ) ;
#5523=EDGE_CURVE ( 'NONE', #28004, #41662, #34757, .T. ) ;
#5531=VERTEX_POINT ( 'NONE', #26871 ) ;
#5534=ORIENTED_EDGE ( 'NONE', *, *, #35670, .F. ) ;
#5538=ORIENTED_EDGE ( 'NONE', *, *, #3513, .T. ) ;
#5539=FACE_OUTER_BOUND ( 'NONE', #47773, .T. ) ;
#5540=DIRECTION ( 'NONE',  ( 0.000000000000000000, 0.8229838658936596829, 0.5680647467311510379 ) ) ;
#5543=DIRECTION ( 'NONE',  ( 0.000000000000000000, -0.4647231720437604574, 0.8854560256532141294 ) ) ;
#5544=AXIS2_PLACEMENT_3D ( 'NONE', #12581, #25454, #12837 ) ;
#5546=DIRECTION ( 'NONE',  ( -0.000000000000000000, 0.9927088740980556381, 0.1205366802553095307 ) ) ;
#5547=ORIENTED_EDGE ( 'NONE', *, *, #39111, .T. ) ;
#5548=VECTOR ( 'NONE', #7871, 1000.000000000000000 ) ;
#5550=CARTESIAN_POINT ( 'NONE',  ( -339.1964088526558498, -175.5095439275177398, -27.86139516340860212 ) ) ;
#5552=EDGE_LOOP ( 'NONE', ( #1172, #27171, #17097, #40327 ) ) ;
#5556=DIRECTION ( 'NONE',  ( 0.000000000000000000, 0.000000000000000000, -1.000000000000000000 ) ) ;
#5560=CARTESIAN_POINT ( 'NONE',  ( -330.4913330509368166, -172.3400804610915031, -33.10432812419114157 ) ) ;
#5565=EDGE_CURVE ( 'NONE', #11626, #29097, #37485, .T. ) ;
#5570=FACE_OUTER_BOUND ( 'NONE', #33249, .T. ) ;
#5571=ORIENTED_EDGE ( 'NONE', *, *, #12162, .F. ) ;
#5574=DIRECTION ( 'NONE',  ( 1.000000000000000000, 7.719741424018471827E-17, -4.051632851310729971E-17 ) ) ;
#5580=EDGE_CURVE ( 'NONE', #37674, #51994, #19273, .T. ) ;
#5581=CARTESIAN_POINT ( 'NONE',  ( -330.4913330509368166, -172.3400804610915031, -33.10432812419114157 ) ) ;
#5582=LINE ( 'NONE', #42335, #42944 ) ;
#5592=VECTOR ( 'NONE', #40750, 1000.000000000000000 ) ;
#5596=VECTOR ( 'NONE', #1487, 1000.000000000000000 ) ;
#5597=CIRCLE ( 'NONE', #44175, 60.00000000000000000 ) ;
#5602=AXIS2_PLACEMENT_3D ( 'NONE', #1908, #18211, #5350 ) ;
#5613=DIRECTION ( 'NONE',  ( 1.000000000000000000, 0.000000000000000000, 0.000000000000000000 ) ) ;
#5615=ORIENTED_EDGE ( 'NONE', *, *, #16077, .T. ) ;
#5618=LINE ( 'NONE', #18214, #15588 ) ;
#5619=AXIS2_PLACEMENT_3D ( 'NONE', #28997, #41101, #37152 ) ;
#5627=EDGE_CURVE ( 'NONE', #34284, #51297, #3477, .T. ) ;
#5631=ORIENTED_EDGE ( 'NONE', *, *, #39886, .T. ) ;
#5638=AXIS2_PLACEMENT_3D ( 'NONE', #44247, #12945, #28970 ) ;
#5639=VECTOR ( 'NONE', #41599, 1000.000000000000114 ) ;
#5640=LINE ( 'NONE', #24812, #50869 ) ;
#5653=ORIENTED_EDGE ( 'NONE', *, *, #12058, .F. ) ;
#5667=ORIENTED_EDGE ( 'NONE', *, *, #625, .F. ) ;
#5668=VERTEX_POINT ( 'NONE', #31593 ) ;
#5669=LINE ( 'NONE', #21690, #51765 ) ;
#5671=VECTOR ( 'NONE', #3267, 1000.000000000000000 ) ;
#5675=VERTEX_POINT ( 'NONE', #47649 ) ;
#5678=CIRCLE ( 'NONE', #19911, 60.00000000000000000 ) ;
#5679=VECTOR ( 'NONE', #34224, 1000.000000000000114 ) ;
#5682=ORIENTED_EDGE ( 'NONE', *, *, #51445, .F. ) ;
#5683=VERTEX_POINT ( 'NONE', #43942 ) ;
#5689=EDGE_CURVE ( 'NONE', #35564, #17216, #23965, .T. ) ;
#5695=CIRCLE ( 'NONE', #41770, 60.00000000000000000 ) ;
#5696=VECTOR ( 'NONE', #7358, 1000.000000000000114 ) ;
#5697=EDGE_CURVE ( 'NONE', #2241, #4717, #24238, .T. ) ;
#5698=CARTESIAN_POINT ( 'NONE',  ( -305.0000000000000568, -68.38646289696045244, -23.71704087764493707 ) ) ;
#5701=EDGE_CURVE ( 'NONE', #37855, #5355, #47897, .T. ) ;
#5703=DIRECTION ( 'NONE',  ( 0.000000000000000000, 1.119474883163699554E-13, 1.000000000000000000 ) ) ;
#5704=FACE_OUTER_BOUND ( 'NONE', #48178, .T. ) ;
#5705=DIRECTION ( 'NONE',  ( 0.000000000000000000, -0.2393156642875615969, -0.9709418174260511236 ) ) ;
#5710=LINE ( 'NONE', #34063, #6333 ) ;
#5712=VECTOR ( 'NONE', #3008, 1000.000000000000000 ) ;
#5715=ORIENTED_EDGE ( 'NONE', *, *, #4078, .F. ) ;
#5717=CARTESIAN_POINT ( 'NONE',  ( -336.3521761649654422, -171.1288023355047585, 34.85916744524404720 ) ) ;
#5723=ORIENTED_EDGE ( 'NONE', *, *, #16135, .F. ) ;
#5724=VERTEX_POINT ( 'NONE', #12127 ) ;
#5728=CARTESIAN_POINT ( 'NONE',  ( -305.0000000000000568, -67.57827586672146936, 21.74306257088660033 ) ) ;
#5734=VECTOR ( 'NONE', #41376, 1000.000000000000000 ) ;
#5735=EDGE_CURVE ( 'NONE', #41896, #2959, #19761, .T. ) ;
#5736=ADVANCED_FACE ( 'NONE', ( #575 ), #4262, .F. ) ;
#5738=ADVANCED_FACE ( 'NONE', ( #32882 ), #6482, .T. ) ;
#5740=LINE ( 'NONE', #29364, #29014 ) ;
#5743=EDGE_LOOP ( 'NONE', ( #18146, #6930, #2470, #10476 ) ) ;
#5749=DIRECTION ( 'NONE',  ( -0.000000000000000000, 0.1205366802553337752, 0.9927088740980526405 ) ) ;
#5750=VERTEX_POINT ( 'NONE', #36058 ) ;
#5753=EDGE_LOOP ( 'NONE', ( #7508, #25857, #12183, #41979 ) ) ;
#5757=EDGE_CURVE ( 'NONE', #11859, #6229, #44470, .T. ) ;
#5758=VECTOR ( 'NONE', #51241, 1000.000000000000000 ) ;
#5759=VERTEX_POINT ( 'NONE', #36572 ) ;
#5762=ADVANCED_FACE ( 'NONE', ( #36844 ), #24484, .F. ) ;
#5764=PLANE ( 'NONE',  #10607 ) ;
#5765=EDGE_LOOP ( 'NONE', ( #38353, #31103, #4269, #20447 ) ) ;
#5770=DIRECTION ( 'NONE',  ( 0.000000000000000000, 0.000000000000000000, 1.000000000000000000 ) ) ;
#5774=CARTESIAN_POINT ( 'NONE',  ( -332.3517673607765914, -139.2044816956407089, -56.89493493766761389 ) ) ;
#5775=EDGE_CURVE ( 'NONE', #10671, #38308, #45949, .T. ) ;
#5777=ORIENTED_EDGE ( 'NONE', *, *, #50348, .F. ) ;
#5786=ORIENTED_EDGE ( 'NONE', *, *, #13438, .F. ) ;
#5793=FACE_OUTER_BOUND ( 'NONE', #8511, .T. ) ;
#5794=PLANE ( 'NONE',  #3993 ) ;
#5797=AXIS2_PLACEMENT_3D ( 'NONE', #19622, #46715, #26731 ) ;
#5798=DIRECTION ( 'NONE',  ( 0.000000000000000000, 0.6631226582407911962, -0.7485107481711046340 ) ) ;
#5801=ORIENTED_EDGE ( 'NONE', *, *, #9274, .T. ) ;
#5806=EDGE_CURVE ( 'NONE', #29626, #21379, #30806, .T. ) ;
#5807=EDGE_CURVE ( 'NONE', #29662, #1527, #41826, .T. ) ;
#5811=LINE ( 'NONE', #5280, #674 ) ;
#5812=LINE ( 'NONE', #29428, #24154 ) ;
#5819=VECTOR ( 'NONE', #27024, 1000.000000000000000 ) ;
#5821=CARTESIAN_POINT ( 'NONE',  ( -180.0000000000000568, -123.5000000000000284, 0.000000000000000000 ) ) ;
#5823=VERTEX_POINT ( 'NONE', #33924 ) ;
#5825=AXIS2_PLACEMENT_3D ( 'NONE', #35611, #26705, #11703 ) ;
#5832=DIRECTION ( 'NONE',  ( -1.000000000000000000, 0.000000000000000000, -0.000000000000000000 ) ) ;
#5834=CARTESIAN_POINT ( 'NONE',  ( -336.3521761649654422, -159.1821513111375452, -47.06073758877369073 ) ) ;
#5839=VECTOR ( 'NONE', #30740, 1000.000000000000114 ) ;
#5842=CARTESIAN_POINT ( 'NONE',  ( -339.1964088526558498, -180.9052250602809977, -13.63415328425247885 ) ) ;
#5846=PLANE ( 'NONE',  #32142 ) ;
#5853=ORIENTED_EDGE ( 'NONE', *, *, #46719, .T. ) ;
#5854=CARTESIAN_POINT ( 'NONE',  ( -339.1964088526558498, -96.52406086224443982, -52.47426709956138069 ) ) ;
#5857=ORIENTED_EDGE ( 'NONE', *, *, #49963, .T. ) ;
#5861=EDGE_CURVE ( 'NONE', #40560, #34017, #13967, .T. ) ;
#5865=VECTOR ( 'NONE', #11967, 1000.000000000000000 ) ;
#5868=ORIENTED_EDGE ( 'NONE', *, *, #46874, .F. ) ;
#5873=PLANE ( 'NONE',  #25762 ) ;
#5881=ORIENTED_EDGE ( 'NONE', *, *, #24044, .T. ) ;
#5882=EDGE_CURVE ( 'NONE', #19062, #46515, #29722, .T. ) ;
#5884=ORIENTED_EDGE ( 'NONE', *, *, #20803, .T. ) ;
#5891=ORIENTED_EDGE ( 'NONE', *, *, #6062, .T. ) ;
#5893=DIRECTION ( 'NONE',  ( -1.000000000000000000, -9.241633304753572918E-15, -4.850383327711924655E-15 ) ) ;
#5896=FACE_OUTER_BOUND ( 'NONE', #48791, .T. ) ;
#5897=DIRECTION ( 'NONE',  ( 1.000000000000000000, -0.000000000000000000, -0.000000000000000000 ) ) ;
#5907=LINE ( 'NONE', #45587, #44643 ) ;
#5911=FACE_OUTER_BOUND ( 'NONE', #18914, .T. ) ;
#5913=VECTOR ( 'NONE', #39102, 1000.000000000000000 ) ;
#5916=LINE ( 'NONE', #38476, #34236 ) ;
#5917=DIRECTION ( 'NONE',  ( -0.000000000000000000, 0.000000000000000000, -1.000000000000000000 ) ) ;
#5918=ADVANCED_FACE ( 'NONE', ( #25026 ), #37626, .F. ) ;
#5922=VERTEX_POINT ( 'NONE', #27329 ) ;
#5925=CARTESIAN_POINT ( 'NONE',  ( -330.4913330509368166, -144.8891964568525452, -54.98865587491815177 ) ) ;
#5926=CARTESIAN_POINT ( 'NONE',  ( -336.3521761649654422, -64.50000000000000000, -1.632288850093980725 ) ) ;
#5927=EDGE_CURVE ( 'NONE', #25253, #13273, #47323, .T. ) ;
#5930=ORIENTED_EDGE ( 'NONE', *, *, #5076, .T. ) ;
#5931=AXIS2_PLACEMENT_3D ( 'NONE', #16061, #43404, #6877 ) ;
#5935=VERTEX_POINT ( 'NONE', #38643 ) ;
#5938=CARTESIAN_POINT ( 'NONE',  ( -305.0000000000000568, -123.5000000000000142, 60.00000000000000000 ) ) ;
#5943=VERTEX_POINT ( 'NONE', #42326 ) ;
#5944=ORIENTED_EDGE ( 'NONE', *, *, #16377, .T. ) ;
#5954=LINE ( 'NONE', #29851, #45062 ) ;
#5955=ORIENTED_EDGE ( 'NONE', *, *, #23102, .T. ) ;
#5956=DIRECTION ( 'NONE',  ( -0.000000000000000000, -0.9709418174260502354, 0.2393156642875652051 ) ) ;
#5960=VERTEX_POINT ( 'NONE', #46813 ) ;
#5964=CARTESIAN_POINT ( 'NONE',  ( -305.0000000000000568, -132.3499116637027271, -59.34373651485605450 ) ) ;
#5968=DIRECTION ( 'NONE',  ( -1.000000000000000000, 0.000000000000000000, 0.000000000000000000 ) ) ;
#5970=VERTEX_POINT ( 'NONE', #7382 ) ;
#5975=CARTESIAN_POINT ( 'NONE',  ( -336.3521761649654422, -146.8829211657874794, -54.23253582808848705 ) ) ;
#5979=CARTESIAN_POINT ( 'NONE',  ( -339.1964088526558498, -180.9052250602809977, -13.63415328425247885 ) ) ;
#5988=DIRECTION ( 'NONE',  ( 0.000000000000000000, -7.285838599102589797E-14, 1.000000000000000000 ) ) ;
#5991=LINE ( 'NONE', #38563, #1987 ) ;
#5996=VECTOR ( 'NONE', #11750, 999.9999999999998863 ) ;
#5999=CARTESIAN_POINT ( 'NONE',  ( 0.000000000000000000, -123.4999999999994174, 59.00000000000002132 ) ) ;
#6001=CARTESIAN_POINT ( 'NONE',  ( -339.1964088526558498, -171.7720157143598669, 33.92731199008546383 ) ) ;
#6003=CARTESIAN_POINT ( 'NONE',  ( -332.3517673607765914, -182.1255794688777314, -12.76876783163923967 ) ) ;
#6008=DIRECTION ( 'NONE',  ( -0.000000000000000000, -0.8854560256532079121, 0.4647231720437724478 ) ) ;
#6009=CARTESIAN_POINT ( 'NONE',  ( -339.1964088526558498, -180.6659093959932250, 14.60509510167942437 ) ) ;
#6020=ORIENTED_EDGE ( 'NONE', *, *, #8147, .F. ) ;
#6023=VERTEX_POINT ( 'NONE', #47064 ) ;
#6024=EDGE_CURVE ( 'NONE', #50020, #4319, #38900, .T. ) ;
#6027=CARTESIAN_POINT ( 'NONE',  ( -305.0000000000000568, -93.31268025388605736, 51.85292399224828586 ) ) ;
#6029=EDGE_CURVE ( 'NONE', #33953, #21286, #11039, .T. ) ;
#6031=CARTESIAN_POINT ( 'NONE',  ( -336.3521761649654422, -105.0395444947681369, -56.09938080879045685 ) ) ;
#6035=ORIENTED_EDGE ( 'NONE', *, *, #2411, .T. ) ;
#6037=AXIS2_PLACEMENT_3D ( 'NONE', #46301, #50753, #10800 ) ;
#6039=ORIENTED_EDGE ( 'NONE', *, *, #50259, .T. ) ;
#6040=DIRECTION ( 'NONE',  ( -1.000000000000000000, 0.000000000000000000, 0.000000000000000000 ) ) ;
#6044=EDGE_CURVE ( 'NONE', #44797, #31178, #6609, .T. ) ;
#6048=ORIENTED_EDGE ( 'NONE', *, *, #17002, .F. ) ;
#6050=LINE ( 'NONE', #25495, #17454 ) ;
#6056=DIRECTION ( 'NONE',  ( -1.000000000000000000, 0.000000000000000000, 0.000000000000000000 ) ) ;
#6057=ORIENTED_EDGE ( 'NONE', *, *, #38339, .F. ) ;
#6059=DIRECTION ( 'NONE',  ( 0.000000000000000000, 0.000000000000000000, 1.000000000000000000 ) ) ;
#6060=DIRECTION ( 'NONE',  ( 0.000000000000000000, 0.000000000000000000, -1.000000000000000000 ) ) ;
#6061=VERTEX_POINT ( 'NONE', #11809 ) ;
#6062=EDGE_CURVE ( 'NONE', #15284, #8221, #3947, .T. ) ;
#6072=DIRECTION ( 'NONE',  ( -0.000000000000000000, -0.9927088740980530845, 0.1205366802553303057 ) ) ;
#6083=LINE ( 'NONE', #21857, #3847 ) ;
#6084=FACE_OUTER_BOUND ( 'NONE', #32766, .T. ) ;
#6085=EDGE_CURVE ( 'NONE', #15537, #14073, #48087, .T. ) ;
#6089=ADVANCED_FACE ( 'NONE', ( #44139 ), #24182, .T. ) ;
#6091=CIRCLE ( 'NONE', #48893, 60.00000000000000000 ) ;
#6093=PLANE ( 'NONE',  #1954 ) ;
#6095=ADVANCED_FACE ( 'NONE', ( #12596 ), #242, .T. ) ;
#6097=ADVANCED_FACE ( 'NONE', ( #778 ), #7623, .F. ) ;
#6102=DIRECTION ( 'NONE',  ( 1.000000000000000000, -0.000000000000000000, -0.000000000000000000 ) ) ;
#6105=CARTESIAN_POINT ( 'NONE',  ( -365.0000000000001137, -78.50000000000002842, 0.000000000000000000 ) ) ;
#6108=EDGE_CURVE ( 'NONE', #16449, #2507, #16099, .T. ) ;
#6109=ORIENTED_EDGE ( 'NONE', *, *, #19130, .T. ) ;
#6111=VECTOR ( 'NONE', #9424, 1000.000000000000000 ) ;
#6118=CARTESIAN_POINT ( 'NONE',  ( -336.3521761649654422, -179.2447759217480154, -19.39547174791710660 ) ) ;
#6119=CARTESIAN_POINT ( 'NONE',  ( -330.4913330509368166, -68.15673923803900891, 20.45418021416622878 ) ) ;
#6121=FACE_OUTER_BOUND ( 'NONE', #45040, .T. ) ;
#6122=ORIENTED_EDGE ( 'NONE', *, *, #13376, .T. ) ;
#6123=CARTESIAN_POINT ( 'NONE',  ( -305.0000000000000568, -149.9277501395804677, 53.86626052140529453 ) ) ;
#6125=DIRECTION ( 'NONE',  ( 0.000000000000000000, 0.000000000000000000, -1.000000000000000000 ) ) ;
#6127=DIRECTION ( 'NONE',  ( 0.000000000000000000, -0.8854560256532043594, 0.4647231720437789981 ) ) ;
#6134=VERTEX_POINT ( 'NONE', #23900 ) ;
#6139=CARTESIAN_POINT ( 'NONE',  ( -332.3517673607765914, -64.61288906875131488, 4.498567634385603142 ) ) ;
#6141=FACE_BOUND ( 'NONE', #47443, .T. ) ;
#6143=ORIENTED_EDGE ( 'NONE', *, *, #45690, .F. ) ;
#6150=ADVANCED_FACE ( 'NONE', ( #45453 ), #33089, .F. ) ;
#6155=ORIENTED_EDGE ( 'NONE', *, *, #7411, .T. ) ;
#6156=CARTESIAN_POINT ( 'NONE',  ( -336.3521761649654422, -72.48138011061176655, -29.74944317415788930 ) ) ;
#6157=ORIENTED_EDGE ( 'NONE', *, *, #8623, .F. ) ;
#6162=VERTEX_POINT ( 'NONE', #33611 ) ;
#6166=DIRECTION ( 'NONE',  ( 0.000000000000000000, 0.1205366802553233113, 0.9927088740980538617 ) ) ;
#6169=DIRECTION ( 'NONE',  ( 0.000000000000000000, -0.7485107481710954191, 0.6631226582408017434 ) ) ;
#6170=EDGE_CURVE ( 'NONE', #40642, #29348, #24958, .T. ) ;
#6173=FACE_OUTER_BOUND ( 'NONE', #35747, .T. ) ;
#6179=EDGE_CURVE ( 'NONE', #19768, #24889, #32828, .T. ) ;
#6181=LINE ( 'NONE', #30332, #46771 ) ;
#6185=VECTOR ( 'NONE', #31798, 999.9999999999998863 ) ;
#6189=ORIENTED_EDGE ( 'NONE', *, *, #13664, .T. ) ;
#6190=CARTESIAN_POINT ( 'NONE',  ( -339.1964088526558498, -71.02573290043838483, 26.97593913775504504 ) ) ;
#6191=EDGE_LOOP ( 'NONE', ( #2211, #45285, #45421, #12883 ) ) ;
#6195=DIRECTION ( 'NONE',  ( -1.000000000000000000, 0.000000000000000000, -0.000000000000000000 ) ) ;
#6198=AXIS2_PLACEMENT_3D ( 'NONE', #27633, #15825, #24216 ) ;
#6202=DIRECTION ( 'NONE',  ( -8.718379230999705894E-17, 0.9709418174260527890, 0.2393156642875547968 ) ) ;
#6210=CARTESIAN_POINT ( 'NONE',  ( -305.0000000000000568, -128.1121410293017391, 59.82247199109905011 ) ) ;
#6212=ORIENTED_EDGE ( 'NONE', *, *, #21604, .T. ) ;
#6213=LINE ( 'NONE', #33287, #17249 ) ;
#6219=AXIS2_PLACEMENT_3D ( 'NONE', #7555, #29061, #5703 ) ;
#6220=DIRECTION ( 'NONE',  ( 1.000000000000000000, -0.000000000000000000, 0.000000000000000000 ) ) ;
#6221=DIRECTION ( 'NONE',  ( 1.000000000000000000, -0.000000000000000000, -0.000000000000000000 ) ) ;
#6222=CARTESIAN_POINT ( 'NONE',  ( -330.4913330509368166, -123.5000000000000284, 0.000000000000000000 ) ) ;
#6225=CARTESIAN_POINT ( 'NONE',  ( -330.4913330509368166, -64.50000000000000000, -0.4999999999999549249 ) ) ;
#6226=DIRECTION ( 'NONE',  ( 1.000000000000000000, -0.000000000000000000, -0.000000000000000000 ) ) ;
#6227=VECTOR ( 'NONE', #50769, 1000.000000000000000 ) ;
#6228=CYLINDRICAL_SURFACE ( 'NONE', #16505, 15.24495751795539000 ) ;
#6229=VERTEX_POINT ( 'NONE', #49906 ) ;
#6237=ORIENTED_EDGE ( 'NONE', *, *, #7064, .F. ) ;
#6245=LINE ( 'NONE', #6771, #25803 ) ;
#6246=CIRCLE ( 'NONE', #26383, 60.00000000000000000 ) ;
#6251=DIRECTION ( 'NONE',  ( -0.000000000000000000, -0.2393156642875582940, -0.9709418174260519008 ) ) ;
#6252=VERTEX_POINT ( 'NONE', #13122 ) ;
#6254=ORIENTED_EDGE ( 'NONE', *, *, #12762, .F. ) ;
#6255=VECTOR ( 'NONE', #8772, 1000.000000000000000 ) ;
#6257=ORIENTED_EDGE ( 'NONE', *, *, #50887, .F. ) ;
#6262=CARTESIAN_POINT ( 'NONE',  ( -339.1964088526558498, -175.9742670995610752, 26.97593913775620678 ) ) ;
#6269=VECTOR ( 'NONE', #34786, 1000.000000000000000 ) ;
#6275=EDGE_CURVE ( 'NONE', #29000, #44562, #1025, .T. ) ;
#6281=ORIENTED_EDGE ( 'NONE', *, *, #13746, .T. ) ;
#6282=PLANE ( 'NONE',  #47774 ) ;
#6286=VECTOR ( 'NONE', #39124, 1000.000000000000000 ) ;
#6288=CARTESIAN_POINT ( 'NONE',  ( -339.1964088526558498, -123.5000000000000284, 0.000000000000000000 ) ) ;
#6289=DIRECTION ( 'NONE',  ( 0.000000000000000000, 0.000000000000000000, 1.000000000000000000 ) ) ;
#6297=CARTESIAN_POINT ( 'NONE',  ( -305.0000000000000568, -181.6348283828473029, -14.84391218300937787 ) ) ;
#6301=CARTESIAN_POINT ( 'NONE',  ( -336.3521761649654422, -65.58448481710581746, 11.56382487286456140 ) ) ;
#6305=EDGE_LOOP ( 'NONE', ( #21020, #18478 ) ) ;
#6308=FACE_OUTER_BOUND ( 'NONE', #45390, .T. ) ;
#6309=VERTEX_POINT ( 'NONE', #37029 ) ;
#6312=FACE_OUTER_BOUND ( 'NONE', #11195, .T. ) ;
#6315=ORIENTED_EDGE ( 'NONE', *, *, #24543, .F. ) ;
#6317=CARTESIAN_POINT ( 'NONE',  ( -336.3521761649654422, -104.1045282520827300, -55.74477592174792306 ) ) ;
#6333=VECTOR ( 'NONE', #21203, 1000.000000000000114 ) ;
#6337=EDGE_CURVE ( 'NONE', #43448, #32451, #50880, .T. ) ;
#6339=LINE ( 'NONE', #13964, #42029 ) ;
#6342=EDGE_CURVE ( 'NONE', #13387, #2972, #32023, .T. ) ;
#6345=VERTEX_POINT ( 'NONE', #23282 ) ;
#6353=CARTESIAN_POINT ( 'NONE',  ( 0.000000000000000000, -66.21443277186274656, 14.11962419296515137 ) ) ;
#6355=DIRECTION ( 'NONE',  ( 0.000000000000000000, 0.000000000000000000, 1.000000000000000000 ) ) ;
#6357=ORIENTED_EDGE ( 'NONE', *, *, #51794, .F. ) ;
#6358=VECTOR ( 'NONE', #28984, 1000.000000000000000 ) ;
#6359=ORIENTED_EDGE ( 'NONE', *, *, #25945, .F. ) ;
#6360=CARTESIAN_POINT ( 'NONE',  ( -336.3521761649654422, -181.4155151828941825, -11.56382487286496463 ) ) ;
#6370=PLANE ( 'NONE',  #8995 ) ;
#6371=ORIENTED_EDGE ( 'NONE', *, *, #34209, .T. ) ;
#6373=CIRCLE ( 'NONE', #22305, 60.00000000000000000 ) ;
#6375=VERTEX_POINT ( 'NONE', #27720 ) ;
#6380=ADVANCED_FACE ( 'NONE', ( #47447 ), #3302, .F. ) ;
#6383=LINE ( 'NONE', #46329, #10384 ) ;
#6386=AXIS2_PLACEMENT_3D ( 'NONE', #38222, #36463, #9156 ) ;
#6387=EDGE_LOOP ( 'NONE', ( #20848, #51335, #38619, #29608 ) ) ;
#6390=VERTEX_POINT ( 'NONE', #39540 ) ;
#6391=ADVANCED_FACE ( 'NONE', ( #42976 ), #11427, .F. ) ;
#6394=VERTEX_POINT ( 'NONE', #11943 ) ;
#6395=FACE_BOUND ( 'NONE', #32784, .T. ) ;
#6400=CARTESIAN_POINT ( 'NONE',  ( -339.1964088526558498, -179.4217241332781043, 21.74306257088782601 ) ) ;
#6407=ORIENTED_EDGE ( 'NONE', *, *, #18495, .F. ) ;
#6410=DIRECTION ( 'NONE',  ( -0.000000000000000000, 0.7485107481710999711, -0.6631226582407964143 ) ) ;
#6411=DIRECTION ( 'NONE',  ( 0.000000000000000000, 0.000000000000000000, 1.000000000000000000 ) ) ;
#6419=DIRECTION ( 'NONE',  ( 0.000000000000000000, -1.110223024625156540E-13, 1.000000000000000000 ) ) ;
#6425=ORIENTED_EDGE ( 'NONE', *, *, #36160, .T. ) ;
#6426=FACE_OUTER_BOUND ( 'NONE', #5384, .T. ) ;
#6430=CARTESIAN_POINT ( 'NONE',  ( -336.3521761649654422, -169.4076645216271402, -37.15394033962039089 ) ) ;
#6431=EDGE_LOOP ( 'NONE', ( #28342, #25188, #51710, #37432 ) ) ;
#6433=ORIENTED_EDGE ( 'NONE', *, *, #34379, .T. ) ;
#6440=ORIENTED_EDGE ( 'NONE', *, *, #47267, .T. ) ;
#6449=EDGE_CURVE ( 'NONE', #44354, #30980, #4329, .T. ) ;
#6452=EDGE_CURVE ( 'NONE', #27857, #13909, #36914, .T. ) ;
#6462=AXIS2_PLACEMENT_3D ( 'NONE', #33727, #1675, #46095 ) ;
#6464=DIRECTION ( 'NONE',  ( 0.000000000000000000, -0.6631226582407989678, -0.7485107481710977506 ) ) ;
#6465=ORIENTED_EDGE ( 'NONE', *, *, #46499, .F. ) ;
#6469=ORIENTED_EDGE ( 'NONE', *, *, #11964, .F. ) ;
#6472=DIRECTION ( 'NONE',  ( -0.000000000000000000, 0.8854560256532157947, 0.4647231720437573488 ) ) ;
#6473=VERTEX_POINT ( 'NONE', #900 ) ;
#6480=ORIENTED_EDGE ( 'NONE', *, *, #26832, .F. ) ;
#6482=CONICAL_SURFACE ( 'NONE', #16570, 20.00000000000000355, 0.4363323129985833826 ) ;
#6483=LINE ( 'NONE', #11426, #18065 ) ;
#6497=VECTOR ( 'NONE', #40523, 1000.000000000000000 ) ;
#6501=ORIENTED_EDGE ( 'NONE', *, *, #14914, .T. ) ;
#6504=DIRECTION ( 'NONE',  ( 0.000000000000000000, -0.1205366802553130001, 0.9927088740980553050 ) ) ;
#6506=DIRECTION ( 'NONE',  ( -0.000000000000000000, 1.047444401652940007E-14, 1.000000000000000000 ) ) ;
#6507=DIRECTION ( 'NONE',  ( 1.000000000000000000, 0.000000000000000000, 0.000000000000000000 ) ) ;
#6508=CARTESIAN_POINT ( 'NONE',  ( 0.000000000000000000, -182.5000000000000568, 0.000000000000000000 ) ) ;
#6511=DIRECTION ( 'NONE',  ( -1.000000000000000000, 0.000000000000000000, 0.000000000000000000 ) ) ;
#6516=ORIENTED_EDGE ( 'NONE', *, *, #40377, .T. ) ;
#6522=LINE ( 'NONE', #22550, #6649 ) ;
#6527=DIRECTION ( 'NONE',  ( -1.000000000000000000, -0.000000000000000000, 0.000000000000000000 ) ) ;
#6530=AXIS2_PLACEMENT_3D ( 'NONE', #1591, #37840, #41513 ) ;
#6539=VECTOR ( 'NONE', #1338, 1000.000000000000000 ) ;
#6555=DIRECTION ( 'NONE',  ( 0.000000000000000000, -0.5680647467311569221, -0.8229838658936556861 ) ) ;
#6558=DIRECTION ( 'NONE',  ( 0.000000000000000000, -3.491481338843133355E-15, -1.000000000000000000 ) ) ;
#6565=CIRCLE ( 'NONE', #13270, 5.000000000000001776 ) ;
#6571=PLANE ( 'NONE',  #50800 ) ;
#6572=VERTEX_POINT ( 'NONE', #5124 ) ;
#6574=PLANE ( 'NONE',  #32307 ) ;
#6576=ADVANCED_FACE ( 'NONE', ( #21133 ), #12205, .T. ) ;
#6581=LINE ( 'NONE', #14208, #9085 ) ;
#6582=DIRECTION ( 'NONE',  ( -0.000000000000000000, 0.7485107481711089639, 0.6631226582407863113 ) ) ;
#6587=ORIENTED_EDGE ( 'NONE', *, *, #31167, .T. ) ;
#6588=DIRECTION ( 'NONE',  ( 0.000000000000000000, -0.9927088740980548609, -0.1205366802553164696 ) ) ;
#6591=ORIENTED_EDGE ( 'NONE', *, *, #11202, .F. ) ;
#6594=DIRECTION ( 'NONE',  ( 0.000000000000000000, 0.8229838658936575735, 0.5680647467311540355 ) ) ;
#6595=CARTESIAN_POINT ( 'NONE',  ( -336.3521761649654422, -77.59233547837267508, 37.15394033962009246 ) ) ;
#6598=AXIS2_PLACEMENT_3D ( 'NONE', #6872, #2921, #26576 ) ;
#6599=FACE_OUTER_BOUND ( 'NONE', #50697, .T. ) ;
#6600=ORIENTED_EDGE ( 'NONE', *, *, #45926, .F. ) ;
#6601=CARTESIAN_POINT ( 'NONE',  ( -305.0000000000000568, -168.0775241366797275, 40.16023333901010517 ) ) ;
#6603=DIRECTION ( 'NONE',  ( -0.000000000000000000, -0.8229838658936516893, 0.5680647467311626952 ) ) ;
#6609=LINE ( 'NONE', #18685, #40016 ) ;
#6610=ORIENTED_EDGE ( 'NONE', *, *, #16364, .T. ) ;
#6611=AXIS2_PLACEMENT_3D ( 'NONE', #19172, #35190, #31501 ) ;
#6622=AXIS2_PLACEMENT_3D ( 'NONE', #40552, #8762, #12179 ) ;
#6623=VERTEX_POINT ( 'NONE', #9324 ) ;
#6624=VECTOR ( 'NONE', #41449, 1000.000000000000000 ) ;
#6626=DIRECTION ( 'NONE',  ( -1.000000000000000000, 0.000000000000000000, 0.000000000000000000 ) ) ;
#6628=EDGE_CURVE ( 'NONE', #37305, #12850, #38461, .T. ) ;
#6629=LINE ( 'NONE', #26322, #42124 ) ;
#6634=DIRECTION ( 'NONE',  ( -8.718379230999707126E-17, 0.9709418174260511236, -0.2393156642875615969 ) ) ;
#6635=AXIS2_PLACEMENT_3D ( 'NONE', #25677, #37506, #5205 ) ;
#6637=CARTESIAN_POINT ( 'NONE',  ( -339.1964088526558498, -180.6659093959932250, 14.60509510167942437 ) ) ;
#6644=ORIENTED_EDGE ( 'NONE', *, *, #37671, .F. ) ;
#6649=VECTOR ( 'NONE', #17820, 1000.000000000000000 ) ;
#6650=EDGE_LOOP ( 'NONE', ( #1102, #22259, #12251, #45967 ) ) ;
#6651=CARTESIAN_POINT ( 'NONE',  ( -305.0000000000000568, -180.4803820837415458, -18.79457521708939183 ) ) ;
#6653=ORIENTED_EDGE ( 'NONE', *, *, #27363, .F. ) ;
#6655=CARTESIAN_POINT ( 'NONE',  ( -332.3517673607765914, -83.15397741537739762, 43.07972642080338233 ) ) ;
#6657=CARTESIAN_POINT ( 'NONE',  ( -330.4913330509368166, -102.6919536717973926, 56.27632902032055284 ) ) ;
#6658=FACE_OUTER_BOUND ( 'NONE', #36270, .T. ) ;
#6662=CIRCLE ( 'NONE', #4148, 60.00000000000000000 ) ;
#6663=DIRECTION ( 'NONE',  ( 1.000000000000000000, -0.000000000000000000, -0.000000000000000000 ) ) ;
#6665=ORIENTED_EDGE ( 'NONE', *, *, #16851, .F. ) ;
#6668=CARTESIAN_POINT ( 'NONE',  ( -336.3521761649654422, -172.9832938399466684, -32.17247266903247294 ) ) ;
#6671=CARTESIAN_POINT ( 'NONE',  ( -339.1964088526558498, -64.86990808808704401, 6.615309698014191220 ) ) ;
#6672=FACE_OUTER_BOUND ( 'NONE', #25158, .T. ) ;
#6675=EDGE_CURVE ( 'NONE', #19616, #44602, #25863, .T. ) ;
#6677=EDGE_CURVE ( 'NONE', #42477, #32555, #30564, .T. ) ;
#6679=CARTESIAN_POINT ( 'NONE',  ( -365.0000000000001137, -78.50000000000002842, 5.000000000000001776 ) ) ;
#6680=EDGE_CURVE ( 'NONE', #7888, #44388, #21670, .T. ) ;
#6681=AXIS2_PLACEMENT_3D ( 'NONE', #14222, #17897, #30241 ) ;
#6682=DIRECTION ( 'NONE',  ( 0.000000000000000000, 0.6631226582407885317, -0.7485107481711069655 ) ) ;
#6684=DIRECTION ( 'NONE',  ( 0.000000000000000000, -0.8854560256532062468, 0.4647231720437755564 ) ) ;
#6685=EDGE_CURVE ( 'NONE', #30451, #47556, #5907, .T. ) ;
#6691=DIRECTION ( 'NONE',  ( 0.000000000000000000, 0.000000000000000000, -1.000000000000000000 ) ) ;
#6692=DIRECTION ( 'NONE',  ( -1.000000000000000000, 4.850383327711829203E-15, -9.241633304753623405E-15 ) ) ;
#6694=ORIENTED_EDGE ( 'NONE', *, *, #39111, .F. ) ;
#6695=EDGE_CURVE ( 'NONE', #15290, #32906, #49539, .T. ) ;
#6696=VERTEX_POINT ( 'NONE', #30313 ) ;
#6709=PLANE ( 'NONE',  #2165 ) ;
#6710=CARTESIAN_POINT ( 'NONE',  ( -339.1964088526558498, -116.8846903019842927, 58.63009191191280678 ) ) ;
#6716=CARTESIAN_POINT ( 'NONE',  ( -339.1964088526558498, -79.00630452878414189, 38.74998146212082162 ) ) ;
#6717=EDGE_CURVE ( 'NONE', #38969, #18701, #1429, .T. ) ;
#6724=DIRECTION ( 'NONE',  ( 0.000000000000000000, 0.6631226582407937498, -0.7485107481711024136 ) ) ;
#6729=EDGE_CURVE ( 'NONE', #38762, #28636, #34511, .T. ) ;
#6731=CIRCLE ( 'NONE', #40271, 20.00000000000000355 ) ;
#6733=ORIENTED_EDGE ( 'NONE', *, *, #30691, .F. ) ;
#6735=ORIENTED_EDGE ( 'NONE', *, *, #24458, .T. ) ;
#6745=VERTEX_POINT ( 'NONE', #30839 ) ;
#6746=DIRECTION ( 'NONE',  ( 1.000000000000000000, -0.000000000000000000, -0.000000000000000000 ) ) ;
#6747=ADVANCED_FACE ( 'NONE', ( #19011 ), #22954, .F. ) ;
#6749=LINE ( 'NONE', #18819, #49221 ) ;
#6765=VERTEX_POINT ( 'NONE', #38962 ) ;
#6771=CARTESIAN_POINT ( 'NONE',  ( -305.0000000000000568, -75.66382151296542702, -36.21739951675945690 ) ) ;
#6772=DIRECTION ( 'NONE',  ( -1.000000000000000000, 5.928974370888993961E-15, 8.589602288500771593E-15 ) ) ;
#6777=EDGE_CURVE ( 'NONE', #49846, #16432, #29552, .T. ) ;
#6779=CARTESIAN_POINT ( 'NONE',  ( -336.3521761649654422, -75.87119766449505676, -34.85916744524372746 ) ) ;
#6784=LINE ( 'NONE', #14939, #2229 ) ;
#6788=LINE ( 'NONE', #14416, #37129 ) ;
#6789=ORIENTED_EDGE ( 'NONE', *, *, #8732, .F. ) ;
#6790=PLANE ( 'NONE',  #17960 ) ;
#6795=ORIENTED_EDGE ( 'NONE', *, *, #19823, .F. ) ;
#6797=PLANE ( 'NONE',  #6816 ) ;
#6799=EDGE_CURVE ( 'NONE', #32390, #16904, #11108, .T. ) ;
#6804=VECTOR ( 'NONE', #4604, 999.9999999999998863 ) ;
#6807=DIRECTION ( 'NONE',  ( 0.000000000000000000, 0.9709418174260519008, -0.2393156642875582940 ) ) ;
#6808=VERTEX_POINT ( 'NONE', #10604 ) ;
#6816=AXIS2_PLACEMENT_3D ( 'NONE', #7814, #51461, #19643 ) ;
#6817=FACE_OUTER_BOUND ( 'NONE', #10091, .T. ) ;
#6818=CARTESIAN_POINT ( 'NONE',  ( -330.4913330509368166, -116.8846903019851311, -58.63009191191288494 ) ) ;
#6823=LINE ( 'NONE', #47292, #28104 ) ;
#6826=ORIENTED_EDGE ( 'NONE', *, *, #32291, .T. ) ;
#6831=VERTEX_POINT ( 'NONE', #51097 ) ;
#6835=LINE ( 'NONE', #43086, #50524 ) ;
#6837=EDGE_LOOP ( 'NONE', ( #48083, #17771, #3605, #23755 ) ) ;
#6839=FACE_OUTER_BOUND ( 'NONE', #13987, .T. ) ;
#6845=PLANE ( 'NONE',  #23967 ) ;
#6852=LINE ( 'NONE', #43375, #21069 ) ;
#6857=VECTOR ( 'NONE', #4529, 1000.000000000000000 ) ;
#6861=CARTESIAN_POINT ( 'NONE',  ( -336.3521761649654422, -172.9832938399466684, -32.17247266903247294 ) ) ;
#6864=CARTESIAN_POINT ( 'NONE',  ( -339.1964088526558498, -163.6602333390095509, 44.57752413668022484 ) ) ;
#6865=AXIS2_PLACEMENT_3D ( 'NONE', #35287, #31340, #10864 ) ;
#6868=ORIENTED_EDGE ( 'NONE', *, *, #40757, .F. ) ;
#6869=VECTOR ( 'NONE', #42483, 1000.000000000000000 ) ;
#6872=CARTESIAN_POINT ( 'NONE',  ( -330.4913330509368166, -74.65991953890832633, 33.10432812419081472 ) ) ;
#6876=DIRECTION ( 'NONE',  ( 1.000000000000000000, -0.000000000000000000, -0.000000000000000000 ) ) ;
#6877=DIRECTION ( 'NONE',  ( 0.000000000000000000, 0.9709418174260519008, -0.2393156642875582940 ) ) ;
#6879=DIRECTION ( 'NONE',  ( 0.000000000000000000, 0.000000000000000000, -1.000000000000000000 ) ) ;
#6880=ORIENTED_EDGE ( 'NONE', *, *, #37885, .T. ) ;
#6883=CARTESIAN_POINT ( 'NONE',  ( -332.3517673607765914, -73.44864141332200802, 31.34948880313848107 ) ) ;
#6888=CIRCLE ( 'NONE', #15293, 60.00000000000000000 ) ;
#6890=ORIENTED_EDGE ( 'NONE', *, *, #25671, .F. ) ;
#6893=CARTESIAN_POINT ( 'NONE',  ( -330.4913330509368166, -137.1341532842531876, -57.40522506028080585 ) ) ;
#6898=ADVANCED_FACE ( 'NONE', ( #22695 ), #14824, .F. ) ;
#6900=FACE_BOUND ( 'NONE', #14466, .T. ) ;
#6901=VECTOR ( 'NONE', #2201, 1000.000000000000000 ) ;
#6903=ADVANCED_FACE ( 'NONE', ( #15086 ), #45006, .F. ) ;
#6906=ORIENTED_EDGE ( 'NONE', *, *, #27962, .T. ) ;
#6907=AXIS2_PLACEMENT_3D ( 'NONE', #45284, #27988, #44023 ) ;
#6908=CIRCLE ( 'NONE', #31238, 60.00000000000000000 ) ;
#6909=DIRECTION ( 'NONE',  ( 0.000000000000000000, 0.000000000000000000, 1.000000000000000000 ) ) ;
#6910=DIRECTION ( 'NONE',  ( 0.000000000000000000, -0.1205366802553130001, 0.9927088740980551940 ) ) ;
#6915=ADVANCED_FACE ( 'NONE', ( #23970 ), #25034, .F. ) ;
#6916=EDGE_CURVE ( 'NONE', #18084, #12833, #32118, .T. ) ;
#6920=DIRECTION ( 'NONE',  ( -1.000000000000000000, 0.000000000000000000, -0.000000000000000000 ) ) ;
#6922=CARTESIAN_POINT ( 'NONE',  ( -336.3521761649654422, -180.1556192733800117, 16.67542351306693149 ) ) ;
#6924=VECTOR ( 'NONE', #26991, 1000.000000000000114 ) ;
#6930=ORIENTED_EDGE ( 'NONE', *, *, #17989, .F. ) ;
#6932=ORIENTED_EDGE ( 'NONE', *, *, #46192, .F. ) ;
#6938=VECTOR ( 'NONE', #5261, 999.9999999999998863 ) ;
#6942=CARTESIAN_POINT ( 'NONE',  ( -339.1964088526558498, -123.5000000000000284, 0.000000000000000000 ) ) ;
#6944=VECTOR ( 'NONE', #41995, 1000.000000000000114 ) ;
#6945=CARTESIAN_POINT ( 'NONE',  ( -330.4913330509368166, -162.2499814621210419, 44.49369547121568758 ) ) ;
#6946=VECTOR ( 'NONE', #46880, 1000.000000000000000 ) ;
#6950=VECTOR ( 'NONE', #43305, 999.9999999999998863 ) ;
#6958=CARTESIAN_POINT ( 'NONE',  ( -336.3521761649654422, -181.8730728925770563, 8.732051761644092025 ) ) ;
#6965=CARTESIAN_POINT ( 'NONE',  ( -305.0000000000000568, -108.6560878169904640, -58.13482838284724608 ) ) ;
#6966=VECTOR ( 'NONE', #37429, 999.9999999999998863 ) ;
#6967=ORIENTED_EDGE ( 'NONE', *, *, #17013, .F. ) ;
#6969=DIRECTION ( 'NONE',  ( -1.000000000000000000, -0.000000000000000000, -0.000000000000000000 ) ) ;
#6975=EDGE_CURVE ( 'NONE', #42318, #21717, #48423, .T. ) ;
#6977=CARTESIAN_POINT ( 'NONE',  ( -339.1964088526558498, -66.09477493971894546, 13.63415328425207917 ) ) ;
#6980=LINE ( 'NONE', #2519, #50493 ) ;
#6982=VECTOR ( 'NONE', #17669, 1000.000000000000000 ) ;
#6990=VECTOR ( 'NONE', #15144, 1000.000000000000000 ) ;
#6991=VERTEX_POINT ( 'NONE', #316 ) ;
#6996=ORIENTED_EDGE ( 'NONE', *, *, #47394, .T. ) ;
#7000=DIRECTION ( 'NONE',  ( -0.000000000000000000, 0.2393156642875547968, -0.9709418174260527890 ) ) ;
#7001=ORIENTED_EDGE ( 'NONE', *, *, #46337, .F. ) ;
#7002=ORIENTED_EDGE ( 'NONE', *, *, #38834, .F. ) ;
#7004=EDGE_LOOP ( 'NONE', ( #31399, #9392, #35994, #17993 ) ) ;
#7005=DIRECTION ( 'NONE',  ( 0.000000000000000000, 0.000000000000000000, 1.000000000000000000 ) ) ;
#7006=EDGE_CURVE ( 'NONE', #40482, #41226, #48942, .T. ) ;
#7013=DIRECTION ( 'NONE',  ( -0.000000000000000000, 0.5680647467311656929, 0.8229838658936495799 ) ) ;
#7015=ORIENTED_EDGE ( 'NONE', *, *, #2157, .F. ) ;
#7018=VERTEX_POINT ( 'NONE', #24247 ) ;
#7027=ORIENTED_EDGE ( 'NONE', *, *, #23771, .T. ) ;
#7028=DIRECTION ( 'NONE',  ( -8.718379230999707126E-17, 0.4647231720437631775, -0.8854560256532126861 ) ) ;
#7030=EDGE_CURVE ( 'NONE', #8616, #13126, #5582, .T. ) ;
#7032=CARTESIAN_POINT ( 'NONE',  ( -330.4913330509368166, -178.4886558749184076, -21.38919645685194837 ) ) ;
#7034=ADVANCED_FACE ( 'NONE', ( #9511 ), #37360, .F. ) ;
#7037=ORIENTED_EDGE ( 'NONE', *, *, #10062, .F. ) ;
#7047=AXIS2_PLACEMENT_3D ( 'NONE', #14604, #11160, #10391 ) ;
#7048=EDGE_CURVE ( 'NONE', #19062, #16981, #41295, .T. ) ;
#7052=LINE ( 'NONE', #43300, #32304 ) ;
#7053=FACE_OUTER_BOUND ( 'NONE', #9680, .T. ) ;
#7055=ORIENTED_EDGE ( 'NONE', *, *, #27386, .F. ) ;
#7057=VECTOR ( 'NONE', #22253, 1000.000000000000227 ) ;
#7060=CARTESIAN_POINT ( 'NONE',  ( -336.3521761649654422, -98.41210887299327226, -53.46519113769058151 ) ) ;
#7063=CARTESIAN_POINT ( 'NONE',  ( -330.0000000000000568, -123.5000000000000284, -60.00000000000000000 ) ) ;
#7064=EDGE_CURVE ( 'NONE', #42669, #42461, #49204, .T. ) ;
#7065=EDGE_LOOP ( 'NONE', ( #18910, #14599, #39610, #48035 ) ) ;
#7072=AXIS2_PLACEMENT_3D ( 'NONE', #28078, #3401, #15501 ) ;
#7074=DIRECTION ( 'NONE',  ( -1.000000000000000000, 0.000000000000000000, 0.000000000000000000 ) ) ;
#7077=DIRECTION ( 'NONE',  ( -8.718379230999705894E-17, 0.3546048870425300148, -0.9350162426854169428 ) ) ;
#7078=ORIENTED_EDGE ( 'NONE', *, *, #37052, .F. ) ;
#7084=EDGE_CURVE ( 'NONE', #76, #47574, #25532, .T. ) ;
#7085=FACE_OUTER_BOUND ( 'NONE', #31288, .T. ) ;
#7088=CARTESIAN_POINT ( 'NONE',  ( -305.0000000000000568, -176.3931552210900691, 28.32515014536862807 ) ) ;
#7094=ORIENTED_EDGE ( 'NONE', *, *, #32043, .T. ) ;
#7096=DIRECTION ( 'NONE',  ( 0.000000000000000000, -0.3546048870425426158, -0.9350162426854120579 ) ) ;
#7099=DIRECTION ( 'NONE',  ( 0.000000000000000000, -0.8854560256532126861, -0.4647231720437631775 ) ) ;
#7100=LINE ( 'NONE', #42833, #13158 ) ;
#7101=CARTESIAN_POINT ( 'NONE',  ( -339.1964088526558498, -138.1050951016792681, -57.16590939599323917 ) ) ;
#7103=CARTESIAN_POINT ( 'NONE',  ( -336.3521761649654422, -161.2787550547969033, 46.61293454085098631 ) ) ;
#7104=DIRECTION ( 'NONE',  ( 0.000000000000000000, -0.4647231720437573488, 0.8854560256532157947 ) ) ;
#7107=CARTESIAN_POINT ( 'NONE',  ( -332.3517673607765914, -176.9651911376907094, -25.08789112700655721 ) ) ;
#7108=LINE ( 'NONE', #22629, #19379 ) ;
#7109=AXIS2_PLACEMENT_3D ( 'NONE', #36030, #29, #44177 ) ;
#7114=ORIENTED_EDGE ( 'NONE', *, *, #50340, .F. ) ;
#7119=CARTESIAN_POINT ( 'NONE',  ( -332.3517673607765914, -87.81784868886214213, 47.06073758877343494 ) ) ;
#7124=DIRECTION ( 'NONE',  ( -1.000000000000000000, -0.000000000000000000, -0.000000000000000000 ) ) ;
#7128=CARTESIAN_POINT ( 'NONE',  ( 0.000000000000000000, -64.93017642821482127, -7.111664135064078351 ) ) ;
#7131=DIRECTION ( 'NONE',  ( 1.000000000000000000, 0.000000000000000000, 0.000000000000000000 ) ) ;
#7132=CARTESIAN_POINT ( 'NONE',  ( -332.3517673607765914, -106.8245764869328980, 56.65561927337994064 ) ) ;
#7141=ORIENTED_EDGE ( 'NONE', *, *, #41980, .F. ) ;
#7145=LINE ( 'NONE', #19241, #45631 ) ;
#7148=FACE_OUTER_BOUND ( 'NONE', #15957, .T. ) ;
#7151=LINE ( 'NONE', #39210, #1553 ) ;
#7156=CARTESIAN_POINT ( 'NONE',  ( -339.1964088526558498, -180.9052250602807703, 13.63415328425337236 ) ) ;
#7157=ORIENTED_EDGE ( 'NONE', *, *, #50884, .F. ) ;
#7158=FACE_BOUND ( 'NONE', #45802, .T. ) ;
#7164=ORIENTED_EDGE ( 'NONE', *, *, #25715, .T. ) ;
#7166=FACE_OUTER_BOUND ( 'NONE', #48284, .T. ) ;
#7168=ORIENTED_EDGE ( 'NONE', *, *, #43198, .F. ) ;
#7173=DIRECTION ( 'NONE',  ( -1.000000000000000000, 0.000000000000000000, 0.000000000000000000 ) ) ;
#7176=CARTESIAN_POINT ( 'NONE',  ( -330.4913330509368166, -123.5000000000000284, 0.000000000000000000 ) ) ;
#7177=DIRECTION ( 'NONE',  ( 1.000000000000000000, -6.525800561035029935E-17, -5.781354811211807281E-17 ) ) ;
#7178=VERTEX_POINT ( 'NONE', #43635 ) ;
#7181=VERTEX_POINT ( 'NONE', #38649 ) ;
#7182=DIRECTION ( 'NONE',  ( 0.000000000000000000, 0.000000000000000000, 1.000000000000000000 ) ) ;
#7185=ORIENTED_EDGE ( 'NONE', *, *, #47029, .F. ) ;
#7195=VECTOR ( 'NONE', #12302, 1000.000000000000000 ) ;
#7197=ORIENTED_EDGE ( 'NONE', *, *, #39008, .F. ) ;
#7202=CARTESIAN_POINT ( 'NONE',  ( -330.4913330509368166, -123.9999999999993747, 59.00000000000002132 ) ) ;
#7204=CARTESIAN_POINT ( 'NONE',  ( -339.1964088526558498, -183.1207326066166559, 6.735595255827131922 ) ) ;
#7206=DIRECTION ( 'NONE',  ( -1.000000000000000000, 0.000000000000000000, 0.000000000000000000 ) ) ;
#7208=EDGE_CURVE ( 'NONE', #37674, #13133, #14500, .T. ) ;
#7213=VERTEX_POINT ( 'NONE', #18694 ) ;
#7215=VECTOR ( 'NONE', #20032, 1000.000000000000114 ) ;
#7217=CARTESIAN_POINT ( 'NONE',  ( -336.3521761649654422, -118.0087234915157381, -58.76657425099333665 ) ) ;
#7218=ORIENTED_EDGE ( 'NONE', *, *, #45451, .F. ) ;
#7219=DIRECTION ( 'NONE',  ( -0.000000000000000000, 0.000000000000000000, -1.000000000000000000 ) ) ;
#7223=EDGE_LOOP ( 'NONE', ( #13047, #6610, #42610, #48108 ) ) ;
#7228=CARTESIAN_POINT ( 'NONE',  ( -336.3521761649654422, -67.40061919120938683, 18.46045550523129819 ) ) ;
#7229=ADVANCED_FACE ( 'NONE', ( #7633 ), #30505, .F. ) ;
#7230=ORIENTED_EDGE ( 'NONE', *, *, #11124, .F. ) ;
#7231=VECTOR ( 'NONE', #24546, 1000.000000000000000 ) ;
#7237=DIRECTION ( 'NONE',  ( 0.000000000000000000, 0.5680647467311485954, -0.8229838658936613482 ) ) ;
#7241=DIRECTION ( 'NONE',  ( 0.000000000000000000, 0.000000000000000000, -1.000000000000000000 ) ) ;
#7248=FACE_OUTER_BOUND ( 'NONE', #43339, .T. ) ;
#7253=LINE ( 'NONE', #23293, #27104 ) ;
#7256=VECTOR ( 'NONE', #7013, 1000.000000000000114 ) ;
#7260=DIRECTION ( 'NONE',  ( -1.000000000000000000, 0.000000000000000000, 0.000000000000000000 ) ) ;
#7263=EDGE_LOOP ( 'NONE', ( #403, #2990, #50450, #1494 ) ) ;
#7266=AXIS2_PLACEMENT_3D ( 'NONE', #4056, #36890, #20327 ) ;
#7267=VECTOR ( 'NONE', #51834, 1000.000000000000000 ) ;
#7270=CIRCLE ( 'NONE', #32434, 60.00000000000000000 ) ;
#7271=DIRECTION ( 'NONE',  ( 0.000000000000000000, 0.5680647467311510379, -0.8229838658936596829 ) ) ;
#7272=ORIENTED_EDGE ( 'NONE', *, *, #26945, .T. ) ;
#7275=EDGE_CURVE ( 'NONE', #15941, #32812, #34455, .T. ) ;
#7281=ORIENTED_EDGE ( 'NONE', *, *, #37473, .T. ) ;
#7285=EDGE_CURVE ( 'NONE', #19813, #46894, #47595, .T. ) ;
#7286=CARTESIAN_POINT ( 'NONE',  ( -339.1964088526558498, -137.1341532842531876, -57.40522506028080585 ) ) ;
#7287=ORIENTED_EDGE ( 'NONE', *, *, #30693, .T. ) ;
#7289=ORIENTED_EDGE ( 'NONE', *, *, #46256, .F. ) ;
#7296=DIRECTION ( 'NONE',  ( 1.000000000000000000, -8.654812430365586465E-17, -1.050884489711573024E-17 ) ) ;
#7298=FACE_OUTER_BOUND ( 'NONE', #27077, .T. ) ;
#7302=ORIENTED_EDGE ( 'NONE', *, *, #18717, .T. ) ;
#7304=PLANE ( 'NONE',  #17322 ) ;
#7307=VECTOR ( 'NONE', #2688, 999.9999999999998863 ) ;
#7311=VECTOR ( 'NONE', #30820, 1000.000000000000000 ) ;
#7313=ORIENTED_EDGE ( 'NONE', *, *, #21739, .T. ) ;
#7333=VERTEX_POINT ( 'NONE', #15802 ) ;
#7336=CIRCLE ( 'NONE', #1481, 60.00000000000000000 ) ;
#7338=EDGE_CURVE ( 'NONE', #20222, #50025, #32583, .T. ) ;
#7339=FACE_OUTER_BOUND ( 'NONE', #35181, .T. ) ;
#7341=ORIENTED_EDGE ( 'NONE', *, *, #44171, .F. ) ;
#7342=DIRECTION ( 'NONE',  ( 1.000000000000000000, -0.000000000000000000, -0.000000000000000000 ) ) ;
#7344=ORIENTED_EDGE ( 'NONE', *, *, #559, .T. ) ;
#7350=ORIENTED_EDGE ( 'NONE', *, *, #37180, .T. ) ;
#7351=FACE_OUTER_BOUND ( 'NONE', #23757, .T. ) ;
#7353=EDGE_CURVE ( 'NONE', #12905, #30781, #4216, .T. ) ;
#7357=DIRECTION ( 'NONE',  ( 0.000000000000000000, -0.4647231720437631775, 0.8854560256532126861 ) ) ;
#7358=DIRECTION ( 'NONE',  ( -0.000000000000000000, -0.6631226582407964143, -0.7485107481710999711 ) ) ;
#7359=ORIENTED_EDGE ( 'NONE', *, *, #44731, .T. ) ;
#7360=EDGE_CURVE ( 'NONE', #3383, #14589, #6091, .T. ) ;
#7361=VECTOR ( 'NONE', #46321, 1000.000000000000227 ) ;
#7362=DIRECTION ( 'NONE',  ( -0.000000000000000000, -0.8229838658936596829, -0.5680647467311510379 ) ) ;
#7365=FACE_OUTER_BOUND ( 'NONE', #37162, .T. ) ;
#7367=CARTESIAN_POINT ( 'NONE',  ( -339.1964088526558498, -182.0095552316575152, 7.608018572113563138 ) ) ;
#7377=AXIS2_PLACEMENT_3D ( 'NONE', #45813, #28719, #13235 ) ;
#7382=CARTESIAN_POINT ( 'NONE',  ( -330.4913330509368166, -64.50000000000000000, 0.4999999999999551470 ) ) ;
#7384=VERTEX_POINT ( 'NONE', #12071 ) ;
#7388=DIRECTION ( 'NONE',  ( 0.000000000000000000, -1.350771346627273875E-13, 1.000000000000000000 ) ) ;
#7389=CARTESIAN_POINT ( 'NONE',  ( -332.3517673607765914, -91.32752733096738496, -49.48329383994654052 ) ) ;
#7390=DIRECTION ( 'NONE',  ( -1.000000000000000000, -0.000000000000000000, 0.000000000000000000 ) ) ;
#7399=ORIENTED_EDGE ( 'NONE', *, *, #32888, .F. ) ;
#7401=ORIENTED_EDGE ( 'NONE', *, *, #51445, .T. ) ;
#7402=CARTESIAN_POINT ( 'NONE',  ( -332.3517673607765914, -136.0347666902908372, 57.67619951860663718 ) ) ;
#7403=CARTESIAN_POINT ( 'NONE',  ( -330.4913330509368166, -89.82879061784626629, 49.66134974749640207 ) ) ;
#7404=ORIENTED_EDGE ( 'NONE', *, *, #22270, .T. ) ;
#7406=DIRECTION ( 'NONE',  ( 0.000000000000000000, 6.245004513516505540E-15, 1.000000000000000000 ) ) ;
#7408=PLANE ( 'NONE',  #30000 ) ;
#7409=ORIENTED_EDGE ( 'NONE', *, *, #44071, .F. ) ;
#7410=AXIS2_PLACEMENT_3D ( 'NONE', #39579, #7028, #42770 ) ;
#7411=EDGE_CURVE ( 'NONE', #7901, #33568, #41774, .T. ) ;
#7412=VECTOR ( 'NONE', #12084, 1000.000000000000000 ) ;
#7413=CARTESIAN_POINT ( 'NONE',  ( -332.3517673607765914, -181.1761995186066088, -12.53476669029101842 ) ) ;
#7414=ADVANCED_BREP_SHAPE_REPRESENTATION ( '', ( #2369, #31742 ), #3199 ) ;
#7415=ORIENTED_EDGE ( 'NONE', *, *, #6085, .F. ) ;
#7424=ORIENTED_EDGE ( 'NONE', *, *, #50605, .T. ) ;
#7425=ADVANCED_FACE ( 'NONE', ( #5793 ), #21019, .F. ) ;
#7436=ORIENTED_EDGE ( 'NONE', *, *, #46958, .T. ) ;
#7437=DIRECTION ( 'NONE',  ( 0.000000000000000000, 0.000000000000000000, 1.000000000000000000 ) ) ;
#7441=CARTESIAN_POINT ( 'NONE',  ( -330.4913330509368166, -182.5000000000000568, 0.4999999999999549249 ) ) ;
#7448=CARTESIAN_POINT ( 'NONE',  ( -336.3521761649654422, -135.2893155068536828, 58.83036664750492406 ) ) ;
#7457=ORIENTED_EDGE ( 'NONE', *, *, #41879, .F. ) ;
#7458=ORIENTED_EDGE ( 'NONE', *, *, #28375, .F. ) ;
#7461=DIRECTION ( 'NONE',  ( -8.718379230999707126E-17, 0.000000000000000000, 1.000000000000000000 ) ) ;
#7464=PLANE ( 'NONE',  #40038 ) ;
#7470=DIRECTION ( 'NONE',  ( 1.000000000000000000, -0.000000000000000000, -0.000000000000000000 ) ) ;
#7472=EDGE_CURVE ( 'NONE', #14905, #4633, #41493, .T. ) ;
#7475=ORIENTED_EDGE ( 'NONE', *, *, #29964, .F. ) ;
#7478=PLANE ( 'NONE',  #11423 ) ;
#7480=ORIENTED_EDGE ( 'NONE', *, *, #17258, .T. ) ;
#7484=CARTESIAN_POINT ( 'NONE',  ( -336.3521761649654422, -118.0087234915157381, -58.76657425099333665 ) ) ;
#7485=VECTOR ( 'NONE', #42011, 1000.000000000000000 ) ;
#7487=CARTESIAN_POINT ( 'NONE',  ( -339.1964088526558498, -108.8949048983204051, 57.16590939599314680 ) ) ;
#7489=PLANE ( 'NONE',  #3554 ) ;
#7491=EDGE_LOOP ( 'NONE', ( #3558, #36708, #51194, #12288 ) ) ;
#7496=ORIENTED_EDGE ( 'NONE', *, *, #10889, .F. ) ;
#7501=VECTOR ( 'NONE', #24021, 1000.000000000000000 ) ;
#7502=EDGE_CURVE ( 'NONE', #39834, #34082, #37572, .T. ) ;
#7507=DIRECTION ( 'NONE',  ( -0.000000000000000000, 0.8229838658936634577, 0.5680647467311457088 ) ) ;
#7508=ORIENTED_EDGE ( 'NONE', *, *, #10450, .T. ) ;
#7514=ORIENTED_EDGE ( 'NONE', *, *, #22895, .T. ) ;
#7517=CARTESIAN_POINT ( 'NONE',  ( -330.4913330509368166, -157.4273119900845757, 48.27201571436049932 ) ) ;
#7518=ORIENTED_EDGE ( 'NONE', *, *, #4188, .T. ) ;
#7519=DIRECTION ( 'NONE',  ( -0.000000000000000000, -0.8229838658936596829, -0.5680647467311510379 ) ) ;
#7522=PLANE ( 'NONE',  #12635 ) ;
#7528=CARTESIAN_POINT ( 'NONE',  ( -330.4913330509368166, -182.5000000000000568, 0.4999999999999549249 ) ) ;
#7532=CARTESIAN_POINT ( 'NONE',  ( -336.3521761649654422, -177.7325358280884586, 23.38292116578760726 ) ) ;
#7537=FACE_OUTER_BOUND ( 'NONE', #25242, .T. ) ;
#7541=CARTESIAN_POINT ( 'NONE',  ( -339.1964088526558498, -124.0000000000002700, -59.00000000000002132 ) ) ;
#7543=PLANE ( 'NONE',  #5797 ) ;
#7544=ORIENTED_EDGE ( 'NONE', *, *, #24257, .F. ) ;
#7545=LINE ( 'NONE', #31190, #17480 ) ;
#7550=AXIS2_PLACEMENT_3D ( 'NONE', #14188, #13918, #18634 ) ;
#7552=DIRECTION ( 'NONE',  ( 0.000000000000000000, 0.5680647467311540355, -0.8229838658936575735 ) ) ;
#7555=CARTESIAN_POINT ( 'NONE',  ( -336.3521761649654422, -123.5000000000000284, 0.000000000000000000 ) ) ;
#7558=DIRECTION ( 'NONE',  ( -1.000000000000000000, 0.000000000000000000, 0.000000000000000000 ) ) ;
#7559=DIRECTION ( 'NONE',  ( -0.000000000000000000, 0.9350162426854146114, -0.3546048870425363986 ) ) ;
#7561=ORIENTED_EDGE ( 'NONE', *, *, #31698, .F. ) ;
#7565=DIRECTION ( 'NONE',  ( 0.000000000000000000, -0.4647231720437604574, 0.8854560256532141294 ) ) ;
#7572=CARTESIAN_POINT ( 'NONE',  ( -330.4913330509368166, -163.6602333390095509, 44.57752413668021774 ) ) ;
#7575=PLANE ( 'NONE',  #30447 ) ;
#7577=ORIENTED_EDGE ( 'NONE', *, *, #31900, .F. ) ;
#7583=DIRECTION ( 'NONE',  ( 0.000000000000000000, -0.4647231720437604574, 0.8854560256532141294 ) ) ;
#7587=( LENGTH_UNIT ( ) NAMED_UNIT ( * ) SI_UNIT ( .MILLI., .METRE. ) );
#7591=ORIENTED_EDGE ( 'NONE', *, *, #9974, .F. ) ;
#7593=ORIENTED_EDGE ( 'NONE', *, *, #42921, .F. ) ;
#7594=DIRECTION ( 'NONE',  ( 0.000000000000000000, 0.1205366802553303057, 0.9927088740980530845 ) ) ;
#7595=EDGE_LOOP ( 'NONE', ( #21054, #22514, #45764, #46747 ) ) ;
#7598=ORIENTED_EDGE ( 'NONE', *, *, #46092, .F. ) ;
#7601=PLANE ( 'NONE',  #31566 ) ;
#7602=VERTEX_POINT ( 'NONE', #18630 ) ;
#7605=DIRECTION ( 'NONE',  ( -1.000000000000000000, 0.000000000000000000, 0.000000000000000000 ) ) ;
#7609=EDGE_CURVE ( 'NONE', #39961, #15284, #2597, .T. ) ;
#7615=DIRECTION ( 'NONE',  ( -1.000000000000000000, -0.000000000000000000, -0.000000000000000000 ) ) ;
#7617=CARTESIAN_POINT ( 'NONE',  ( -339.1964088526558498, -167.3305728129748786, -39.49849221029221269 ) ) ;
#7623=PLANE ( 'NONE',  #9022 ) ;
#7627=ORIENTED_EDGE ( 'NONE', *, *, #18153, .T. ) ;
#7632=CARTESIAN_POINT ( 'NONE',  ( -332.3517673607765914, -147.2170408776451609, -55.11353710303946940 ) ) ;
#7633=FACE_OUTER_BOUND ( 'NONE', #42194, .T. ) ;
#7636=ORIENTED_EDGE ( 'NONE', *, *, #5318, .F. ) ;
#7652=ORIENTED_EDGE ( 'NONE', *, *, #14279, .T. ) ;
#7656=CARTESIAN_POINT ( 'NONE',  ( -339.1964088526558498, -102.6919536717973784, 56.27632902032055284 ) ) ;
#7658=CARTESIAN_POINT ( 'NONE',  ( -332.3517673607765914, -66.51961791625839737, 18.79457521708899392 ) ) ;
#7661=DIRECTION ( 'NONE',  ( -1.000000000000000000, 0.000000000000000000, 0.000000000000000000 ) ) ;
#7663=ORIENTED_EDGE ( 'NONE', *, *, #32111, .F. ) ;
#7665=DIRECTION ( 'NONE',  ( -1.000000000000000000, -0.000000000000000000, 0.000000000000000000 ) ) ;
#7666=VECTOR ( 'NONE', #25148, 1000.000000000000000 ) ;
#7669=EDGE_CURVE ( 'NONE', #30653, #36591, #22828, .T. ) ;
#7674=FACE_OUTER_BOUND ( 'NONE', #141, .T. ) ;
#7676=AXIS2_PLACEMENT_3D ( 'NONE', #26636, #31082, #11106 ) ;
#7677=ORIENTED_EDGE ( 'NONE', *, *, #41308, .F. ) ;
#7678=CARTESIAN_POINT ( 'NONE',  ( -332.3517673607765914, -154.8494888031386836, 50.05135858667791382 ) ) ;
#7680=DIRECTION ( 'NONE',  ( -1.000000000000000000, -0.000000000000000000, -0.000000000000000000 ) ) ;
#7681=EDGE_CURVE ( 'NONE', #30840, #3547, #43311, .T. ) ;
#7682=LINE ( 'NONE', #2702, #3426 ) ;
#7686=EDGE_CURVE ( 'NONE', #45092, #41614, #42270, .T. ) ;
#7688=EDGE_CURVE ( 'NONE', #31493, #33271, #16772, .T. ) ;
#7692=DIRECTION ( 'NONE',  ( -1.000000000000000000, -0.000000000000000000, 0.000000000000000000 ) ) ;
#7695=ORIENTED_EDGE ( 'NONE', *, *, #2585, .T. ) ;
#7697=ORIENTED_EDGE ( 'NONE', *, *, #20787, .T. ) ;
#7702=ORIENTED_EDGE ( 'NONE', *, *, #12861, .F. ) ;
#7704=VERTEX_POINT ( 'NONE', #727 ) ;
#7707=VECTOR ( 'NONE', #12463, 1000.000000000000000 ) ;
#7708=DIRECTION ( 'NONE',  ( 0.000000000000000000, -0.9709418174260492362, 0.2393156642875685636 ) ) ;
#7709=CARTESIAN_POINT ( 'NONE',  ( -305.0000000000000568, -101.7569374291123268, 55.92172413327813274 ) ) ;
#7711=ORIENTED_EDGE ( 'NONE', *, *, #39866, .F. ) ;
#7713=CIRCLE ( 'NONE', #41282, 60.00000000000000000 ) ;
#7714=ORIENTED_EDGE ( 'NONE', *, *, #9588, .T. ) ;
#7715=EDGE_CURVE ( 'NONE', #8493, #18723, #3620, .T. ) ;
#7717=FACE_OUTER_BOUND ( 'NONE', #27801, .T. ) ;
#7723=PLANE ( 'NONE',  #16438 ) ;
#7726=ORIENTED_EDGE ( 'NONE', *, *, #51596, .F. ) ;
#7729=ORIENTED_EDGE ( 'NONE', *, *, #2352, .T. ) ;
#7733=ORIENTED_EDGE ( 'NONE', *, *, #7905, .F. ) ;
#7734=PLANE ( 'NONE',  #32428 ) ;
#7735=PLANE ( 'NONE',  #40495 ) ;
#7737=CARTESIAN_POINT ( 'NONE',  ( -330.4913330509368166, -138.3439121830100191, -58.13482838284712528 ) ) ;
#7745=CARTESIAN_POINT ( 'NONE',  ( -336.3521761649654422, -92.15051119686104641, -50.05135858667769355 ) ) ;
#7748=CARTESIAN_POINT ( 'NONE',  ( -336.3521761649654422, -171.3361784870343740, 36.21739951675978375 ) ) ;
#7751=EDGE_LOOP ( 'NONE', ( #26655, #25101, #16756, #872 ) ) ;
#7755=ORIENTED_EDGE ( 'NONE', *, *, #25028, .T. ) ;
#7757=CARTESIAN_POINT ( 'NONE',  ( -330.4913330509368166, -64.86990808808717190, -6.615309698015095385 ) ) ;
#7761=CARTESIAN_POINT ( 'NONE',  ( -339.1964088526558498, -75.22798428563991990, -33.92731199008514409 ) ) ;
#7762=VECTOR ( 'NONE', #13037, 1000.000000000000000 ) ;
#7763=CIRCLE ( 'NONE', #37131, 60.00000000000000000 ) ;
#7764=VERTEX_POINT ( 'NONE', #40142 ) ;
#7770=CARTESIAN_POINT ( 'NONE',  ( -330.4913330509368166, -66.33409060400670398, -14.60509510167892522 ) ) ;
#7771=FACE_OUTER_BOUND ( 'NONE', #190, .T. ) ;
#7784=VERTEX_POINT ( 'NONE', #4159 ) ;
#7785=DIRECTION ( 'NONE',  ( 0.000000000000000000, -0.4647231720437755564, -0.8854560256532062468 ) ) ;
#7787=VERTEX_POINT ( 'NONE', #32249 ) ;
#7788=DIRECTION ( 'NONE',  ( -0.000000000000000000, -0.4647231720437724478, -0.8854560256532078011 ) ) ;
#7790=CARTESIAN_POINT ( 'NONE',  ( 0.000000000000000000, -84.37576316379318087, -44.16213414209506283 ) ) ;
#7791=EDGE_CURVE ( 'NONE', #37919, #5531, #445, .T. ) ;
#7797=VECTOR ( 'NONE', #33033, 1000.000000000000000 ) ;
#7799=CARTESIAN_POINT ( 'NONE',  ( -336.3521761649654422, -93.75055682584159911, 51.01861988938794923 ) ) ;
#7805=DIRECTION ( 'NONE',  ( -0.000000000000000000, 0.9350162426854146114, -0.3546048870425363986 ) ) ;
#7808=CARTESIAN_POINT ( 'NONE',  ( -330.4913330509368166, -123.5000000000000284, 0.000000000000000000 ) ) ;
#7810=VERTEX_POINT ( 'NONE', #48570 ) ;
#7812=DIRECTION ( 'NONE',  ( 0.000000000000000000, -0.1205366802553268363, -0.9927088740980534176 ) ) ;
#7813=AXIS2_PLACEMENT_3D ( 'NONE', #35332, #11154, #31910 ) ;
#7814=CARTESIAN_POINT ( 'NONE',  ( -339.1964088526558498, -167.3305728129742249, 39.49849221029288060 ) ) ;
#7819=EDGE_CURVE ( 'NONE', #13356, #5724, #36189, .T. ) ;
#7827=CARTESIAN_POINT ( 'NONE',  ( -339.1964088526558498, -89.57268800991437274, 48.27201571435973904 ) ) ;
#7828=AXIS2_PLACEMENT_3D ( 'NONE', #8055, #4124, #20138 ) ;
#7829=ORIENTED_EDGE ( 'NONE', *, *, #16681, .T. ) ;
#7834=ADVANCED_FACE ( 'NONE', ( #43574 ), #7575, .F. ) ;
#7835=DIRECTION ( 'NONE',  ( -0.000000000000000000, 0.5680647467311656929, 0.8229838658936495799 ) ) ;
#7838=DIRECTION ( 'NONE',  ( -0.000000000000000000, -0.7485107481711046340, -0.6631226582407911962 ) ) ;
#7839=CARTESIAN_POINT ( 'NONE',  ( -332.3517673607765914, -79.68838513426354098, -40.99441916720346768 ) ) ;
#7844=DIRECTION ( 'NONE',  ( -1.000000000000000000, 0.000000000000000000, -0.000000000000000000 ) ) ;
#7847=EDGE_CURVE ( 'NONE', #38856, #7810, #4939, .T. ) ;
#7848=CARTESIAN_POINT ( 'NONE',  ( -336.3521761649654422, -77.59233547837267508, 37.15394033962009246 ) ) ;
#7851=FACE_OUTER_BOUND ( 'NONE', #20598, .T. ) ;
#7852=EDGE_CURVE ( 'NONE', #18828, #30731, #13334, .T. ) ;
#7857=EDGE_CURVE ( 'NONE', #22679, #47261, #37168, .T. ) ;
#7860=DIRECTION ( 'NONE',  ( -1.000000000000000000, -0.000000000000000000, 0.000000000000000000 ) ) ;
#7861=CARTESIAN_POINT ( 'NONE',  ( -330.4913330509368166, -78.92247586332024412, -40.16023333900999859 ) ) ;
#7862=DIRECTION ( 'NONE',  ( 0.000000000000000000, -0.3546048870425267951, 0.9350162426854181641 ) ) ;
#7863=ORIENTED_EDGE ( 'NONE', *, *, #17738, .T. ) ;
#7866=PLANE ( 'NONE',  #50668 ) ;
#7868=LINE ( 'NONE', #40189, #48091 ) ;
#7869=ORIENTED_EDGE ( 'NONE', *, *, #24146, .T. ) ;
#7871=DIRECTION ( 'NONE',  ( 0.000000000000000000, -0.1205366802553303196, -0.9927088740980530845 ) ) ;
#7875=EDGE_LOOP ( 'NONE', ( #36761, #339, #6733, #36169 ) ) ;
#7878=LINE ( 'NONE', #23905, #18692 ) ;
#7882=AXIS2_PLACEMENT_3D ( 'NONE', #40897, #5179, #4920 ) ;
#7888=VERTEX_POINT ( 'NONE', #37240 ) ;
#7893=VECTOR ( 'NONE', #9862, 1000.000000000000000 ) ;
#7896=DIRECTION ( 'NONE',  ( 1.000000000000000000, -0.000000000000000000, 0.000000000000000000 ) ) ;
#7901=VERTEX_POINT ( 'NONE', #45400 ) ;
#7902=DIRECTION ( 'NONE',  ( 0.000000000000000000, 0.6631226582407964143, 0.7485107481710999711 ) ) ;
#7905=EDGE_CURVE ( 'NONE', #6134, #46591, #9391, .T. ) ;
#7909=ADVANCED_FACE ( 'NONE', ( #17547 ), #49597, .T. ) ;
#7911=FACE_OUTER_BOUND ( 'NONE', #11583, .T. ) ;
#7912=EDGE_CURVE ( 'NONE', #34872, #5675, #44867, .T. ) ;
#7924=ORIENTED_EDGE ( 'NONE', *, *, #5144, .T. ) ;
#7932=DIRECTION ( 'NONE',  ( -0.000000000000000000, 0.9709418174260519008, -0.2393156642875582940 ) ) ;
#7934=DIRECTION ( 'NONE',  ( 0.000000000000000000, 0.000000000000000000, 1.000000000000000000 ) ) ;
#7941=ADVANCED_FACE ( 'NONE', ( #25415 ), #9136, .F. ) ;
#7942=CARTESIAN_POINT ( 'NONE',  ( -332.3517673607765914, -67.99860710409808462, -22.79463504017392950 ) ) ;
#7945=VECTOR ( 'NONE', #44781, 1000.000000000000000 ) ;
#7946=VERTEX_POINT ( 'NONE', #13582 ) ;
#7947=DIRECTION ( 'NONE',  ( -1.000000000000000000, -0.000000000000000000, 0.000000000000000000 ) ) ;
#7950=VECTOR ( 'NONE', #21910, 1000.000000000000000 ) ;
#7955=DIRECTION ( 'NONE',  ( -0.000000000000000000, 0.6631226582407937498, -0.7485107481711024136 ) ) ;
#7956=ORIENTED_EDGE ( 'NONE', *, *, #32233, .T. ) ;
#7957=ORIENTED_EDGE ( 'NONE', *, *, #8033, .T. ) ;
#7963=DIRECTION ( 'NONE',  ( -0.000000000000000000, -0.3546048870425300148, 0.9350162426854169428 ) ) ;
#7967=VECTOR ( 'NONE', #8022, 1000.000000000000114 ) ;
#7971=DIRECTION ( 'NONE',  ( 0.000000000000000000, 0.000000000000000000, -1.000000000000000000 ) ) ;
#7972=EDGE_CURVE ( 'NONE', #44682, #8048, #38005, .T. ) ;
#7980=VERTEX_POINT ( 'NONE', #30131 ) ;
#7985=DIRECTION ( 'NONE',  ( 0.000000000000000000, 0.9927088740980530845, -0.1205366802553303057 ) ) ;
#7986=EDGE_CURVE ( 'NONE', #49622, #18571, #1951, .T. ) ;
#7991=ADVANCED_FACE ( 'NONE', ( #10153 ), #2534, .T. ) ;
#7992=ORIENTED_EDGE ( 'NONE', *, *, #38355, .F. ) ;
#7995=PLANE ( 'NONE',  #1096 ) ;
#7998=ORIENTED_EDGE ( 'NONE', *, *, #3766, .F. ) ;
#7999=AXIS2_PLACEMENT_3D ( 'NONE', #23504, #49876, #3524 ) ;
#8002=PLANE ( 'NONE',  #19661 ) ;
#8005=EDGE_CURVE ( 'NONE', #36071, #20840, #42468, .T. ) ;
#8021=ORIENTED_EDGE ( 'NONE', *, *, #18289, .T. ) ;
#8022=DIRECTION ( 'NONE',  ( -0.000000000000000000, -0.9350162426854121689, 0.3546048870425426158 ) ) ;
#8030=DIRECTION ( 'NONE',  ( 0.000000000000000000, 0.000000000000000000, 1.000000000000000000 ) ) ;
#8033=EDGE_CURVE ( 'NONE', #45363, #24508, #50122, .T. ) ;
#8037=DIRECTION ( 'NONE',  ( -0.000000000000000000, -3.491481338843133355E-15, -1.000000000000000000 ) ) ;
#8041=FACE_BOUND ( 'NONE', #11695, .T. ) ;
#8045=LINE ( 'NONE', #3328, #37530 ) ;
#8048=VERTEX_POINT ( 'NONE', #34576 ) ;
#8052=CIRCLE ( 'NONE', #499, 60.00000000000000000 ) ;
#8055=CARTESIAN_POINT ( 'NONE',  ( -330.4913330509368166, -123.5000000000000284, 0.000000000000000000 ) ) ;
#8059=VECTOR ( 'NONE', #8624, 1000.000000000000000 ) ;
#8061=EDGE_CURVE ( 'NONE', #51893, #21483, #26434, .T. ) ;
#8062=CIRCLE ( 'NONE', #38284, 60.00000000000000000 ) ;
#8063=EDGE_LOOP ( 'NONE', ( #11475, #25173, #11343, #44366 ) ) ;
#8067=DIRECTION ( 'NONE',  ( 0.000000000000000000, 5.504855830433067636E-14, -1.000000000000000000 ) ) ;
#8084=ORIENTED_EDGE ( 'NONE', *, *, #46852, .F. ) ;
#8092=EDGE_CURVE ( 'NONE', #41126, #35764, #14897, .T. ) ;
#8102=LINE ( 'NONE', #39372, #725 ) ;
#8104=ORIENTED_EDGE ( 'NONE', *, *, #7847, .F. ) ;
#8112=ORIENTED_EDGE ( 'NONE', *, *, #37938, .T. ) ;
#8114=VERTEX_POINT ( 'NONE', #10933 ) ;
#8115=VECTOR ( 'NONE', #45503, 1000.000000000000000 ) ;
#8122=ORIENTED_EDGE ( 'NONE', *, *, #48160, .F. ) ;
#8125=LINE ( 'NONE', #35198, #27348 ) ;
#8126=VECTOR ( 'NONE', #5832, 1000.000000000000000 ) ;
#8127=DIRECTION ( 'NONE',  ( 1.000000000000000000, -0.000000000000000000, -0.000000000000000000 ) ) ;
#8130=VECTOR ( 'NONE', #49750, 1000.000000000000000 ) ;
#8131=VECTOR ( 'NONE', #34496, 1000.000000000000000 ) ;
#8134=ADVANCED_FACE ( 'NONE', ( #2782 ), #50892, .F. ) ;
#8142=DIRECTION ( 'NONE',  ( -0.000000000000000000, 0.6631226582408039638, 0.7485107481710934207 ) ) ;
#8144=ORIENTED_EDGE ( 'NONE', *, *, #13664, .F. ) ;
#8145=ORIENTED_EDGE ( 'NONE', *, *, #28112, .T. ) ;
#8147=EDGE_CURVE ( 'NONE', #20203, #11822, #7253, .T. ) ;
#8158=ORIENTED_EDGE ( 'NONE', *, *, #45971, .T. ) ;
#8166=ORIENTED_EDGE ( 'NONE', *, *, #28881, .T. ) ;
#8169=CARTESIAN_POINT ( 'NONE',  ( -332.3517673607765914, -110.7312321683605916, -58.62557946887767457 ) ) ;
#8171=FACE_OUTER_BOUND ( 'NONE', #8887, .T. ) ;
#8174=DIRECTION ( 'NONE',  ( 0.000000000000000000, 0.5680647467311540355, -0.8229838658936575735 ) ) ;
#8177=ORIENTED_EDGE ( 'NONE', *, *, #42160, .F. ) ;
#8178=DIRECTION ( 'NONE',  ( 0.000000000000000000, -0.3546048870425235200, 0.9350162426854194964 ) ) ;
#8179=FACE_OUTER_BOUND ( 'NONE', #32810, .T. ) ;
#8182=ORIENTED_EDGE ( 'NONE', *, *, #3175, .F. ) ;
#8186=LINE ( 'NONE', #24221, #21135 ) ;
#8188=DIRECTION ( 'NONE',  ( 1.000000000000000000, 0.000000000000000000, -8.718379230999705894E-17 ) ) ;
#8191=FACE_OUTER_BOUND ( 'NONE', #7223, .T. ) ;
#8195=DIRECTION ( 'NONE',  ( -1.000000000000000000, 0.000000000000000000, 0.000000000000000000 ) ) ;
#8196=PLANE ( 'NONE',  #4662 ) ;
#8197=ORIENTED_EDGE ( 'NONE', *, *, #552, .F. ) ;
#8199=VERTEX_POINT ( 'NONE', #39550 ) ;
#8204=DIRECTION ( 'NONE',  ( 0.000000000000000000, 3.631354476378115974E-14, -1.000000000000000000 ) ) ;
#8214=EDGE_LOOP ( 'NONE', ( #49589, #25196, #2364, #21493 ) ) ;
#8216=EDGE_CURVE ( 'NONE', #37898, #47019, #17829, .T. ) ;
#8219=ORIENTED_EDGE ( 'NONE', *, *, #1810, .F. ) ;
#8221=VERTEX_POINT ( 'NONE', #49211 ) ;
#8222=ADVANCED_FACE ( 'NONE', ( #40320 ), #47974, .F. ) ;
#8223=VERTEX_POINT ( 'NONE', #47726 ) ;
#8227=DIRECTION ( 'NONE',  ( -1.000000000000000000, -0.000000000000000000, -0.000000000000000000 ) ) ;
#8233=DIRECTION ( 'NONE',  ( -1.000000000000000000, 3.701062773504947387E-15, 9.758900497077123602E-15 ) ) ;
#8234=FACE_OUTER_BOUND ( 'NONE', #3299, .T. ) ;
#8236=ORIENTED_EDGE ( 'NONE', *, *, #182, .T. ) ;
#8237=DIRECTION ( 'NONE',  ( 0.000000000000000000, 0.000000000000000000, 1.000000000000000000 ) ) ;
#8239=DIRECTION ( 'NONE',  ( 1.000000000000000000, 0.000000000000000000, -0.000000000000000000 ) ) ;
#8243=VERTEX_POINT ( 'NONE', #37105 ) ;
#8245=DIRECTION ( 'NONE',  ( 0.000000000000000000, 0.3546048870425331789, -0.9350162426854158326 ) ) ;
#8247=CARTESIAN_POINT ( 'NONE',  ( -339.1964088526558498, -68.51134412508150717, 21.38919645685156112 ) ) ;
#8250=CARTESIAN_POINT ( 'NONE',  ( -339.1964088526558498, -102.1108035431470427, 54.98865587491797413 ) ) ;
#8253=VERTEX_POINT ( 'NONE', #7517 ) ;
#8257=VECTOR ( 'NONE', #25075, 1000.000000000000000 ) ;
#8262=EDGE_CURVE ( 'NONE', #13126, #46591, #29557, .T. ) ;
#8263=PLANE ( 'NONE',  #33223 ) ;
#8265=CARTESIAN_POINT ( 'NONE',  ( -339.1964088526558498, -74.65991953890826949, 33.10432812419072945 ) ) ;
#8269=ADVANCED_FACE ( 'NONE', ( #27475 ), #51935, .F. ) ;
#8273=ORIENTED_EDGE ( 'NONE', *, *, #21739, .F. ) ;
#8274=CIRCLE ( 'NONE', #4948, 60.00000000000000000 ) ;
#8276=CARTESIAN_POINT ( 'NONE',  ( 0.000000000000000000, -64.93017642821470758, 7.111664135063263892 ) ) ;
#8280=ORIENTED_EDGE ( 'NONE', *, *, #1812, .T. ) ;
#8282=EDGE_CURVE ( 'NONE', #41229, #33330, #49986, .T. ) ;
#8283=EDGE_CURVE ( 'NONE', #36522, #43333, #33689, .T. ) ;
#8306=FACE_BOUND ( 'NONE', #41972, .T. ) ;
#8309=CIRCLE ( 'NONE', #41881, 60.00000000000000000 ) ;
#8311=VERTEX_POINT ( 'NONE', #46056 ) ;
#8315=ORIENTED_EDGE ( 'NONE', *, *, #17602, .F. ) ;
#8319=CARTESIAN_POINT ( 'NONE',  ( -339.1964088526558498, -64.99044476834235695, 7.608018572112245970 ) ) ;
#8320=ORIENTED_EDGE ( 'NONE', *, *, #23576, .T. ) ;
#8321=CARTESIAN_POINT ( 'NONE',  ( -339.1964088526558498, -178.8432607619609485, -20.45418021416653076 ) ) ;
#8322=ORIENTED_EDGE ( 'NONE', *, *, #37175, .F. ) ;
#8329=LINE ( 'NONE', #40359, #29790 ) ;
#8338=ADVANCED_FACE ( 'NONE', ( #42087 ), #45783, .F. ) ;
#8343=CARTESIAN_POINT ( 'NONE',  ( -339.1964088526558498, -84.00150778970767362, -43.83057281297470098 ) ) ;
#8346=ORIENTED_EDGE ( 'NONE', *, *, #8602, .T. ) ;
#8349=ORIENTED_EDGE ( 'NONE', *, *, #21076, .T. ) ;
#8350=CARTESIAN_POINT ( 'NONE',  ( -336.3521761649654422, -98.41210887299327226, -53.46519113769058151 ) ) ;
#8352=DIRECTION ( 'NONE',  ( 1.000000000000000000, -0.000000000000000000, 0.000000000000000000 ) ) ;
#8354=EDGE_CURVE ( 'NONE', #33846, #8674, #8544, .T. ) ;
#8357=EDGE_CURVE ( 'NONE', #7888, #36418, #48862, .T. ) ;
#8361=EDGE_LOOP ( 'NONE', ( #41452, #33683, #3468, #12954 ) ) ;
#8365=ADVANCED_FACE ( 'NONE', ( #21002 ), #36489, .F. ) ;
#8366=PLANE ( 'NONE',  #21705 ) ;
#8368=ORIENTED_EDGE ( 'NONE', *, *, #12540, .T. ) ;
#8372=VERTEX_POINT ( 'NONE', #40432 ) ;
#8376=VERTEX_POINT ( 'NONE', #37022 ) ;
#8380=LINE ( 'NONE', #12041, #43444 ) ;
#8383=ORIENTED_EDGE ( 'NONE', *, *, #30168, .T. ) ;
#8384=CARTESIAN_POINT ( 'NONE',  ( -330.4913330509368166, -68.51134412508180560, -21.38919645685231075 ) ) ;
#8394=DIRECTION ( 'NONE',  ( -0.000000000000000000, -0.9927088740980548609, -0.1205366802553164696 ) ) ;
#8395=CARTESIAN_POINT ( 'NONE',  ( -330.4913330509368166, -163.6602333390101762, -44.57752413667967772 ) ) ;
#8396=VECTOR ( 'NONE', #29876, 1000.000000000000000 ) ;
#8402=CARTESIAN_POINT ( 'NONE',  ( -339.1964088526558498, -79.66942718702553350, -39.49849221029258928 ) ) ;
#8403=EDGE_LOOP ( 'NONE', ( #32253, #28819, #30796, #20978 ) ) ;
#8407=VECTOR ( 'NONE', #2412, 1000.000000000000000 ) ;
#8409=EDGE_CURVE ( 'NONE', #11143, #8243, #21263, .T. ) ;
#8410=PLANE ( 'NONE',  #24550 ) ;
#8414=DIRECTION ( 'NONE',  ( 0.000000000000000000, -0.9927088740980556381, -0.1205366802553095307 ) ) ;
#8416=ORIENTED_EDGE ( 'NONE', *, *, #52012, .T. ) ;
#8423=CARTESIAN_POINT ( 'NONE',  ( -330.0000000000000568, -123.5000000000000142, 60.00000000000000000 ) ) ;
#8424=CARTESIAN_POINT ( 'NONE',  ( -305.0000000000000568, -109.6270296344155923, 58.37414404713457117 ) ) ;
#8433=CARTESIAN_POINT ( 'NONE',  ( -330.4913330509368166, -74.65991953890832633, 33.10432812419081472 ) ) ;
#8436=CARTESIAN_POINT ( 'NONE',  ( -332.3517673607765914, -127.9985676343858501, 58.88711093124869222 ) ) ;
#8438=DIRECTION ( 'NONE',  ( 1.000000000000000000, 0.000000000000000000, 0.000000000000000000 ) ) ;
#8439=VECTOR ( 'NONE', #28820, 1000.000000000000114 ) ;
#8440=ORIENTED_EDGE ( 'NONE', *, *, #14388, .F. ) ;
#8441=CARTESIAN_POINT ( 'NONE',  ( -305.0000000000000568, -121.8677111499054320, 59.97779283292990016 ) ) ;
#8442=CARTESIAN_POINT ( 'NONE',  ( -336.3521761649654422, -140.1754235130667610, -56.65561927338005432 ) ) ;
#8443=DIRECTION ( 'NONE',  ( -0.000000000000000000, -1.000000000000000000, -0.000000000000000000 ) ) ;
#8444=ORIENTED_EDGE ( 'NONE', *, *, #33334, .T. ) ;
#8449=CARTESIAN_POINT ( 'NONE',  ( -330.4913330509368166, -175.9742670995615015, -26.97593913775547136 ) ) ;
#8451=CARTESIAN_POINT ( 'NONE',  ( -330.4913330509368166, -123.5000000000000284, 0.000000000000000000 ) ) ;
#8454=FACE_OUTER_BOUND ( 'NONE', #38370, .T. ) ;
#8456=CARTESIAN_POINT ( 'NONE',  ( -336.3521761649654422, -70.03480886230919111, 25.08789112700620194 ) ) ;
#8462=DIRECTION ( 'NONE',  ( -1.000000000000000000, 0.000000000000000000, 0.000000000000000000 ) ) ;
#8464=EDGE_LOOP ( 'NONE', ( #42144, #44483, #15442, #32817 ) ) ;
#8467=ORIENTED_EDGE ( 'NONE', *, *, #10579, .F. ) ;
#8469=AXIS2_PLACEMENT_3D ( 'NONE', #11960, #44027, #24068 ) ;
#8473=LINE ( 'NONE', #24503, #6497 ) ;
#8474=VERTEX_POINT ( 'NONE', #21523 ) ;
#8476=ORIENTED_EDGE ( 'NONE', *, *, #4205, .T. ) ;
#8477=CARTESIAN_POINT ( 'NONE',  ( -332.3517673607765914, -180.1590281025188460, -19.74220186498920881 ) ) ;
#8481=CARTESIAN_POINT ( 'NONE',  ( -336.3521761649654422, -176.5004679656469477, -25.97334715265976612 ) ) ;
#8482=CARTESIAN_POINT ( 'NONE',  ( -336.3521761649654422, -174.9833430614318388, 28.86398714850502856 ) ) ;
#8487=CARTESIAN_POINT ( 'NONE',  ( -336.3521761649654422, -181.1761995186066088, -12.53476669029101842 ) ) ;
#8493=VERTEX_POINT ( 'NONE', #48614 ) ;
#8500=ORIENTED_EDGE ( 'NONE', *, *, #38496, .T. ) ;
#8505=VERTEX_POINT ( 'NONE', #51566 ) ;
#8506=DIRECTION ( 'NONE',  ( -0.000000000000000000, 0.1205366802553337752, 0.9927088740980526405 ) ) ;
#8508=ADVANCED_FACE ( 'NONE', ( #47636 ), #8647, .T. ) ;
#8510=LINE ( 'NONE', #48485, #9406 ) ;
#8511=EDGE_LOOP ( 'NONE', ( #22811, #16900, #8084, #23193 ) ) ;
#8514=DIRECTION ( 'NONE',  ( -0.000000000000000000, 0.8854560256532157947, 0.4647231720437573488 ) ) ;
#8516=ORIENTED_EDGE ( 'NONE', *, *, #48741, .F. ) ;
#8519=ORIENTED_EDGE ( 'NONE', *, *, #35123, .T. ) ;
#8520=EDGE_CURVE ( 'NONE', #6745, #8999, #17335, .T. ) ;
#8542=PLANE ( 'NONE',  #13156 ) ;
#8544=CIRCLE ( 'NONE', #43810, 31.65769145387501027 ) ;
#8547=FACE_BOUND ( 'NONE', #29222, .T. ) ;
#8552=ORIENTED_EDGE ( 'NONE', *, *, #20947, .T. ) ;
#8554=EDGE_LOOP ( 'NONE', ( #30551, #31808, #22845, #20110 ) ) ;
#8555=ORIENTED_EDGE ( 'NONE', *, *, #48828, .T. ) ;
#8556=CARTESIAN_POINT ( 'NONE',  ( -336.3521761649654422, -153.2494431741581025, -51.01861988938816950 ) ) ;
#8559=PLANE ( 'NONE',  #13733 ) ;
#8560=DIRECTION ( 'NONE',  ( 0.000000000000000000, 7.100801428331730794E-14, -1.000000000000000000 ) ) ;
#8561=VERTEX_POINT ( 'NONE', #13895 ) ;
#8568=VERTEX_POINT ( 'NONE', #14166 ) ;
#8571=LINE ( 'NONE', #41155, #5180 ) ;
#8573=CARTESIAN_POINT ( 'NONE',  ( -336.3521761649654422, -171.1288023355047585, 34.85916744524404720 ) ) ;
#8576=DIRECTION ( 'NONE',  ( -0.000000000000000000, -0.8854560256532062468, 0.4647231720437755564 ) ) ;
#8577=EDGE_LOOP ( 'NONE', ( #6735, #37385, #18295, #43378 ) ) ;
#8578=DIRECTION ( 'NONE',  ( 1.000000000000000000, 0.000000000000000000, 0.000000000000000000 ) ) ;
#8581=AXIS2_PLACEMENT_3D ( 'NONE', #19314, #46927, #15895 ) ;
#8582=DIRECTION ( 'NONE',  ( 0.000000000000000000, -0.3546048870425426158, -0.9350162426854121689 ) ) ;
#8584=ORIENTED_EDGE ( 'NONE', *, *, #43952, .F. ) ;
#8587=PLANE ( 'NONE',  #35682 ) ;
#8588=ORIENTED_EDGE ( 'NONE', *, *, #32596, .F. ) ;
#8589=DIRECTION ( 'NONE',  ( -1.000000000000000000, 0.000000000000000000, -0.000000000000000000 ) ) ;
#8591=EDGE_LOOP ( 'NONE', ( #28945, #35265, #25319, #6281 ) ) ;
#8592=ADVANCED_FACE ( 'NONE', ( #38578 ), #33602, .F. ) ;
#8594=DIRECTION ( 'NONE',  ( -0.000000000000000000, 0.5680647467311457088, -0.8229838658936633466 ) ) ;
#8596=VERTEX_POINT ( 'NONE', #30183 ) ;
#8602=EDGE_CURVE ( 'NONE', #23236, #9916, #30425, .T. ) ;
#8606=CARTESIAN_POINT ( 'NONE',  ( -332.3517673607765914, -165.2193480479701293, -43.12187378178659714 ) ) ;
#8608=ADVANCED_FACE ( 'NONE', ( #29914 ), #41752, .T. ) ;
#8616=VERTEX_POINT ( 'NONE', #10723 ) ;
#8617=LINE ( 'NONE', #37259, #18983 ) ;
#8618=FACE_OUTER_BOUND ( 'NONE', #44368, .T. ) ;
#8622=ORIENTED_EDGE ( 'NONE', *, *, #8262, .F. ) ;
#8623=EDGE_CURVE ( 'NONE', #2171, #32119, #6788, .T. ) ;
#8624=DIRECTION ( 'NONE',  ( 1.000000000000000000, -6.525800561034911606E-17, 5.781354811211940401E-17 ) ) ;
#8627=EDGE_LOOP ( 'NONE', ( #27453, #7714, #27817, #49298 ) ) ;
#8632=EDGE_CURVE ( 'NONE', #50991, #15872, #30678, .T. ) ;
#8633=CARTESIAN_POINT ( 'NONE',  ( -332.3517673607765914, -64.50000000000000000, -1.632288850093980725 ) ) ;
#8637=VERTEX_POINT ( 'NONE', #49641 ) ;
#8642=CARTESIAN_POINT ( 'NONE',  ( -339.1964088526558498, -74.65991953890876687, -33.10432812419148263 ) ) ;
#8647=PLANE ( 'NONE',  #16972 ) ;
#8651=VECTOR ( 'NONE', #46119, 1000.000000000000000 ) ;
#8655=DIRECTION ( 'NONE',  ( 0.000000000000000000, 0.9927088740980544168, 0.1205366802553199251 ) ) ;
#8656=FACE_OUTER_BOUND ( 'NONE', #46417, .T. ) ;
#8660=VECTOR ( 'NONE', #25786, 999.9999999999998863 ) ;
#8666=VECTOR ( 'NONE', #24241, 1000.000000000000000 ) ;
#8669=ORIENTED_EDGE ( 'NONE', *, *, #4236, .T. ) ;
#8674=VERTEX_POINT ( 'NONE', #27252 ) ;
#8675=ORIENTED_EDGE ( 'NONE', *, *, #3608, .F. ) ;
#8678=EDGE_CURVE ( 'NONE', #31178, #27045, #11226, .T. ) ;
#8684=FACE_OUTER_BOUND ( 'NONE', #32046, .T. ) ;
#8685=LINE ( 'NONE', #28641, #35895 ) ;
#8688=DIRECTION ( 'NONE',  ( 0.000000000000000000, 0.4647231720437724478, 0.8854560256532078011 ) ) ;
#8694=DIRECTION ( 'NONE',  ( 0.000000000000000000, 0.000000000000000000, 1.000000000000000000 ) ) ;
#8702=CARTESIAN_POINT ( 'NONE',  ( -330.4913330509368166, -180.6659093959934523, -14.60509510167853442 ) ) ;
#8703=EDGE_LOOP ( 'NONE', ( #46703, #49008, #40519, #17814 ) ) ;
#8704=CARTESIAN_POINT ( 'NONE',  ( -330.4913330509368166, -63.99980407363864288, -7.728304129924675969 ) ) ;
#8705=CARTESIAN_POINT ( 'NONE',  ( -336.3521761649654422, -91.32752733096738496, -49.48329383994654052 ) ) ;
#8711=CARTESIAN_POINT ( 'NONE',  ( -305.0000000000000568, -63.50208336950359467, -0.4999999999996888600 ) ) ;
#8713=DIRECTION ( 'NONE',  ( -1.000000000000000000, 0.000000000000000000, -0.000000000000000000 ) ) ;
#8717=CARTESIAN_POINT ( 'NONE',  ( -332.3517673607765914, -127.9985676343858501, 58.88711093124869222 ) ) ;
#8719=DIRECTION ( 'NONE',  ( -1.000000000000000000, -2.497772389992548343E-15, -1.013386094502323194E-14 ) ) ;
#8720=LINE ( 'NONE', #29467, #44622 ) ;
#8721=DIRECTION ( 'NONE',  ( 0.000000000000000000, 0.000000000000000000, -1.000000000000000000 ) ) ;
#8723=ORIENTED_EDGE ( 'NONE', *, *, #37465, .T. ) ;
#8727=DIRECTION ( 'NONE',  ( 0.000000000000000000, 0.2393156642875582940, 0.9709418174260519008 ) ) ;
#8730=ORIENTED_EDGE ( 'NONE', *, *, #36352, .T. ) ;
#8732=EDGE_CURVE ( 'NONE', #5675, #16257, #24564, .T. ) ;
#8734=DIRECTION ( 'NONE',  ( -0.000000000000000000, 0.000000000000000000, -1.000000000000000000 ) ) ;
#8738=PLANE ( 'NONE',  #13462 ) ;
#8741=PLANE ( 'NONE',  #22847 ) ;
#8745=DIRECTION ( 'NONE',  ( 0.000000000000000000, 0.000000000000000000, -1.000000000000000000 ) ) ;
#8748=CARTESIAN_POINT ( 'NONE',  ( -339.1964088526558498, -66.09477493971917283, -13.63415328425296202 ) ) ;
#8750=LINE ( 'NONE', #24274, #46706 ) ;
#8757=ORIENTED_EDGE ( 'NONE', *, *, #40781, .F. ) ;
#8760=CARTESIAN_POINT ( 'NONE',  ( -332.3517673607765914, -152.3639871485048900, -51.48334306143194539 ) ) ;
#8762=DIRECTION ( 'NONE',  ( 0.000000000000000000, -0.3546048870425267951, 0.9350162426854181641 ) ) ;
#8768=DIRECTION ( 'NONE',  ( -0.000000000000000000, -0.2393156642875615969, -0.9709418174260511236 ) ) ;
#8772=DIRECTION ( 'NONE',  ( -0.000000000000000000, -0.4647231720437604574, 0.8854560256532141294 ) ) ;
#8773=LINE ( 'NONE', #20093, #40847 ) ;
#8774=EDGE_CURVE ( 'NONE', #10230, #1251, #44686, .T. ) ;
#8777=PLANE ( 'NONE',  #19404 ) ;
#8779=ORIENTED_EDGE ( 'NONE', *, *, #19478, .T. ) ;
#8781=LINE ( 'NONE', #37421, #40371 ) ;
#8785=CIRCLE ( 'NONE', #51597, 60.00000000000000000 ) ;
#8786=VERTEX_POINT ( 'NONE', #11743 ) ;
#8792=CARTESIAN_POINT ( 'NONE',  ( -332.3517673607765914, -119.0014323656137947, -58.88711093124865670 ) ) ;
#8793=ORIENTED_EDGE ( 'NONE', *, *, #18546, .F. ) ;
#8801=ORIENTED_EDGE ( 'NONE', *, *, #1912, .F. ) ;
#8804=DIRECTION ( 'NONE',  ( -8.718379230999708359E-17, -0.8229838658936495799, 0.5680647467311656929 ) ) ;
#8808=DIRECTION ( 'NONE',  ( 0.000000000000000000, 0.000000000000000000, -1.000000000000000000 ) ) ;
#8809=DIRECTION ( 'NONE',  ( 0.000000000000000000, 0.9350162426854121689, -0.3546048870425426158 ) ) ;
#8825=FACE_OUTER_BOUND ( 'NONE', #32151, .T. ) ;
#8829=VERTEX_POINT ( 'NONE', #33010 ) ;
#8832=CARTESIAN_POINT ( 'NONE',  ( -339.1964088526558498, -64.99044476834235695, 7.608018572112245970 ) ) ;
#8833=AXIS2_PLACEMENT_3D ( 'NONE', #46627, #6684, #22705 ) ;
#8840=CARTESIAN_POINT ( 'NONE',  ( -330.4913330509368166, -122.9999999999994600, 59.00000000000002132 ) ) ;
#8841=DIRECTION ( 'NONE',  ( -0.000000000000000000, -0.7485107481710977506, 0.6631226582407989678 ) ) ;
#8842=DIRECTION ( 'NONE',  ( 0.000000000000000000, 0.000000000000000000, -1.000000000000000000 ) ) ;
#8852=LINE ( 'NONE', #37489, #26300 ) ;
#8855=DIRECTION ( 'NONE',  ( 1.000000000000000000, 0.000000000000000000, 0.000000000000000000 ) ) ;
#8859=CIRCLE ( 'NONE', #38232, 60.00000000000000000 ) ;
#8861=CARTESIAN_POINT ( 'NONE',  ( -332.3517673607765914, -86.34605966037949543, -45.90766452162698386 ) ) ;
#8862=ORIENTED_EDGE ( 'NONE', *, *, #7852, .F. ) ;
#8867=CARTESIAN_POINT ( 'NONE',  ( -336.3521761649654422, -174.9833430614318388, 28.86398714850502856 ) ) ;
#8870=VERTEX_POINT ( 'NONE', #13312 ) ;
#8877=VECTOR ( 'NONE', #12820, 1000.000000000000114 ) ;
#8879=PLANE ( 'NONE',  #22572 ) ;
#8880=FACE_OUTER_BOUND ( 'NONE', #25041, .T. ) ;
#8882=DIRECTION ( 'NONE',  ( 0.000000000000000000, -0.4647231720437755564, -0.8854560256532062468 ) ) ;
#8885=VERTEX_POINT ( 'NONE', #49323 ) ;
#8887=EDGE_LOOP ( 'NONE', ( #42493, #10261, #3304, #5615 ) ) ;
#8888=ORIENTED_EDGE ( 'NONE', *, *, #22461, .T. ) ;
#8890=PLANE ( 'NONE',  #21688 ) ;
#8892=CARTESIAN_POINT ( 'NONE',  ( -339.1964088526558498, -168.0775241366801254, -40.16023333900967884 ) ) ;
#8893=ORIENTED_EDGE ( 'NONE', *, *, #19267, .T. ) ;
#8900=DIRECTION ( 'NONE',  ( 0.000000000000000000, -0.6631226582407863113, 0.7485107481711089639 ) ) ;
#8907=DIRECTION ( 'NONE',  ( 0.000000000000000000, -0.2393156642875615969, -0.9709418174260511236 ) ) ;
#8908=FACE_OUTER_BOUND ( 'NONE', #37803, .T. ) ;
#8922=EDGE_CURVE ( 'NONE', #22978, #49147, #40363, .T. ) ;
#8923=ORIENTED_EDGE ( 'NONE', *, *, #1027, .F. ) ;
#8924=AXIS2_PLACEMENT_3D ( 'NONE', #51249, #39134, #23622 ) ;
#8928=CARTESIAN_POINT ( 'NONE',  ( -305.0000000000000568, -123.5000000000000142, 60.00000000000000000 ) ) ;
#8931=CARTESIAN_POINT ( 'NONE',  ( -305.0000000000000568, -95.17484985463171654, -52.89315522109019696 ) ) ;
#8938=EDGE_CURVE ( 'NONE', #48723, #17876, #37217, .T. ) ;
#8944=EDGE_CURVE ( 'NONE', #16500, #23459, #24608, .T. ) ;
#8955=VECTOR ( 'NONE', #51504, 1000.000000000000114 ) ;
#8957=FACE_OUTER_BOUND ( 'NONE', #49271, .T. ) ;
#8961=DIRECTION ( 'NONE',  ( 1.000000000000000000, -0.000000000000000000, -0.000000000000000000 ) ) ;
#8963=DIRECTION ( 'NONE',  ( -0.000000000000000000, 0.3546048870425426158, 0.9350162426854120579 ) ) ;
#8964=DIRECTION ( 'NONE',  ( -0.000000000000000000, -0.8854560256532126861, -0.4647231720437631775 ) ) ;
#8965=CARTESIAN_POINT ( 'NONE',  ( -332.3517673607765914, -123.5000000000000284, 0.000000000000000000 ) ) ;
#8966=ADVANCED_FACE ( 'NONE', ( #45382 ), #13564, .F. ) ;
#8969=DIRECTION ( 'NONE',  ( -1.000000000000000000, 0.000000000000000000, 0.000000000000000000 ) ) ;
#8985=AXIS2_PLACEMENT_3D ( 'NONE', #30316, #46623, #7182 ) ;
#8987=CARTESIAN_POINT ( 'NONE',  ( -339.1964088526558498, -150.4759391377560576, -52.47426709956116042 ) ) ;
#8989=DIRECTION ( 'NONE',  ( -0.000000000000000000, 0.5680647467311540355, -0.8229838658936575735 ) ) ;
#8995=AXIS2_PLACEMENT_3D ( 'NONE', #21884, #38420, #46071 ) ;
#8999=VERTEX_POINT ( 'NONE', #37738 ) ;
#9003=DIRECTION ( 'NONE',  ( 1.000000000000000000, -0.000000000000000000, -0.000000000000000000 ) ) ;
#9006=CARTESIAN_POINT ( 'NONE',  ( -332.3517673607765914, -84.94915232962709695, -45.97643030831888922 ) ) ;
#9009=ADVANCED_FACE ( 'NONE', ( #5704 ), #45641, .F. ) ;
#9013=CARTESIAN_POINT ( 'NONE',  ( -330.4913330509368166, -137.1341532842531876, -57.40522506028080585 ) ) ;
#9022=AXIS2_PLACEMENT_3D ( 'NONE', #32042, #40441, #3672 ) ;
#9026=AXIS2_PLACEMENT_3D ( 'NONE', #9204, #17094, #40987 ) ;
#9029=CARTESIAN_POINT ( 'NONE',  ( -332.3517673607765914, -140.4009141470556870, -57.57047073799078873 ) ) ;
#9030=LINE ( 'NONE', #13484, #42532 ) ;
#9031=ORIENTED_EDGE ( 'NONE', *, *, #18683, .T. ) ;
#9032=AXIS2_PLACEMENT_3D ( 'NONE', #32661, #46428, #50627 ) ;
#9033=EDGE_LOOP ( 'NONE', ( #34418, #30140, #44134, #8555 ) ) ;
#9036=VECTOR ( 'NONE', #49163, 1000.000000000000000 ) ;
#9044=DIRECTION ( 'NONE',  ( 1.000000000000000000, -0.000000000000000000, -0.000000000000000000 ) ) ;
#9048=ORIENTED_EDGE ( 'NONE', *, *, #42671, .F. ) ;
#9051=ORIENTED_EDGE ( 'NONE', *, *, #47814, .F. ) ;
#9054=CARTESIAN_POINT ( 'NONE',  ( -336.3521761649654422, -142.8954717479169574, 55.74477592174805096 ) ) ;
#9058=EDGE_LOOP ( 'NONE', ( #8021, #51340, #7415, #29351 ) ) ;
#9060=ORIENTED_EDGE ( 'NONE', *, *, #16647, .F. ) ;
#9061=ORIENTED_EDGE ( 'NONE', *, *, #16681, .F. ) ;
#9062=VECTOR ( 'NONE', #14079, 1000.000000000000114 ) ;
#9063=AXIS2_PLACEMENT_3D ( 'NONE', #48857, #52030, #3924 ) ;
#9065=DIRECTION ( 'NONE',  ( 0.000000000000000000, -0.1205366802553303196, -0.9927088740980530845 ) ) ;
#9068=ORIENTED_EDGE ( 'NONE', *, *, #31996, .T. ) ;
#9069=CARTESIAN_POINT ( 'NONE',  ( -332.3517673607765914, -66.84438072661991725, -16.67542351306652648 ) ) ;
#9070=CARTESIAN_POINT ( 'NONE',  ( -305.0000000000000568, -183.4777928329299357, 1.632288850093980725 ) ) ;
#9071=DIRECTION ( 'NONE',  ( 0.000000000000000000, -0.2393156642875448881, 0.9709418174260553425 ) ) ;
#9072=AXIS2_PLACEMENT_3D ( 'NONE', #47976, #11958, #44025 ) ;
#9073=EDGE_LOOP ( 'NONE', ( #14394, #48890, #9761, #23314 ) ) ;
#9078=PLANE ( 'NONE',  #44286 ) ;
#9084=VERTEX_POINT ( 'NONE', #17531 ) ;
#9085=VECTOR ( 'NONE', #22332, 999.9999999999998863 ) ;
#9089=FACE_BOUND ( 'NONE', #14504, .T. ) ;
#9090=CARTESIAN_POINT ( 'NONE',  ( -330.4913330509368166, -78.92247586331968989, 40.16023333900940173 ) ) ;
#9094=ORIENTED_EDGE ( 'NONE', *, *, #17974, .T. ) ;
#9100=CARTESIAN_POINT ( 'NONE',  ( -336.3521761649654422, -123.5000000000000284, 0.000000000000000000 ) ) ;
#9102=LINE ( 'NONE', #41145, #43027 ) ;
#9105=ORIENTED_EDGE ( 'NONE', *, *, #27779, .T. ) ;
#9107=ORIENTED_EDGE ( 'NONE', *, *, #25133, .T. ) ;
#9111=AXIS2_PLACEMENT_3D ( 'NONE', #17363, #33383, #2357 ) ;
#9112=DIRECTION ( 'NONE',  ( 0.000000000000000000, -0.8854560256532093554, 0.4647231720437695057 ) ) ;
#9118=DIRECTION ( 'NONE',  ( 0.000000000000000000, 0.000000000000000000, 1.000000000000000000 ) ) ;
#9121=CARTESIAN_POINT ( 'NONE',  ( -336.3521761649654422, -182.5000000000000568, 1.632288850093980725 ) ) ;
#9129=CARTESIAN_POINT ( 'NONE',  ( 0.000000000000000000, -175.7419055135395922, -27.41866715058203852 ) ) ;
#9132=CARTESIAN_POINT ( 'NONE',  ( -332.3517673607765914, -125.1322888500942270, -59.97779283292990016 ) ) ;
#9135=CARTESIAN_POINT ( 'NONE',  ( -339.1964088526558498, -123.5000000000000284, 0.000000000000000000 ) ) ;
#9136=PLANE ( 'NONE',  #24560 ) ;
#9138=EDGE_CURVE ( 'NONE', #49593, #24719, #30892, .T. ) ;
#9142=ORIENTED_EDGE ( 'NONE', *, *, #9960, .F. ) ;
#9149=DIRECTION ( 'NONE',  ( 1.000000000000000000, 0.000000000000000000, -0.000000000000000000 ) ) ;
#9150=LINE ( 'NONE', #29882, #30521 ) ;
#9156=DIRECTION ( 'NONE',  ( 0.000000000000000000, 0.000000000000000000, -1.000000000000000000 ) ) ;
#9161=VERTEX_POINT ( 'NONE', #23004 ) ;
#9168=EDGE_LOOP ( 'NONE', ( #49934, #22485, #7141, #7027 ) ) ;
#9172=EDGE_LOOP ( 'NONE', ( #44787, #25247, #26016, #19974 ) ) ;
#9175=AXIS2_PLACEMENT_3D ( 'NONE', #2346, #42266, #34396 ) ;
#9176=FACE_OUTER_BOUND ( 'NONE', #49360, .T. ) ;
#9180=DIRECTION ( 'NONE',  ( 1.000000000000000000, -0.000000000000000000, -0.000000000000000000 ) ) ;
#9183=DIRECTION ( 'NONE',  ( 0.000000000000000000, -0.3546048870425235200, 0.9350162426854194964 ) ) ;
#9185=DIRECTION ( 'NONE',  ( 0.000000000000000000, 0.1205366802553199251, -0.9927088740980544168 ) ) ;
#9186=LINE ( 'NONE', #25209, #44119 ) ;
#9189=CARTESIAN_POINT ( 'NONE',  ( -332.3517673607765914, -114.6500883362968892, 59.34373651485599055 ) ) ;
#9191=EDGE_CURVE ( 'NONE', #9672, #34082, #8062, .T. ) ;
#9192=ADVANCED_FACE ( 'NONE', ( #11419 ), #39014, .F. ) ;
#9193=FACE_OUTER_BOUND ( 'NONE', #5403, .T. ) ;
#9197=VERTEX_POINT ( 'NONE', #50872 ) ;
#9198=VECTOR ( 'NONE', #39001, 1000.000000000000000 ) ;
#9204=CARTESIAN_POINT ( 'NONE',  ( -336.3521761649654422, -123.5000000000000284, 0.000000000000000000 ) ) ;
#9205=LINE ( 'NONE', #16576, #37776 ) ;
#9207=ORIENTED_EDGE ( 'NONE', *, *, #17246, .T. ) ;
#9209=AXIS2_PLACEMENT_3D ( 'NONE', #19341, #15403, #43512 ) ;
#9214=CARTESIAN_POINT ( 'NONE',  ( -339.1964088526558498, -103.0458197858333165, -55.34326076196084188 ) ) ;
#9216=CARTESIAN_POINT ( 'NONE',  ( 0.000000000000000000, -116.3883358649353141, 58.56982357178514320 ) ) ;
#9222=DIRECTION ( 'NONE',  ( -0.000000000000000000, 0.9350162426854181641, 0.3546048870425267951 ) ) ;
#9223=EDGE_LOOP ( 'NONE', ( #35980, #45338, #40807, #19531 ) ) ;
#9228=DIRECTION ( 'NONE',  ( -0.000000000000000000, 1.000000000000000000, -0.000000000000000000 ) ) ;
#9232=AXIS2_PLACEMENT_3D ( 'NONE', #30387, #30918, #46440 ) ;
#9237=LINE ( 'NONE', #49695, #27481 ) ;
#9246=EDGE_CURVE ( 'NONE', #6229, #27746, #12565, .T. ) ;
#9248=VERTEX_POINT ( 'NONE', #21238 ) ;
#9249=EDGE_CURVE ( 'NONE', #50694, #13737, #5218, .T. ) ;
#9250=AXIS2_PLACEMENT_3D ( 'NONE', #28105, #12608, #5006 ) ;
#9251=CARTESIAN_POINT ( 'NONE',  ( -305.0000000000000568, -65.12585595286518014, 13.87297036558326013 ) ) ;
#9255=DIRECTION ( 'NONE',  ( -0.000000000000000000, -0.8229838658936516893, 0.5680647467311626952 ) ) ;
#9258=PLANE ( 'NONE',  #12801 ) ;
#9260=ORIENTED_EDGE ( 'NONE', *, *, #10815, .F. ) ;
#9272=DIRECTION ( 'NONE',  ( 0.000000000000000000, 0.000000000000000000, 1.000000000000000000 ) ) ;
#9273=ORIENTED_EDGE ( 'NONE', *, *, #28374, .F. ) ;
#9274=EDGE_CURVE ( 'NONE', #7810, #44829, #8617, .T. ) ;
#9275=DIRECTION ( 'NONE',  ( -0.000000000000000000, -0.7485107481710953081, 0.6631226582408016323 ) ) ;
#9279=LINE ( 'NONE', #8482, #33152 ) ;
#9281=FACE_OUTER_BOUND ( 'NONE', #17422, .T. ) ;
#9286=ADVANCED_FACE ( 'NONE', ( #33323 ), #36998, .F. ) ;
#9288=CARTESIAN_POINT ( 'NONE',  ( -330.4913330509368166, -66.09477493971897388, 13.63415328425216622 ) ) ;
#9289=PLANE ( 'NONE',  #5602 ) ;
#9290=ADVANCED_FACE ( 'NONE', ( #14325 ), #30338, .F. ) ;
#9294=LINE ( 'NONE', #21644, #41806 ) ;
#9298=VERTEX_POINT ( 'NONE', #49366 ) ;
#9299=CARTESIAN_POINT ( 'NONE',  ( -332.3517673607765914, -162.0508476703726330, 45.97643030831915212 ) ) ;
#9301=DIRECTION ( 'NONE',  ( -0.000000000000000000, -0.6631226582407885317, 0.7485107481711069655 ) ) ;
#9302=AXIS2_PLACEMENT_3D ( 'NONE', #17691, #34470, #46069 ) ;
#9310=DIRECTION ( 'NONE',  ( -0.000000000000000000, -0.9350162426854132791, 0.3546048870425396182 ) ) ;
#9311=ORIENTED_EDGE ( 'NONE', *, *, #10110, .T. ) ;
#9313=DIRECTION ( 'NONE',  ( 0.000000000000000000, -0.9709418174260544543, -0.2393156642875482465 ) ) ;
#9319=DIRECTION ( 'NONE',  ( -1.000000000000000000, 0.000000000000000000, -0.000000000000000000 ) ) ;
#9323=LINE ( 'NONE', #13261, #1788 ) ;
#9324=CARTESIAN_POINT ( 'NONE',  ( -336.3521761649654422, -153.6873197461136158, -51.85292399224849902 ) ) ;
#9327=CARTESIAN_POINT ( 'NONE',  ( -336.3521761649654422, -113.7752393642576720, 58.25253621232167944 ) ) ;
#9330=ORIENTED_EDGE ( 'NONE', *, *, #40895, .T. ) ;
#9333=FACE_OUTER_BOUND ( 'NONE', #49656, .T. ) ;
#9335=FACE_OUTER_BOUND ( 'NONE', #24261, .T. ) ;
#9337=ORIENTED_EDGE ( 'NONE', *, *, #8632, .T. ) ;
#9338=ORIENTED_EDGE ( 'NONE', *, *, #31926, .T. ) ;
#9339=CIRCLE ( 'NONE', #16053, 60.00000000000000000 ) ;
#9340=ORIENTED_EDGE ( 'NONE', *, *, #21689, .T. ) ;
#9349=ORIENTED_EDGE ( 'NONE', *, *, #13516, .F. ) ;
#9351=ORIENTED_EDGE ( 'NONE', *, *, #21443, .T. ) ;
#9355=CARTESIAN_POINT ( 'NONE',  ( -336.3521761649654422, -147.2170408776451609, -55.11353710303946940 ) ) ;
#9356=DIRECTION ( 'NONE',  ( 0.000000000000000000, 0.000000000000000000, 1.000000000000000000 ) ) ;
#9358=DIRECTION ( 'NONE',  ( 0.000000000000000000, 5.319818659662208160E-15, -1.000000000000000000 ) ) ;
#9364=DIRECTION ( 'NONE',  ( 0.000000000000000000, 0.8229838658936575735, 0.5680647467311540355 ) ) ;
#9365=EDGE_CURVE ( 'NONE', #31967, #10943, #14587, .T. ) ;
#9369=VECTOR ( 'NONE', #35878, 1000.000000000000000 ) ;
#9370=CARTESIAN_POINT ( 'NONE',  ( -336.3521761649654422, -91.32752733096738496, -49.48329383994654052 ) ) ;
#9371=CARTESIAN_POINT ( 'NONE',  ( -332.3517673607765914, -100.1170788342122080, 54.23253582808833073 ) ) ;
#9384=ORIENTED_EDGE ( 'NONE', *, *, #10826, .T. ) ;
#9385=FACE_OUTER_BOUND ( 'NONE', #28511, .T. ) ;
#9389=AXIS2_PLACEMENT_3D ( 'NONE', #26969, #47741, #43003 ) ;
#9391=LINE ( 'NONE', #40916, #33793 ) ;
#9392=ORIENTED_EDGE ( 'NONE', *, *, #46155, .F. ) ;
#9395=ORIENTED_EDGE ( 'NONE', *, *, #1199, .T. ) ;
#9396=ORIENTED_EDGE ( 'NONE', *, *, #20337, .F. ) ;
#9398=CARTESIAN_POINT ( 'NONE',  ( -330.4913330509368166, -172.5932850007654338, 34.49419324804716069 ) ) ;
#9401=CARTESIAN_POINT ( 'NONE',  ( -330.4913330509368166, -123.5000000000000284, 0.000000000000000000 ) ) ;
#9402=CARTESIAN_POINT ( 'NONE',  ( -339.1964088526558498, -123.5000000000000284, 0.000000000000000000 ) ) ;
#9406=VECTOR ( 'NONE', #25085, 1000.000000000000114 ) ;
#9411=LINE ( 'NONE', #37520, #28140 ) ;
#9413=VERTEX_POINT ( 'NONE', #2743 ) ;
#9420=CARTESIAN_POINT ( 'NONE',  ( -339.1964088526558498, -64.99044476834248485, -7.608018572113150135 ) ) ;
#9421=ORIENTED_EDGE ( 'NONE', *, *, #22807, .F. ) ;
#9423=ORIENTED_EDGE ( 'NONE', *, *, #3447, .T. ) ;
#9424=DIRECTION ( 'NONE',  ( 0.000000000000000000, -0.4647231720437755564, -0.8854560256532062468 ) ) ;
#9431=ORIENTED_EDGE ( 'NONE', *, *, #31727, .T. ) ;
#9435=CARTESIAN_POINT ( 'NONE',  ( -336.3521761649654422, -86.34605966037949543, -45.90766452162698386 ) ) ;
#9436=DIRECTION ( 'NONE',  ( -0.000000000000000000, 0.000000000000000000, -1.000000000000000000 ) ) ;
#9443=DIRECTION ( 'NONE',  ( -0.000000000000000000, 0.9927088740980556381, 0.1205366802553095307 ) ) ;
#9446=EDGE_CURVE ( 'NONE', #13290, #25971, #3516, .T. ) ;
#9448=VECTOR ( 'NONE', #33369, 1000.000000000000000 ) ;
#9452=DIRECTION ( 'NONE',  ( 0.000000000000000000, -0.8229838658936634577, -0.5680647467311457088 ) ) ;
#9455=ORIENTED_EDGE ( 'NONE', *, *, #39755, .F. ) ;
#9457=DIRECTION ( 'NONE',  ( 0.000000000000000000, 0.000000000000000000, 1.000000000000000000 ) ) ;
#9459=ORIENTED_EDGE ( 'NONE', *, *, #8944, .F. ) ;
#9465=EDGE_LOOP ( 'NONE', ( #15946, #32271, #12859, #40664 ) ) ;
#9466=ADVANCED_FACE ( 'NONE', ( #43475 ), #7478, .F. ) ;
#9469=LINE ( 'NONE', #17628, #51912 ) ;
#9470=DIRECTION ( 'NONE',  ( -1.000000000000000000, 0.000000000000000000, -0.000000000000000000 ) ) ;
#9473=PLANE ( 'NONE',  #45136 ) ;
#9475=EDGE_CURVE ( 'NONE', #30972, #3140, #47932, .T. ) ;
#9476=CARTESIAN_POINT ( 'NONE',  ( -305.0000000000000568, -177.3662605214052519, -26.42775013958059560 ) ) ;
#9477=ORIENTED_EDGE ( 'NONE', *, *, #16352, .T. ) ;
#9483=DIRECTION ( 'NONE',  ( 0.000000000000000000, 0.000000000000000000, -1.000000000000000000 ) ) ;
#9487=LINE ( 'NONE', #41017, #42487 ) ;
#9489=CARTESIAN_POINT ( 'NONE',  ( -330.4913330509368166, -89.57268800991444380, 48.27201571435978877 ) ) ;
#9493=DIRECTION ( 'NONE',  ( -0.000000000000000000, 0.2393156642875547968, -0.9709418174260527890 ) ) ;
#9500=CARTESIAN_POINT ( 'NONE',  ( -336.3521761649653854, -173.7880015656344312, -32.72792230702632565 ) ) ;
#9501=ORIENTED_EDGE ( 'NONE', *, *, #34453, .F. ) ;
#9503=CARTESIAN_POINT ( 'NONE',  ( -339.1964088526558498, -162.9984922102920848, 43.83057281297495678 ) ) ;
#9505=CARTESIAN_POINT ( 'NONE',  ( -332.3517673607765914, -133.2247606357419443, -58.25253621232173629 ) ) ;
#9509=LINE ( 'NONE', #578, #6857 ) ;
#9510=FACE_OUTER_BOUND ( 'NONE', #19591, .T. ) ;
#9511=FACE_OUTER_BOUND ( 'NONE', #20436, .T. ) ;
#9512=ORIENTED_EDGE ( 'NONE', *, *, #35668, .F. ) ;
#9515=EDGE_CURVE ( 'NONE', #12661, #34438, #28198, .T. ) ;
#9523=CARTESIAN_POINT ( 'NONE',  ( -339.1964088526558498, -89.57268800991437274, 48.27201571435973904 ) ) ;
#9532=EDGE_LOOP ( 'NONE', ( #4409, #30399, #13443, #40431 ) ) ;
#9533=AXIS2_PLACEMENT_3D ( 'NONE', #45113, #13024, #41146 ) ;
#9536=ORIENTED_EDGE ( 'NONE', *, *, #44292, .T. ) ;
#9537=LINE ( 'NONE', #21360, #28886 ) ;
#9538=EDGE_CURVE ( 'NONE', #32555, #24446, #16394, .T. ) ;
#9547=ORIENTED_EDGE ( 'NONE', *, *, #3578, .F. ) ;
#9549=VECTOR ( 'NONE', #41756, 1000.000000000000114 ) ;
#9550=EDGE_LOOP ( 'NONE', ( #20044, #2252, #15959, #42394 ) ) ;
#9552=CARTESIAN_POINT ( 'NONE',  ( -336.3521761649654422, -70.49953203435293858, 25.97334715265942151 ) ) ;
#9554=ORIENTED_EDGE ( 'NONE', *, *, #4181, .F. ) ;
#9555=CARTESIAN_POINT ( 'NONE',  ( -305.0000000000000568, -66.51961791625839737, 18.79457521708899392 ) ) ;
#9558=CARTESIAN_POINT ( 'NONE',  ( -305.0000000000000568, -182.1255794688777314, -12.76876783163924323 ) ) ;
#9560=LINE ( 'NONE', #28476, #7231 ) ;
#9562=FACE_OUTER_BOUND ( 'NONE', #9805, .T. ) ;
#9565=EDGE_LOOP ( 'NONE', ( #32056, #12443, #5007, #18584 ) ) ;
#9575=EDGE_CURVE ( 'NONE', #39066, #13383, #8750, .T. ) ;
#9576=DIRECTION ( 'NONE',  ( 0.000000000000000000, -2.326842422443557418E-13, 1.000000000000000000 ) ) ;
#9588=EDGE_CURVE ( 'NONE', #30266, #26571, #9791, .T. ) ;
#9602=ADVANCED_FACE ( 'NONE', ( #25311 ), #14008, .F. ) ;
#9610=DIRECTION ( 'NONE',  ( -0.000000000000000000, 0.9350162426854107256, -0.3546048870425463906 ) ) ;
#9612=CARTESIAN_POINT ( 'NONE',  ( -336.3521761649654422, -164.5945333327934463, -42.41660376256285048 ) ) ;
#9615=ORIENTED_EDGE ( 'NONE', *, *, #27234, .F. ) ;
#9620=ORIENTED_EDGE ( 'NONE', *, *, #33967, .T. ) ;
#9625=DIRECTION ( 'NONE',  ( 0.000000000000000000, -0.8229838658936613482, -0.5680647467311485954 ) ) ;
#9626=CARTESIAN_POINT ( 'NONE',  ( -332.3517673607765914, -133.2247606357419443, -58.25253621232173629 ) ) ;
#9627=AXIS2_PLACEMENT_3D ( 'NONE', #30829, #18744, #46876 ) ;
#9628=DIRECTION ( 'NONE',  ( 0.000000000000000000, 1.156482317317871449E-14, -1.000000000000000000 ) ) ;
#9631=CARTESIAN_POINT ( 'NONE',  ( -339.1964088526558498, -173.1613497474965300, 33.67120938215357739 ) ) ;
#9635=ADVANCED_FACE ( 'NONE', ( #9802 ), #45551, .F. ) ;
#9636=CARTESIAN_POINT ( 'NONE',  ( -180.0000000000000568, -123.5000000000000284, 0.000000000000000000 ) ) ;
#9638=ORIENTED_EDGE ( 'NONE', *, *, #15285, .F. ) ;
#9643=CARTESIAN_POINT ( 'NONE',  ( -332.3517673607765914, -132.2320517616439020, -58.37307289257706344 ) ) ;
#9651=VECTOR ( 'NONE', #3596, 1000.000000000000114 ) ;
#9652=ADVANCED_FACE ( 'NONE', ( #33468 ), #9289, .F. ) ;
#9653=ORIENTED_EDGE ( 'NONE', *, *, #11124, .T. ) ;
#9654=PLANE ( 'NONE',  #10856 ) ;
#9656=DIRECTION ( 'NONE',  ( -1.000000000000000000, 0.000000000000000000, -0.000000000000000000 ) ) ;
#9661=FACE_OUTER_BOUND ( 'NONE', #3291, .T. ) ;
#9663=EDGE_LOOP ( 'NONE', ( #23122, #47390, #6057, #14155 ) ) ;
#9667=VECTOR ( 'NONE', #39117, 1000.000000000000000 ) ;
#9670=CARTESIAN_POINT ( 'NONE',  ( -332.3517673607765914, -182.2665742509934148, -5.491276508484069119 ) ) ;
#9672=VERTEX_POINT ( 'NONE', #29500 ) ;
#9673=LINE ( 'NONE', #10437, #17825 ) ;
#9674=CARTESIAN_POINT ( 'NONE',  ( -332.3517673607765914, -123.5000000000000284, 0.000000000000000000 ) ) ;
#9677=VECTOR ( 'NONE', #51546, 1000.000000000000114 ) ;
#9679=AXIS2_PLACEMENT_3D ( 'NONE', #10487, #30215, #33636 ) ;
#9680=EDGE_LOOP ( 'NONE', ( #37141, #25871, #24226, #46427 ) ) ;
#9683=DIRECTION ( 'NONE',  ( 1.000000000000000000, -0.000000000000000000, -0.000000000000000000 ) ) ;
#9699=CIRCLE ( 'NONE', #12191, 60.00000000000000000 ) ;
#9701=CARTESIAN_POINT ( 'NONE',  ( -330.4913330509368166, -150.4759391377560576, -52.47426709956116042 ) ) ;
#9702=ORIENTED_EDGE ( 'NONE', *, *, #47746, .T. ) ;
#9703=ADVANCED_FACE ( 'NONE', ( #38158 ), #2167, .F. ) ;
#9710=AXIS2_PLACEMENT_3D ( 'NONE', #45467, #13140, #9457 ) ;
#9716=ORIENTED_EDGE ( 'NONE', *, *, #32358, .F. ) ;
#9720=EDGE_CURVE ( 'NONE', #5531, #1746, #9030, .T. ) ;
#9726=ORIENTED_EDGE ( 'NONE', *, *, #41365, .T. ) ;
#9728=DIRECTION ( 'NONE',  ( 0.000000000000000000, -0.8229838658936516893, 0.5680647467311626952 ) ) ;
#9735=ORIENTED_EDGE ( 'NONE', *, *, #23840, .T. ) ;
#9737=EDGE_CURVE ( 'NONE', #20555, #40265, #34235, .T. ) ;
#9739=DIRECTION ( 'NONE',  ( 0.000000000000000000, 0.000000000000000000, 1.000000000000000000 ) ) ;
#9745=DIRECTION ( 'NONE',  ( 0.000000000000000000, -6.129356281784718821E-14, -1.000000000000000000 ) ) ;
#9748=CARTESIAN_POINT ( 'NONE',  ( -330.4913330509368166, -123.5000000000000284, 0.000000000000000000 ) ) ;
#9749=LINE ( 'NONE', #25262, #39987 ) ;
#9753=ORIENTED_EDGE ( 'NONE', *, *, #22486, .T. ) ;
#9758=EDGE_CURVE ( 'NONE', #29300, #45837, #15294, .T. ) ;
#9761=ORIENTED_EDGE ( 'NONE', *, *, #37951, .F. ) ;
#9763=CARTESIAN_POINT ( 'NONE',  ( -339.1964088526558498, -167.3305728129748786, -39.49849221029221269 ) ) ;
#9766=DIRECTION ( 'NONE',  ( 0.000000000000000000, -0.8229838658936634577, -0.5680647467311457088 ) ) ;
#9772=DIRECTION ( 'NONE',  ( 0.000000000000000000, 0.4647231720437695057, 0.8854560256532093554 ) ) ;
#9777=DIRECTION ( 'NONE',  ( 1.000000000000000000, -0.000000000000000000, -0.000000000000000000 ) ) ;
#9781=AXIS2_PLACEMENT_3D ( 'NONE', #24469, #11856, #32347 ) ;
#9783=ADVANCED_FACE ( 'NONE', ( #11329 ), #26851, .F. ) ;
#9791=CIRCLE ( 'NONE', #30752, 60.00000000000000000 ) ;
#9793=DIRECTION ( 'NONE',  ( 0.000000000000000000, 0.8854560256532079121, -0.4647231720437724478 ) ) ;
#9795=VECTOR ( 'NONE', #17374, 1000.000000000000000 ) ;
#9797=EDGE_LOOP ( 'NONE', ( #22442, #32121, #40796, #32082 ) ) ;
#9798=LINE ( 'NONE', #49744, #24693 ) ;
#9799=ORIENTED_EDGE ( 'NONE', *, *, #29800, .F. ) ;
#9802=FACE_OUTER_BOUND ( 'NONE', #5743, .T. ) ;
#9805=EDGE_LOOP ( 'NONE', ( #25771, #37969, #11173, #14883 ) ) ;
#9806=DIRECTION ( 'NONE',  ( 0.000000000000000000, 0.8854560256532079121, -0.4647231720437724478 ) ) ;
#9807=VECTOR ( 'NONE', #8514, 1000.000000000000000 ) ;
#9812=ADVANCED_FACE ( 'NONE', ( #26339 ), #38677, .F. ) ;
#9815=CARTESIAN_POINT ( 'NONE',  ( -339.1964088526558498, -124.0000000000002700, -59.99791663049643375 ) ) ;
#9817=LINE ( 'NONE', #25846, #8131 ) ;
#9820=DIRECTION ( 'NONE',  ( -1.000000000000000000, 0.000000000000000000, 0.000000000000000000 ) ) ;
#9821=VECTOR ( 'NONE', #47051, 1000.000000000000000 ) ;
#9827=CARTESIAN_POINT ( 'NONE',  ( -330.4913330509368166, -151.3613951634084742, 52.00954392751779665 ) ) ;
#9828=CARTESIAN_POINT ( 'NONE',  ( -339.1964088526558498, -130.1153096980144426, 58.63009191191295599 ) ) ;
#9834=DIRECTION ( 'NONE',  ( 0.000000000000000000, 0.9709418174260511236, -0.2393156642875615969 ) ) ;
#9838=CARTESIAN_POINT ( 'NONE',  ( -336.3521761649654422, -99.78295912235451226, 55.11353710303931308 ) ) ;
#9842=FACE_OUTER_BOUND ( 'NONE', #33965, .T. ) ;
#9844=AXIS2_PLACEMENT_3D ( 'NONE', #16879, #16628, #44206 ) ;
#9848=FACE_OUTER_BOUND ( 'NONE', #48014, .T. ) ;
#9850=AXIS2_PLACEMENT_3D ( 'NONE', #12607, #49418, #37040 ) ;
#9852=LINE ( 'NONE', #46375, #41703 ) ;
#9859=VECTOR ( 'NONE', #9793, 999.9999999999998863 ) ;
#9861=DIRECTION ( 'NONE',  ( -1.000000000000000000, 0.000000000000000000, 0.000000000000000000 ) ) ;
#9862=DIRECTION ( 'NONE',  ( -0.000000000000000000, 0.5680647467311625842, 0.8229838658936516893 ) ) ;
#9864=AXIS2_PLACEMENT_3D ( 'NONE', #38629, #26541, #15243 ) ;
#9865=VECTOR ( 'NONE', #36273, 1000.000000000000114 ) ;
#9867=LINE ( 'NONE', #14077, #18970 ) ;
#9879=ORIENTED_EDGE ( 'NONE', *, *, #40781, .T. ) ;
#9887=ORIENTED_EDGE ( 'NONE', *, *, #33600, .F. ) ;
#9891=LINE ( 'NONE', #13036, #39758 ) ;
#9899=EDGE_LOOP ( 'NONE', ( #47402, #14302, #17003, #24794 ) ) ;
#9901=EDGE_CURVE ( 'NONE', #16323, #27843, #32336, .T. ) ;
#9902=CARTESIAN_POINT ( 'NONE',  ( -339.1964088526558498, -123.5000000000000284, 0.000000000000000000 ) ) ;
#9903=AXIS2_PLACEMENT_3D ( 'NONE', #3527, #18786, #43484 ) ;
#9907=ORIENTED_EDGE ( 'NONE', *, *, #13578, .F. ) ;
#9908=VECTOR ( 'NONE', #20188, 1000.000000000000000 ) ;
#9913=DIRECTION ( 'NONE',  ( 0.000000000000000000, 0.000000000000000000, -1.000000000000000000 ) ) ;
#9915=EDGE_CURVE ( 'NONE', #31493, #10996, #31837, .T. ) ;
#9916=VERTEX_POINT ( 'NONE', #27875 ) ;
#9921=LINE ( 'NONE', #5728, #8396 ) ;
#9922=AXIS2_PLACEMENT_3D ( 'NONE', #49627, #30410, #50158 ) ;
#9929=ORIENTED_EDGE ( 'NONE', *, *, #12161, .T. ) ;
#9940=CARTESIAN_POINT ( 'NONE',  ( -336.3521761649654422, -127.9985676343858501, 58.88711093124869222 ) ) ;
#9942=EDGE_CURVE ( 'NONE', #34815, #23236, #19735, .T. ) ;
#9947=ADVANCED_FACE ( 'NONE', ( #11848 ), #47623, .F. ) ;
#9948=AXIS2_PLACEMENT_3D ( 'NONE', #32018, #7594, #27300 ) ;
#9953=CARTESIAN_POINT ( 'NONE',  ( -332.3517673607765914, -174.5186198893880771, 29.74944317415823392 ) ) ;
#9957=LINE ( 'NONE', #46469, #28954 ) ;
#9960=EDGE_CURVE ( 'NONE', #1071, #32381, #32480, .T. ) ;
#9963=DIRECTION ( 'NONE',  ( 0.000000000000000000, -0.2393156642875652051, -0.9709418174260502354 ) ) ;
#9964=EDGE_CURVE ( 'NONE', #8561, #18461, #36542, .T. ) ;
#9966=VECTOR ( 'NONE', #50365, 1000.000000000000000 ) ;
#9969=EDGE_CURVE ( 'NONE', #40473, #27857, #3982, .T. ) ;
#9974=EDGE_CURVE ( 'NONE', #31069, #38530, #3942, .T. ) ;
#9979=EDGE_CURVE ( 'NONE', #13526, #4036, #16557, .T. ) ;
#9984=FACE_OUTER_BOUND ( 'NONE', #3746, .T. ) ;
#9993=LINE ( 'NONE', #30457, #51953 ) ;
#9994=FACE_OUTER_BOUND ( 'NONE', #33830, .T. ) ;
#9998=CARTESIAN_POINT ( 'NONE',  ( -330.4913330509368166, -103.0458197858324496, 55.34326076196052213 ) ) ;
#10000=CIRCLE ( 'NONE', #51988, 31.65769145387501027 ) ;
#10003=DIRECTION ( 'NONE',  ( 0.000000000000000000, 0.000000000000000000, 1.000000000000000000 ) ) ;
#10005=ORIENTED_EDGE ( 'NONE', *, *, #12492, .T. ) ;
#10010=DIRECTION ( 'NONE',  ( 0.000000000000000000, 0.8854560256532093554, -0.4647231720437695057 ) ) ;
#10019=CARTESIAN_POINT ( 'NONE',  ( -332.3517673607765914, -69.26746417191145611, -23.38292116578723068 ) ) ;
#10027=LINE ( 'NONE', #14483, #2968 ) ;
#10031=FACE_OUTER_BOUND ( 'NONE', #23039, .T. ) ;
#10032=EDGE_CURVE ( 'NONE', #19616, #47019, #17117, .T. ) ;
#10035=EDGE_CURVE ( 'NONE', #47727, #37884, #18238, .T. ) ;
#10037=VECTOR ( 'NONE', #48756, 1000.000000000000000 ) ;
#10042=ORIENTED_EDGE ( 'NONE', *, *, #1879, .T. ) ;
#10046=ORIENTED_EDGE ( 'NONE', *, *, #9901, .T. ) ;
#10052=ORIENTED_EDGE ( 'NONE', *, *, #34379, .F. ) ;
#10053=VECTOR ( 'NONE', #50387, 1000.000000000000000 ) ;
#10054=PLANE ( 'NONE',  #35186 ) ;
#10056=LINE ( 'NONE', #14518, #3962 ) ;
#10058=CARTESIAN_POINT ( 'NONE',  ( -339.1964088526558498, -124.0000000000002700, -59.00000000000002132 ) ) ;
#10062=EDGE_CURVE ( 'NONE', #27996, #21361, #13679, .T. ) ;
#10064=CARTESIAN_POINT ( 'NONE',  ( -180.0000000000000568, -123.5000000000000284, 20.00000000000001776 ) ) ;
#10065=CARTESIAN_POINT ( 'NONE',  ( -330.4913330509368166, -180.6659093959932250, 14.60509510167933556 ) ) ;
#10068=DIRECTION ( 'NONE',  ( 1.043714542225393381E-14, -0.9350162426854158326, -0.3546048870425331789 ) ) ;
#10083=EDGE_LOOP ( 'NONE', ( #14002, #34590, #40536, #12439 ) ) ;
#10087=AXIS2_PLACEMENT_3D ( 'NONE', #21691, #13283, #1450 ) ;
#10090=CARTESIAN_POINT ( 'NONE',  ( -330.4913330509368166, -103.0458197858332312, -55.34326076196081345 ) ) ;
#10091=EDGE_LOOP ( 'NONE', ( #26263, #50478, #51324, #27982 ) ) ;
#10093=DIRECTION ( 'NONE',  ( -1.000000000000000000, -0.000000000000000000, -1.043714542225393381E-14 ) ) ;
#10097=CARTESIAN_POINT ( 'NONE',  ( 0.000000000000000000, -64.93017642821482127, -7.111664135064078351 ) ) ;
#10102=DIRECTION ( 'NONE',  ( -1.000000000000000000, 0.000000000000000000, 0.000000000000000000 ) ) ;
#10105=LINE ( 'NONE', #5398, #32788 ) ;
#10109=ORIENTED_EDGE ( 'NONE', *, *, #24077, .T. ) ;
#10110=EDGE_CURVE ( 'NONE', #14029, #32415, #42046, .T. ) ;
#10115=VERTEX_POINT ( 'NONE', #36821 ) ;
#10116=EDGE_CURVE ( 'NONE', #19768, #35535, #33898, .T. ) ;
#10120=VECTOR ( 'NONE', #12125, 1000.000000000000000 ) ;
#10122=CARTESIAN_POINT ( 'NONE',  ( -339.1964088526558498, -183.1207326066167695, -6.735595255826207328 ) ) ;
#10124=CARTESIAN_POINT ( 'NONE',  ( -330.4913330509368166, -123.5000000000000284, 0.000000000000000000 ) ) ;
#10128=DIRECTION ( 'NONE',  ( 1.000000000000000000, 0.000000000000000000, 0.000000000000000000 ) ) ;
#10129=CARTESIAN_POINT ( 'NONE',  ( -305.0000000000000568, -129.1091364105427033, 59.73723787327234191 ) ) ;
#10136=EDGE_CURVE ( 'NONE', #15154, #26719, #44975, .T. ) ;
#10140=DIRECTION ( 'NONE',  ( -1.000000000000000000, -0.000000000000000000, 0.000000000000000000 ) ) ;
#10141=PLANE ( 'NONE',  #29903 ) ;
#10146=VECTOR ( 'NONE', #29718, 1000.000000000000000 ) ;
#10152=PLANE ( 'NONE',  #32650 ) ;
#10153=FACE_OUTER_BOUND ( 'NONE', #45646, .T. ) ;
#10158=EDGE_CURVE ( 'NONE', #13339, #45638, #29186, .T. ) ;
#10161=ORIENTED_EDGE ( 'NONE', *, *, #27431, .T. ) ;
#10167=DIRECTION ( 'NONE',  ( -1.000000000000000000, 0.000000000000000000, -0.000000000000000000 ) ) ;
#10168=CARTESIAN_POINT ( 'NONE',  ( -305.0000000000000568, -162.9117225908387070, 45.24064679492076380 ) ) ;
#10181=CARTESIAN_POINT ( 'NONE',  ( -339.1964088526558498, -68.15673923803930734, -20.45418021416698551 ) ) ;
#10183=EDGE_LOOP ( 'NONE', ( #5224, #40217, #37398, #23598 ) ) ;
#10189=EDGE_LOOP ( 'NONE', ( #37011, #31868, #1008, #4724 ) ) ;
#10202=DIRECTION ( 'NONE',  ( 0.000000000000000000, 0.3546048870425267951, -0.9350162426854181641 ) ) ;
#10204=AXIS2_PLACEMENT_3D ( 'NONE', #24556, #28238, #9065 ) ;
#10211=CARTESIAN_POINT ( 'NONE',  ( -330.4913330509368166, -95.63860483659048839, 52.00954392751722111 ) ) ;
#10214=CARTESIAN_POINT ( 'NONE',  ( -305.0000000000000568, -183.1207326066166559, 6.735595255827129257 ) ) ;
#10216=CARTESIAN_POINT ( 'NONE',  ( -339.1964088526558498, -75.22798428563942252, 33.92731199008440512 ) ) ;
#10218=EDGE_CURVE ( 'NONE', #28909, #5759, #3141, .T. ) ;
#10219=EDGE_CURVE ( 'NONE', #49982, #48449, #15232, .T. ) ;
#10222=CIRCLE ( 'NONE', #41238, 60.00000000000000000 ) ;
#10225=EDGE_CURVE ( 'NONE', #8474, #42568, #34169, .T. ) ;
#10228=ORIENTED_EDGE ( 'NONE', *, *, #6275, .T. ) ;
#10230=VERTEX_POINT ( 'NONE', #47037 ) ;
#10231=ADVANCED_FACE ( 'NONE', ( #38364 ), #14464, .T. ) ;
#10233=ADVANCED_FACE ( 'NONE', ( #10251 ), #23118, .F. ) ;
#10234=VECTOR ( 'NONE', #41620, 1000.000000000000000 ) ;
#10236=CARTESIAN_POINT ( 'NONE',  ( -339.1964088526558498, -68.51134412508183402, -21.38919645685240312 ) ) ;
#10237=LINE ( 'NONE', #34662, #13885 ) ;
#10238=ORIENTED_EDGE ( 'NONE', *, *, #20828, .F. ) ;
#10239=DIRECTION ( 'NONE',  ( -1.000000000000000000, 0.000000000000000000, 0.000000000000000000 ) ) ;
#10247=CARTESIAN_POINT ( 'NONE',  ( -336.3521761649654422, -154.8494888031386836, 50.05135858667791382 ) ) ;
#10251=FACE_OUTER_BOUND ( 'NONE', #49541, .T. ) ;
#10258=EDGE_LOOP ( 'NONE', ( #29017, #14513, #35786, #7480 ) ) ;
#10259=CARTESIAN_POINT ( 'NONE',  ( -332.3517673607765914, -63.55776901541228341, -2.632288850093980503 ) ) ;
#10261=ORIENTED_EDGE ( 'NONE', *, *, #35779, .T. ) ;
#10263=PLANE ( 'NONE',  #15767 ) ;
#10264=DIRECTION ( 'NONE',  ( 0.000000000000000000, 7.632783294297951215E-14, -1.000000000000000000 ) ) ;
#10265=CARTESIAN_POINT ( 'NONE',  ( -339.1964088526558498, -64.99044476834248485, -7.608018572113150135 ) ) ;
#10274=ORIENTED_EDGE ( 'NONE', *, *, #11877, .T. ) ;
#10280=VECTOR ( 'NONE', #43209, 1000.000000000000000 ) ;
#10282=VECTOR ( 'NONE', #7805, 999.9999999999998863 ) ;
#10284=PLANE ( 'NONE',  #6037 ) ;
#10292=ADVANCED_FACE ( 'NONE', ( #28340 ), #27569, .F. ) ;
#10293=LINE ( 'NONE', #34711, #2836 ) ;
#10294=DIRECTION ( 'NONE',  ( -1.000000000000000000, 0.000000000000000000, 0.000000000000000000 ) ) ;
#10295=ORIENTED_EDGE ( 'NONE', *, *, #49794, .F. ) ;
#10303=VECTOR ( 'NONE', #46302, 999.9999999999998863 ) ;
#10309=ADVANCED_FACE ( 'NONE', ( #43601 ), #3649, .F. ) ;
#10311=EDGE_LOOP ( 'NONE', ( #2525, #46067, #51159, #5322 ) ) ;
#10314=DIRECTION ( 'NONE',  ( 0.000000000000000000, 1.000000000000000000, -1.047444401652940007E-14 ) ) ;
#10318=EDGE_CURVE ( 'NONE', #26071, #43135, #12328, .T. ) ;
#10327=VERTEX_POINT ( 'NONE', #44392 ) ;
#10328=FACE_BOUND ( 'NONE', #44890, .T. ) ;
#10329=PLANE ( 'NONE',  #13053 ) ;
#10332=ORIENTED_EDGE ( 'NONE', *, *, #24055, .T. ) ;
#10334=LINE ( 'NONE', #14547, #5213 ) ;
#10336=AXIS2_PLACEMENT_3D ( 'NONE', #19323, #23769, #35584 ) ;
#10339=PLANE ( 'NONE',  #30768 ) ;
#10345=FACE_OUTER_BOUND ( 'NONE', #27545, .T. ) ;
#10346=CARTESIAN_POINT ( 'NONE',  ( -332.3517673607765914, -92.15051119686104641, -50.05135858667769355 ) ) ;
#10347=ORIENTED_EDGE ( 'NONE', *, *, #26937, .T. ) ;
#10348=EDGE_LOOP ( 'NONE', ( #9536, #13626, #37701, #9879 ) ) ;
#10354=ORIENTED_EDGE ( 'NONE', *, *, #39749, .F. ) ;
#10363=ORIENTED_EDGE ( 'NONE', *, *, #12192, .F. ) ;
#10367=EDGE_CURVE ( 'NONE', #2629, #45033, #4439, .T. ) ;
#10370=AXIS2_PLACEMENT_3D ( 'NONE', #51386, #39527, #31654 ) ;
#10371=ORIENTED_EDGE ( 'NONE', *, *, #44869, .T. ) ;
#10375=ORIENTED_EDGE ( 'NONE', *, *, #32035, .F. ) ;
#10380=PLANE ( 'NONE',  #4132 ) ;
#10382=LINE ( 'NONE', #26406, #18368 ) ;
#10384=VECTOR ( 'NONE', #14007, 1000.000000000000000 ) ;
#10388=LINE ( 'NONE', #7228, #45463 ) ;
#10389=EDGE_LOOP ( 'NONE', ( #37796, #17128, #25499, #49878 ) ) ;
#10391=DIRECTION ( 'NONE',  ( 0.000000000000000000, -2.201942332173227054E-13, -1.000000000000000000 ) ) ;
#10394=EDGE_CURVE ( 'NONE', #26301, #15638, #8380, .T. ) ;
#10398=ORIENTED_EDGE ( 'NONE', *, *, #22742, .T. ) ;
#10401=ORIENTED_EDGE ( 'NONE', *, *, #16996, .T. ) ;
#10406=DIRECTION ( 'NONE',  ( 0.000000000000000000, -5.782411586589357402E-14, 1.000000000000000000 ) ) ;
#10410=DIRECTION ( 'NONE',  ( -0.000000000000000000, 0.7485107481710999711, -0.6631226582407964143 ) ) ;
#10428=LINE ( 'NONE', #2556, #2981 ) ;
#10429=ORIENTED_EDGE ( 'NONE', *, *, #1582, .F. ) ;
#10430=ORIENTED_EDGE ( 'NONE', *, *, #33174, .T. ) ;
#10432=ORIENTED_EDGE ( 'NONE', *, *, #34549, .F. ) ;
#10433=PLANE ( 'NONE',  #45968 ) ;
#10434=AXIS2_PLACEMENT_3D ( 'NONE', #4645, #36709, #9118 ) ;
#10437=CARTESIAN_POINT ( 'NONE',  ( -339.1964088526558498, -171.7720157143598669, 33.92731199008546383 ) ) ;
#10438=DIRECTION ( 'NONE',  ( 0.000000000000000000, 1.249000902703301108E-14, -1.000000000000000000 ) ) ;
#10439=VERTEX_POINT ( 'NONE', #8633 ) ;
#10441=ORIENTED_EDGE ( 'NONE', *, *, #14304, .F. ) ;
#10442=VECTOR ( 'NONE', #45831, 1000.000000000000000 ) ;
#10444=CARTESIAN_POINT ( 'NONE',  ( -336.3521761649654422, -169.4076645216271402, -37.15394033962039089 ) ) ;
#10448=DIRECTION ( 'NONE',  ( 1.000000000000000000, 0.000000000000000000, -0.000000000000000000 ) ) ;
#10449=LINE ( 'NONE', #2330, #33998 ) ;
#10450=EDGE_CURVE ( 'NONE', #31317, #34375, #47652, .T. ) ;
#10455=VERTEX_POINT ( 'NONE', #44640 ) ;
#10458=DIRECTION ( 'NONE',  ( 0.000000000000000000, 0.8854560256532157947, 0.4647231720437573488 ) ) ;
#10463=DIRECTION ( 'NONE',  ( -1.000000000000000000, 0.000000000000000000, -0.000000000000000000 ) ) ;
#10464=EDGE_CURVE ( 'NONE', #76, #7181, #15282, .T. ) ;
#10468=VECTOR ( 'NONE', #44649, 1000.000000000000000 ) ;
#10475=FACE_OUTER_BOUND ( 'NONE', #26639, .T. ) ;
#10476=ORIENTED_EDGE ( 'NONE', *, *, #32585, .T. ) ;
#10477=CIRCLE ( 'NONE', #22226, 60.00000000000000000 ) ;
#10478=FACE_OUTER_BOUND ( 'NONE', #29262, .T. ) ;
#10479=ORIENTED_EDGE ( 'NONE', *, *, #36626, .F. ) ;
#10480=CARTESIAN_POINT ( 'NONE',  ( -332.3517673607765914, -169.4764303083190384, -38.55084767037274673 ) ) ;
#10487=CARTESIAN_POINT ( 'NONE',  ( -330.4913330509368166, -115.8919814278863356, 58.50955523165747252 ) ) ;
#10488=ORIENTED_EDGE ( 'NONE', *, *, #42366, .F. ) ;
#10492=DIRECTION ( 'NONE',  ( -8.718379230999708359E-17, -0.2393156642875449158, 0.9709418174260553425 ) ) ;
#10493=EDGE_LOOP ( 'NONE', ( #23481, #104, #46016, #41854 ) ) ;
#10494=CARTESIAN_POINT ( 'NONE',  ( -330.4913330509368166, -182.5000000000000568, -0.4999999999999551470 ) ) ;
#10504=VECTOR ( 'NONE', #31581, 1000.000000000000000 ) ;
#10506=EDGE_LOOP ( 'NONE', ( #36362, #41438, #6048, #7514 ) ) ;
#10507=LINE ( 'NONE', #22616, #33100 ) ;
#10508=LINE ( 'NONE', #6595, #10724 ) ;
#10516=ORIENTED_EDGE ( 'NONE', *, *, #16352, .F. ) ;
#10518=CARTESIAN_POINT ( 'NONE',  ( -336.3521761649654422, -166.5797264208035244, 40.34602258462248159 ) ) ;
#10521=EDGE_CURVE ( 'NONE', #11143, #41973, #46836, .T. ) ;
#10522=DIRECTION ( 'NONE',  ( 1.000000000000000000, -0.000000000000000000, -0.000000000000000000 ) ) ;
#10535=EDGE_CURVE ( 'NONE', #14596, #45545, #34471, .T. ) ;
#10549=CARTESIAN_POINT ( 'NONE',  ( -305.0000000000000568, -63.87926739338328730, 6.735595255826143379 ) ) ;
#10554=EDGE_LOOP ( 'NONE', ( #18312, #34987, #41382, #27060 ) ) ;
#10556=DIRECTION ( 'NONE',  ( 0.000000000000000000, 0.000000000000000000, -1.000000000000000000 ) ) ;
#10569=PLANE ( 'NONE',  #38065 ) ;
#10570=CARTESIAN_POINT ( 'NONE',  ( -330.4913330509368166, -84.00150778970706256, 43.83057281297416097 ) ) ;
#10573=LINE ( 'NONE', #2685, #28122 ) ;
#10578=EDGE_CURVE ( 'NONE', #50151, #10964, #42098, .T. ) ;
#10579=EDGE_CURVE ( 'NONE', #34048, #6061, #47088, .T. ) ;
#10580=ORIENTED_EDGE ( 'NONE', *, *, #7338, .T. ) ;
#10583=LINE ( 'NONE', #42647, #29827 ) ;
#10586=LINE ( 'NONE', #9555, #28268 ) ;
#10592=EDGE_LOOP ( 'NONE', ( #2300, #20158, #25562, #50717 ) ) ;
#10602=DIRECTION ( 'NONE',  ( -0.000000000000000000, 0.9927088740980556381, 0.1205366802553095307 ) ) ;
#10604=CARTESIAN_POINT ( 'NONE',  ( -330.4913330509368166, -123.0000000000002700, -59.99791663049643375 ) ) ;
#10607=AXIS2_PLACEMENT_3D ( 'NONE', #26214, #21777, #46219 ) ;
#10609=ORIENTED_EDGE ( 'NONE', *, *, #11709, .F. ) ;
#10623=ORIENTED_EDGE ( 'NONE', *, *, #40134, .T. ) ;
#10627=CARTESIAN_POINT ( 'NONE',  ( -305.0000000000000568, -69.20050475944881896, 25.52576769896171882 ) ) ;
#10628=VECTOR ( 'NONE', #46809, 1000.000000000000000 ) ;
#10629=VECTOR ( 'NONE', #39719, 1000.000000000000000 ) ;
#10632=ORIENTED_EDGE ( 'NONE', *, *, #23110, .T. ) ;
#10638=VECTOR ( 'NONE', #47984, 1000.000000000000114 ) ;
#10639=PLANE ( 'NONE',  #25648 ) ;
#10640=CARTESIAN_POINT ( 'NONE',  ( -336.3521761649654422, -123.5000000000000284, 0.000000000000000000 ) ) ;
#10643=VECTOR ( 'NONE', #34233, 999.9999999999998863 ) ;
#10646=EDGE_CURVE ( 'NONE', #49014, #18461, #32075, .T. ) ;
#10651=VECTOR ( 'NONE', #13792, 1000.000000000000000 ) ;
#10652=AXIS2_PLACEMENT_3D ( 'NONE', #40480, #28130, #27634 ) ;
#10656=ORIENTED_EDGE ( 'NONE', *, *, #32716, .F. ) ;
#10658=DIRECTION ( 'NONE',  ( 0.000000000000000000, 0.5680647467311457088, -0.8229838658936634577 ) ) ;
#10660=DIRECTION ( 'NONE',  ( -0.000000000000000000, 0.9927088740980538617, -0.1205366802553232974 ) ) ;
#10665=EDGE_CURVE ( 'NONE', #49241, #19447, #15813, .T. ) ;
#10669=EDGE_LOOP ( 'NONE', ( #41049, #27759, #43126, #35745 ) ) ;
#10671=VERTEX_POINT ( 'NONE', #8423 ) ;
#10672=EDGE_CURVE ( 'NONE', #4273, #4514, #39944, .T. ) ;
#10675=EDGE_LOOP ( 'NONE', ( #11925, #34064, #49511, #44492 ) ) ;
#10682=FACE_OUTER_BOUND ( 'NONE', #38413, .T. ) ;
#10690=FACE_OUTER_BOUND ( 'NONE', #41167, .T. ) ;
#10692=CARTESIAN_POINT ( 'NONE',  ( -330.4913330509368166, -79.66942718702547666, -39.49849221029252533 ) ) ;
#10697=CARTESIAN_POINT ( 'NONE',  ( -330.4913330509368166, -145.2430625708868206, 55.92172413327848801 ) ) ;
#10701=VECTOR ( 'NONE', #37010, 1000.000000000000000 ) ;
#10704=AXIS2_PLACEMENT_3D ( 'NONE', #25995, #26240, #42018 ) ;
#10705=CARTESIAN_POINT ( 'NONE',  ( -336.3521761649654422, -91.32752733096738496, -49.48329383994654052 ) ) ;
#10715=CARTESIAN_POINT ( 'NONE',  ( -339.1964088526558498, -175.5095439275173135, 27.86139516340941213 ) ) ;
#10719=AXIS2_PLACEMENT_3D ( 'NONE', #16202, #11731, #51187 ) ;
#10721=CARTESIAN_POINT ( 'NONE',  ( -339.1964088526558498, -143.9541802141672235, -55.34326076196065003 ) ) ;
#10723=CARTESIAN_POINT ( 'NONE',  ( -332.3517673607765914, -64.66963335249506883, 11.78931550685348206 ) ) ;
#10724=VECTOR ( 'NONE', #42579, 1000.000000000000000 ) ;
#10728=VECTOR ( 'NONE', #46262, 1000.000000000000227 ) ;
#10729=DIRECTION ( 'NONE',  ( 1.000000000000000000, 3.091579882402590330E-17, -8.151826190875920009E-17 ) ) ;
#10730=ORIENTED_EDGE ( 'NONE', *, *, #1582, .T. ) ;
#10735=CARTESIAN_POINT ( 'NONE',  ( -336.3521761649654422, -161.4024510877913485, 45.24454186338643780 ) ) ;
#10736=ORIENTED_EDGE ( 'NONE', *, *, #30442, .T. ) ;
#10745=EDGE_LOOP ( 'NONE', ( #19087, #30005, #11251, #4545 ) ) ;
#10752=EDGE_CURVE ( 'NONE', #26038, #32799, #39438, .T. ) ;
#10753=VECTOR ( 'NONE', #16320, 999.9999999999998863 ) ;
#10754=EDGE_CURVE ( 'NONE', #41126, #35288, #8685, .T. ) ;
#10774=VERTEX_POINT ( 'NONE', #41512 ) ;
#10776=CIRCLE ( 'NONE', #49397, 15.24495751795539000 ) ;
#10783=CARTESIAN_POINT ( 'NONE',  ( -339.1964088526558498, -181.8741440471346493, 13.87297036558423002 ) ) ;
#10785=VECTOR ( 'NONE', #31032, 999.9999999999998863 ) ;
#10788=CARTESIAN_POINT ( 'NONE',  ( -336.3521761649654422, -65.58448481710581746, 11.56382487286456140 ) ) ;
#10789=CARTESIAN_POINT ( 'NONE',  ( -336.3521761649654422, -136.0347666902908372, 57.67619951860663718 ) ) ;
#10790=PLANE ( 'NONE',  #1950 ) ;
#10791=VERTEX_POINT ( 'NONE', #13669 ) ;
#10792=CIRCLE ( 'NONE', #51106, 60.00000000000000000 ) ;
#10794=DIRECTION ( 'NONE',  ( -1.000000000000000000, 5.928974370888818045E-15, -8.589602288500893078E-15 ) ) ;
#10800=DIRECTION ( 'NONE',  ( 0.000000000000000000, 0.9350162426854194964, 0.3546048870425235200 ) ) ;
#10804=DIRECTION ( 'NONE',  ( -0.000000000000000000, 0.7485107481710999711, -0.6631226582407964143 ) ) ;
#10805=CARTESIAN_POINT ( 'NONE',  ( -330.4913330509368166, -71.49045607248213230, 27.86139516340826461 ) ) ;
#10808=VECTOR ( 'NONE', #8195, 1000.000000000000000 ) ;
#10814=ADVANCED_FACE ( 'NONE', ( #5539 ), #29177, .T. ) ;
#10815=EDGE_CURVE ( 'NONE', #5724, #7178, #45230, .T. ) ;
#10816=EDGE_CURVE ( 'NONE', #3747, #1163, #804, .T. ) ;
#10820=PLANE ( 'NONE',  #11708 ) ;
#10822=CIRCLE ( 'NONE', #4119, 60.00000000000000000 ) ;
#10824=LINE ( 'NONE', #3201, #49294 ) ;
#10826=EDGE_CURVE ( 'NONE', #24446, #27872, #5811, .T. ) ;
#10831=CARTESIAN_POINT ( 'NONE',  ( -305.0000000000000568, -179.0013928959018301, 22.79463504017430253 ) ) ;
#10835=ORIENTED_EDGE ( 'NONE', *, *, #10136, .F. ) ;
#10838=VERTEX_POINT ( 'NONE', #1590 ) ;
#10844=PLANE ( 'NONE',  #50033 ) ;
#10846=ORIENTED_EDGE ( 'NONE', *, *, #26231, .F. ) ;
#10851=VERTEX_POINT ( 'NONE', #29689 ) ;
#10856=AXIS2_PLACEMENT_3D ( 'NONE', #26446, #42754, #1765 ) ;
#10857=DIRECTION ( 'NONE',  ( 0.000000000000000000, 0.4647231720437664526, -0.8854560256532110207 ) ) ;
#10858=DIRECTION ( 'NONE',  ( -1.000000000000000000, 0.000000000000000000, 0.000000000000000000 ) ) ;
#10861=CARTESIAN_POINT ( 'NONE',  ( 0.000000000000000000, -137.6196241929661710, -57.28556722813703317 ) ) ;
#10862=CARTESIAN_POINT ( 'NONE',  ( -330.4913330509368166, -123.5000000000000284, 0.000000000000000000 ) ) ;
#10864=DIRECTION ( 'NONE',  ( 0.000000000000000000, 0.000000000000000000, 1.000000000000000000 ) ) ;
#10867=DIRECTION ( 'NONE',  ( 0.000000000000000000, -0.7485107481710953081, 0.6631226582408016323 ) ) ;
#10869=CARTESIAN_POINT ( 'NONE',  ( -305.0000000000000568, -182.8437365148560616, 8.849911663702917153 ) ) ;
#10871=ORIENTED_EDGE ( 'NONE', *, *, #17325, .T. ) ;
#10872=FACE_OUTER_BOUND ( 'NONE', #39425, .T. ) ;
#10873=VERTEX_POINT ( 'NONE', #46768 ) ;
#10879=EDGE_CURVE ( 'NONE', #42079, #45025, #14975, .T. ) ;
#10881=CARTESIAN_POINT ( 'NONE',  ( -490.0000000000001137, -168.5000000000000284, -14.36509618646847386 ) ) ;
#10885=CARTESIAN_POINT ( 'NONE',  ( -339.1964088526558498, -175.5095439275173135, 27.86139516340941213 ) ) ;
#10886=DIRECTION ( 'NONE',  ( 0.000000000000000000, -0.5680647467311485954, 0.8229838658936613482 ) ) ;
#10889=EDGE_CURVE ( 'NONE', #7181, #34020, #23107, .T. ) ;
#10894=LINE ( 'NONE', #30590, #44993 ) ;
#10898=DIRECTION ( 'NONE',  ( -0.000000000000000000, 0.7485107481710999711, -0.6631226582407964143 ) ) ;
#10902=CARTESIAN_POINT ( 'NONE',  ( -330.4913330509368166, -84.75001853787871653, -44.49369547121542467 ) ) ;
#10905=FACE_OUTER_BOUND ( 'NONE', #24574, .T. ) ;
#10906=ORIENTED_EDGE ( 'NONE', *, *, #44901, .T. ) ;
#10908=EDGE_CURVE ( 'NONE', #11338, #5960, #46509, .T. ) ;
#10911=EDGE_LOOP ( 'NONE', ( #28213, #43926, #28689, #14123 ) ) ;
#10917=CARTESIAN_POINT ( 'NONE',  ( -339.1964088526558498, -167.3305728129742249, 39.49849221029288060 ) ) ;
#10919=ADVANCED_FACE ( 'NONE', ( #28058 ), #47289, .F. ) ;
#10920=ADVANCED_FACE ( 'NONE', ( #4173 ), #39375, .F. ) ;
#10921=CARTESIAN_POINT ( 'NONE',  ( -336.3521761649654422, -97.52665284734005979, -53.00046796564681983 ) ) ;
#10924=DIRECTION ( 'NONE',  ( 1.000000000000000000, 0.000000000000000000, 0.000000000000000000 ) ) ;
#10930=DIRECTION ( 'NONE',  ( 0.000000000000000000, 0.000000000000000000, -1.000000000000000000 ) ) ;
#10932=LINE ( 'NONE', #31678, #50307 ) ;
#10933=CARTESIAN_POINT ( 'NONE',  ( -339.1964088526558498, -108.8949048983213004, -57.16590939599337418 ) ) ;
#10940=EDGE_LOOP ( 'NONE', ( #31120, #51875, #6789, #23015 ) ) ;
#10942=VECTOR ( 'NONE', #12649, 1000.000000000000000 ) ;
#10943=VERTEX_POINT ( 'NONE', #19410 ) ;
#10944=EDGE_CURVE ( 'NONE', #16640, #8493, #16253, .T. ) ;
#10962=ORIENTED_EDGE ( 'NONE', *, *, #42456, .F. ) ;
#10964=VERTEX_POINT ( 'NONE', #35432 ) ;
#10971=LINE ( 'NONE', #23334, #2185 ) ;
#10982=CARTESIAN_POINT ( 'NONE',  ( -305.0000000000000568, -183.4979166304964622, -0.4999999999999573119 ) ) ;
#10984=ORIENTED_EDGE ( 'NONE', *, *, #36263, .T. ) ;
#10985=CARTESIAN_POINT ( 'NONE',  ( -305.0000000000000568, -158.9146170832377720, -48.43351006119259949 ) ) ;
#10987=DIRECTION ( 'NONE',  ( 1.000000000000000000, -0.000000000000000000, 0.000000000000000000 ) ) ;
#10996=VERTEX_POINT ( 'NONE', #27802 ) ;
#10999=DIRECTION ( 'NONE',  ( -0.000000000000000000, -0.5680647467311485954, 0.8229838658936613482 ) ) ;
#11005=EDGE_CURVE ( 'NONE', #46482, #50353, #43836, .T. ) ;
#11008=DIRECTION ( 'NONE',  ( -1.000000000000000000, 0.000000000000000000, 0.000000000000000000 ) ) ;
#11009=ORIENTED_EDGE ( 'NONE', *, *, #22749, .T. ) ;
#11010=LINE ( 'NONE', #28067, #5758 ) ;
#11016=FACE_OUTER_BOUND ( 'NONE', #32664, .T. ) ;
#11023=DIRECTION ( 'NONE',  ( 0.000000000000000000, 0.000000000000000000, 1.000000000000000000 ) ) ;
#11025=LINE ( 'NONE', #27053, #13976 ) ;
#11026=ORIENTED_EDGE ( 'NONE', *, *, #6342, .F. ) ;
#11029=CARTESIAN_POINT ( 'NONE',  ( -305.0000000000000568, -72.67320051506121104, 31.88473700876054551 ) ) ;
#11030=DIRECTION ( 'NONE',  ( -0.000000000000000000, 0.2393156642875652051, 0.9709418174260502354 ) ) ;
#11036=VECTOR ( 'NONE', #46670, 1000.000000000000000 ) ;
#11037=DIRECTION ( 'NONE',  ( -1.000000000000000000, -0.000000000000000000, -0.000000000000000000 ) ) ;
#11039=LINE ( 'NONE', #35465, #37524 ) ;
#11042=EDGE_CURVE ( 'NONE', #44752, #23503, #27559, .T. ) ;
#11046=LINE ( 'NONE', #38397, #10303 ) ;
#11047=CARTESIAN_POINT ( 'NONE',  ( -339.1964088526558498, -75.22798428563991990, -33.92731199008514409 ) ) ;
#11050=PLANE ( 'NONE',  #38601 ) ;
#11054=EDGE_LOOP ( 'NONE', ( #12678, #5379, #22373, #34080 ) ) ;
#11055=ORIENTED_EDGE ( 'NONE', *, *, #36982, .T. ) ;
#11058=VERTEX_POINT ( 'NONE', #40160 ) ;
#11060=DIRECTION ( 'NONE',  ( -1.000000000000000000, 0.000000000000000000, 0.000000000000000000 ) ) ;
#11061=ORIENTED_EDGE ( 'NONE', *, *, #44942, .T. ) ;
#11063=LINE ( 'NONE', #32074, #19351 ) ;
#11064=CARTESIAN_POINT ( 'NONE',  ( -336.3521761649654422, -145.9479049231020440, -54.58714071513102795 ) ) ;
#11068=CARTESIAN_POINT ( 'NONE',  ( -332.3517673607765914, -126.1322888500942554, -59.94223098458773080 ) ) ;
#11069=ORIENTED_EDGE ( 'NONE', *, *, #12757, .F. ) ;
#11074=FACE_OUTER_BOUND ( 'NONE', #13223, .T. ) ;
#11080=CARTESIAN_POINT ( 'NONE',  ( -336.3521761649653854, -156.2279223070262049, 50.28800156563451651 ) ) ;
#11082=CARTESIAN_POINT ( 'NONE',  ( -336.3521761649654422, -113.7752393642576720, 58.25253621232167944 ) ) ;
#11083=DIRECTION ( 'NONE',  ( -0.000000000000000000, 0.000000000000000000, 1.000000000000000000 ) ) ;
#11088=DIRECTION ( 'NONE',  ( 1.000000000000000000, -0.000000000000000000, -0.000000000000000000 ) ) ;
#11090=CARTESIAN_POINT ( 'NONE',  ( -339.1964088526558498, -71.49045607248213230, 27.86139516340826106 ) ) ;
#11092=ORIENTED_EDGE ( 'NONE', *, *, #42403, .T. ) ;
#11096=AXIS2_PLACEMENT_3D ( 'NONE', #678, #16727, #8808 ) ;
#11105=CARTESIAN_POINT ( 'NONE',  ( -336.3521761649654422, -113.7752393642576720, 58.25253621232167944 ) ) ;
#11106=DIRECTION ( 'NONE',  ( 0.000000000000000000, 0.000000000000000000, -1.000000000000000000 ) ) ;
#11108=LINE ( 'NONE', #27395, #16967 ) ;
#11114=EDGE_CURVE ( 'NONE', #50694, #4146, #32860, .T. ) ;
#11120=CARTESIAN_POINT ( 'NONE',  ( -332.3517673607765914, -155.6724726690323450, 49.48329383994676078 ) ) ;
#11121=EDGE_LOOP ( 'NONE', ( #45948, #12104, #49961, #47617 ) ) ;
#11124=EDGE_CURVE ( 'NONE', #32868, #1251, #41011, .T. ) ;
#11126=CARTESIAN_POINT ( 'NONE',  ( -305.0000000000000568, -78.92247586332004516, -40.16023333900979964 ) ) ;
#11136=CARTESIAN_POINT ( 'NONE',  ( -365.0000000000001137, -78.50000000000002842, 0.000000000000000000 ) ) ;
#11143=VERTEX_POINT ( 'NONE', #37065 ) ;
#11146=DIRECTION ( 'NONE',  ( -1.000000000000000000, 0.000000000000000000, -0.000000000000000000 ) ) ;
#11150=VERTEX_POINT ( 'NONE', #28651 ) ;
#11153=EDGE_LOOP ( 'NONE', ( #29674, #39881, #14988, #1193 ) ) ;
#11154=DIRECTION ( 'NONE',  ( 1.000000000000000000, 0.000000000000000000, 0.000000000000000000 ) ) ;
#11158=DIRECTION ( 'NONE',  ( 1.043714542225393381E-14, -0.7485107481711024136, -0.6631226582407937498 ) ) ;
#11159=ADVANCED_FACE ( 'NONE', ( #40740 ), #29185, .F. ) ;
#11160=DIRECTION ( 'NONE',  ( -1.000000000000000000, -0.000000000000000000, -0.000000000000000000 ) ) ;
#11165=AXIS2_PLACEMENT_3D ( 'NONE', #26173, #18563, #22239 ) ;
#11166=EDGE_CURVE ( 'NONE', #2008, #8829, #36820, .T. ) ;
#11173=ORIENTED_EDGE ( 'NONE', *, *, #23536, .F. ) ;
#11177=EDGE_CURVE ( 'NONE', #31178, #28257, #21046, .T. ) ;
#11181=ORIENTED_EDGE ( 'NONE', *, *, #23771, .F. ) ;
#11184=CARTESIAN_POINT ( 'NONE',  ( -339.1964088526558498, -102.1108035431478811, -54.98865587491830809 ) ) ;
#11192=VERTEX_POINT ( 'NONE', #29697 ) ;
#11195=EDGE_LOOP ( 'NONE', ( #48481, #43948, #44928, #5191 ) ) ;
#11202=EDGE_CURVE ( 'NONE', #29300, #11668, #6581, .T. ) ;
#11208=ORIENTED_EDGE ( 'NONE', *, *, #26181, .F. ) ;
#11212=DIRECTION ( 'NONE',  ( 0.000000000000000000, -1.892005071132037688E-13, 1.000000000000000000 ) ) ;
#11224=EDGE_CURVE ( 'NONE', #50838, #3877, #22075, .T. ) ;
#11226=LINE ( 'NONE', #35928, #10282 ) ;
#11228=CARTESIAN_POINT ( 'NONE',  ( -336.3521761649654422, -142.8954717479169574, 55.74477592174805096 ) ) ;
#11238=LINE ( 'NONE', #10985, #26255 ) ;
#11249=ORIENTED_EDGE ( 'NONE', *, *, #40496, .F. ) ;
#11251=ORIENTED_EDGE ( 'NONE', *, *, #22048, .F. ) ;
#11252=DIRECTION ( 'NONE',  ( -0.000000000000000000, 0.9927088740980556381, 0.1205366802553095307 ) ) ;
#11254=VECTOR ( 'NONE', #31076, 1000.000000000000000 ) ;
#11261=CARTESIAN_POINT ( 'NONE',  ( -330.4913330509368166, -162.9984922102920848, 43.83057281297495678 ) ) ;
#11262=ORIENTED_EDGE ( 'NONE', *, *, #25374, .F. ) ;
#11263=CARTESIAN_POINT ( 'NONE',  ( -339.1964088526558498, -130.1153096980153236, -58.63009191191284941 ) ) ;
#11268=CARTESIAN_POINT ( 'NONE',  ( -330.4913330509368166, -79.66942718702547666, -39.49849221029252533 ) ) ;
#11272=LINE ( 'NONE', #42300, #40439 ) ;
#11278=CARTESIAN_POINT ( 'NONE',  ( -339.1964088526558498, -144.8891964568517778, 54.98865587491845730 ) ) ;
#11280=EDGE_CURVE ( 'NONE', #6134, #39742, #13678, .T. ) ;
#11281=EDGE_CURVE ( 'NONE', #4514, #5217, #17501, .T. ) ;
#11287=CARTESIAN_POINT ( 'NONE',  ( -332.3517673607765914, -128.9912765084839066, 58.76657425099337928 ) ) ;
#11288=DIRECTION ( 'NONE',  ( 1.000000000000000000, 0.000000000000000000, 0.000000000000000000 ) ) ;
#11289=AXIS2_PLACEMENT_3D ( 'NONE', #30722, #6056, #46267 ) ;
#11301=ADVANCED_FACE ( 'NONE', ( #6312 ), #14714, .F. ) ;
#11308=EDGE_LOOP ( 'NONE', ( #36226, #35708, #36346, #8273 ) ) ;
#11311=LINE ( 'NONE', #37051, #50231 ) ;
#11313=PLANE ( 'NONE',  #22819 ) ;
#11318=DIRECTION ( 'NONE',  ( -0.000000000000000000, -0.9709418174260502354, 0.2393156642875652051 ) ) ;
#11323=ORIENTED_EDGE ( 'NONE', *, *, #42027, .T. ) ;
#11324=CARTESIAN_POINT ( 'NONE',  ( -336.3521761649654422, -70.49953203435293858, 25.97334715265942151 ) ) ;
#11327=PLANE ( 'NONE',  #15725 ) ;
#11328=CARTESIAN_POINT ( 'NONE',  ( -336.3521761649654422, -92.15051119686104641, -50.05135858667769355 ) ) ;
#11329=FACE_OUTER_BOUND ( 'NONE', #13883, .T. ) ;
#11333=EDGE_CURVE ( 'NONE', #30259, #8199, #49943, .T. ) ;
#11335=ORIENTED_EDGE ( 'NONE', *, *, #42160, .T. ) ;
#11337=CARTESIAN_POINT ( 'NONE',  ( 0.000000000000000000, -150.9186671505826212, -52.24190551353930090 ) ) ;
#11338=VERTEX_POINT ( 'NONE', #29966 ) ;
#11339=AXIS2_PLACEMENT_3D ( 'NONE', #5478, #1249, #1522 ) ;
#11343=ORIENTED_EDGE ( 'NONE', *, *, #34142, .T. ) ;
#11348=VECTOR ( 'NONE', #44625, 1000.000000000000000 ) ;
#11349=EDGE_LOOP ( 'NONE', ( #9887, #15143, #18195, #36749 ) ) ;
#11355=LINE ( 'NONE', #27388, #3396 ) ;
#11360=PLANE ( 'NONE',  #32874 ) ;
#11361=ADVANCED_FACE ( 'NONE', ( #7085 ), #31776, .F. ) ;
#11362=CARTESIAN_POINT ( 'NONE',  ( -305.0000000000000568, -179.4217241332784454, -21.74306257088699113 ) ) ;
#11364=ORIENTED_EDGE ( 'NONE', *, *, #2860, .F. ) ;
#11367=ORIENTED_EDGE ( 'NONE', *, *, #32725, .T. ) ;
#11375=DIRECTION ( 'NONE',  ( -0.000000000000000000, 0.6631226582407937498, -0.7485107481711024136 ) ) ;
#11380=LINE ( 'NONE', #11126, #3967 ) ;
#11383=ORIENTED_EDGE ( 'NONE', *, *, #36103, .F. ) ;
#11386=CARTESIAN_POINT ( 'NONE',  ( -332.3517673607765914, -146.8829211657874794, -54.23253582808848705 ) ) ;
#11387=CARTESIAN_POINT ( 'NONE',  ( -339.1964088526558498, -151.3613951634084742, 52.00954392751779665 ) ) ;
#11388=DIRECTION ( 'NONE',  ( 0.000000000000000000, 0.000000000000000000, 1.000000000000000000 ) ) ;
#11391=EDGE_CURVE ( 'NONE', #8199, #46931, #38872, .T. ) ;
#11396=AXIS2_PLACEMENT_3D ( 'NONE', #27588, #7615, #39651 ) ;
#11398=CARTESIAN_POINT ( 'NONE',  ( -339.1964088526558498, -123.5000000000000284, 0.000000000000000000 ) ) ;
#11399=DIRECTION ( 'NONE',  ( 0.000000000000000000, 0.000000000000000000, 1.000000000000000000 ) ) ;
#11400=ORIENTED_EDGE ( 'NONE', *, *, #44901, .F. ) ;
#11403=AXIS2_PLACEMENT_3D ( 'NONE', #34742, #50285, #2689 ) ;
#11404=CARTESIAN_POINT ( 'NONE',  ( -330.4913330509368166, -157.4273119900852578, -48.27201571436002325 ) ) ;
#11406=ORIENTED_EDGE ( 'NONE', *, *, #40895, .F. ) ;
#11407=EDGE_CURVE ( 'NONE', #32138, #29000, #11010, .T. ) ;
#11410=ORIENTED_EDGE ( 'NONE', *, *, #34001, .T. ) ;
#11415=ORIENTED_EDGE ( 'NONE', *, *, #12162, .T. ) ;
#11418=FACE_OUTER_BOUND ( 'NONE', #27877, .T. ) ;
#11419=FACE_OUTER_BOUND ( 'NONE', #33409, .T. ) ;
#11420=VECTOR ( 'NONE', #13174, 1000.000000000000114 ) ;
#11421=CARTESIAN_POINT ( 'NONE',  ( -305.0000000000000568, -152.8183901354257159, -52.34913561719022113 ) ) ;
#11422=DIRECTION ( 'NONE',  ( 0.000000000000000000, 0.4647231720437604574, -0.8854560256532141294 ) ) ;
#11423=AXIS2_PLACEMENT_3D ( 'NONE', #15617, #42943, #27690 ) ;
#11426=CARTESIAN_POINT ( 'NONE',  ( -339.1964088526558498, -182.1300919119128423, 6.615309698015510165 ) ) ;
#11427=PLANE ( 'NONE',  #42191 ) ;
#11428=ORIENTED_EDGE ( 'NONE', *, *, #1188, .T. ) ;
#11433=AXIS2_PLACEMENT_3D ( 'NONE', #34964, #366, #16422 ) ;
#11437=ORIENTED_EDGE ( 'NONE', *, *, #7030, .F. ) ;
#11441=CARTESIAN_POINT ( 'NONE',  ( -336.3521761649654422, -146.8829211657874794, -54.23253582808848705 ) ) ;
#11442=ORIENTED_EDGE ( 'NONE', *, *, #40496, .T. ) ;
#11448=AXIS2_PLACEMENT_3D ( 'NONE', #42059, #18156, #48922 ) ;
#11451=CARTESIAN_POINT ( 'NONE',  ( -305.0000000000000568, -64.87442053112221174, 12.76876783163883111 ) ) ;
#11452=AXIS2_PLACEMENT_3D ( 'NONE', #17188, #49250, #45054 ) ;
#11455=EDGE_CURVE ( 'NONE', #46710, #2495, #39384, .T. ) ;
#11459=EDGE_CURVE ( 'NONE', #17674, #30731, #35704, .T. ) ;
#11460=VECTOR ( 'NONE', #30535, 999.9999999999998863 ) ;
#11462=EDGE_LOOP ( 'NONE', ( #28685, #24706, #15311, #17986 ) ) ;
#11464=ORIENTED_EDGE ( 'NONE', *, *, #30117, .T. ) ;
#11466=ADVANCED_FACE ( 'NONE', ( #19418 ), #43078, .F. ) ;
#11471=CARTESIAN_POINT ( 'NONE',  ( -339.1964088526558498, -123.5000000000000284, 0.000000000000000000 ) ) ;
#11472=VERTEX_POINT ( 'NONE', #39633 ) ;
#11474=DIRECTION ( 'NONE',  ( -0.000000000000000000, -3.491481338843133355E-15, -1.000000000000000000 ) ) ;
#11475=ORIENTED_EDGE ( 'NONE', *, *, #18134, .T. ) ;
#11476=EDGE_CURVE ( 'NONE', #9197, #51141, #24195, .T. ) ;
#11481=VECTOR ( 'NONE', #2461, 1000.000000000000000 ) ;
#11483=DIRECTION ( 'NONE',  ( 0.000000000000000000, -0.8229838658936575735, -0.5680647467311540355 ) ) ;
#11484=DIRECTION ( 'NONE',  ( 0.000000000000000000, 0.000000000000000000, 1.000000000000000000 ) ) ;
#11489=EDGE_LOOP ( 'NONE', ( #1173, #41014, #22017, #11897 ) ) ;
#11494=AXIS2_PLACEMENT_3D ( 'NONE', #41637, #28765, #33242 ) ;
#11495=AXIS2_PLACEMENT_3D ( 'NONE', #39748, #3765, #19794 ) ;
#11497=VECTOR ( 'NONE', #45679, 1000.000000000000000 ) ;
#11498=VECTOR ( 'NONE', #12119, 1000.000000000000000 ) ;
#11501=DIRECTION ( 'NONE',  ( 0.000000000000000000, -0.7485107481711069655, -0.6631226582407885317 ) ) ;
#11510=ORIENTED_EDGE ( 'NONE', *, *, #4013, .T. ) ;
#11517=CARTESIAN_POINT ( 'NONE',  ( -339.1964088526558498, -175.9742670995615015, -26.97593913775538965 ) ) ;
#11522=ADVANCED_FACE ( 'NONE', ( #12307 ), #8890, .T. ) ;
#11525=ORIENTED_EDGE ( 'NONE', *, *, #22467, .F. ) ;
#11527=DIRECTION ( 'NONE',  ( -0.000000000000000000, 0.6631226582408039638, 0.7485107481710934207 ) ) ;
#11529=VECTOR ( 'NONE', #49809, 1000.000000000000000 ) ;
#11530=VECTOR ( 'NONE', #47614, 1000.000000000000000 ) ;
#11536=DIRECTION ( 'NONE',  ( -8.718379230999705894E-17, 0.9927088740980535286, -0.1205366802553268502 ) ) ;
#11543=LINE ( 'NONE', #7088, #42590 ) ;
#11544=EDGE_LOOP ( 'NONE', ( #25167, #37668, #34303, #658 ) ) ;
#11546=VECTOR ( 'NONE', #40215, 1000.000000000000000 ) ;
#11547=DIRECTION ( 'NONE',  ( 0.000000000000000000, -0.8229838658936613482, -0.5680647467311485954 ) ) ;
#11553=LINE ( 'NONE', #27580, #35889 ) ;
#11554=CARTESIAN_POINT ( 'NONE',  ( -339.1964088526558498, -130.1153096980144426, 58.63009191191295599 ) ) ;
#11562=CARTESIAN_POINT ( 'NONE',  ( -330.4913330509368166, -143.9541802141664562, 55.34326076196094135 ) ) ;
#11563=ORIENTED_EDGE ( 'NONE', *, *, #32035, .T. ) ;
#11566=CARTESIAN_POINT ( 'NONE',  ( -339.1964088526558498, -89.57268800991514013, -48.27201571436026484 ) ) ;
#11576=CARTESIAN_POINT ( 'NONE',  ( -339.1964088526558498, -123.5000000000000284, 0.000000000000000000 ) ) ;
#11578=DIRECTION ( 'NONE',  ( 1.000000000000000000, 0.000000000000000000, 0.000000000000000000 ) ) ;
#11583=EDGE_LOOP ( 'NONE', ( #24303, #20601, #30929, #32213 ) ) ;
#11584=ORIENTED_EDGE ( 'NONE', *, *, #23974, .T. ) ;
#11585=ORIENTED_EDGE ( 'NONE', *, *, #9246, .F. ) ;
#11591=DIRECTION ( 'NONE',  ( -0.000000000000000000, 0.000000000000000000, 1.000000000000000000 ) ) ;
#11592=DIRECTION ( 'NONE',  ( 0.000000000000000000, 0.5680647467311510379, -0.8229838658936596829 ) ) ;
#11593=VECTOR ( 'NONE', #8188, 1000.000000000000000 ) ;
#11596=ORIENTED_EDGE ( 'NONE', *, *, #34978, .F. ) ;
#11597=AXIS2_PLACEMENT_3D ( 'NONE', #8321, #4909, #16470 ) ;
#11598=AXIS2_PLACEMENT_3D ( 'NONE', #42870, #7131, #10556 ) ;
#11603=EDGE_LOOP ( 'NONE', ( #5274, #37699, #12409, #36095 ) ) ;
#11604=LINE ( 'NONE', #35502, #37497 ) ;
#11605=CARTESIAN_POINT ( 'NONE',  ( -336.3521761649654422, -146.8829211657874794, -54.23253582808848705 ) ) ;
#11607=DIRECTION ( 'NONE',  ( -0.000000000000000000, -0.6631226582407911962, 0.7485107481711046340 ) ) ;
#11608=VERTEX_POINT ( 'NONE', #37269 ) ;
#11611=CARTESIAN_POINT ( 'NONE',  ( -332.3517673607765914, -64.15626348514393840, -8.849911663702497933 ) ) ;
#11613=VERTEX_POINT ( 'NONE', #1261 ) ;
#11616=DIRECTION ( 'NONE',  ( 1.000000000000000000, 0.000000000000000000, -0.000000000000000000 ) ) ;
#11618=ORIENTED_EDGE ( 'NONE', *, *, #23709, .F. ) ;
#11621=EDGE_CURVE ( 'NONE', #23503, #31214, #29251, .T. ) ;
#11622=VECTOR ( 'NONE', #13941, 1000.000000000000000 ) ;
#11624=ORIENTED_EDGE ( 'NONE', *, *, #40962, .T. ) ;
#11626=VERTEX_POINT ( 'NONE', #21505 ) ;
#11627=CARTESIAN_POINT ( 'NONE',  ( -332.3517673607765914, -82.50558083279611310, 43.81161486573607533 ) ) ;
#11629=LINE ( 'NONE', #23465, #41138 ) ;
#11630=CARTESIAN_POINT ( 'NONE',  ( -339.1964088526558498, -89.82879061784626629, 49.66134974749640207 ) ) ;
#11635=DIRECTION ( 'NONE',  ( 0.000000000000000000, -0.9350162426854169428, -0.3546048870425300148 ) ) ;
#11644=ORIENTED_EDGE ( 'NONE', *, *, #28632, .T. ) ;
#11645=AXIS2_PLACEMENT_3D ( 'NONE', #51424, #18325, #34584 ) ;
#11651=EDGE_CURVE ( 'NONE', #12334, #38856, #41461, .T. ) ;
#11652=LINE ( 'NONE', #41569, #18574 ) ;
#11657=CIRCLE ( 'NONE', #41029, 10.00000000000000711 ) ;
#11658=PLANE ( 'NONE',  #24980 ) ;
#11660=PLANE ( 'NONE',  #19502 ) ;
#11662=EDGE_LOOP ( 'NONE', ( #13520, #33773, #42104, #12040 ) ) ;
#11663=DIRECTION ( 'NONE',  ( -0.000000000000000000, -0.9709418174260511236, 0.2393156642875615969 ) ) ;
#11664=LINE ( 'NONE', #343, #1308 ) ;
#11665=CARTESIAN_POINT ( 'NONE',  ( -305.0000000000000568, -166.6218737817864621, 41.71934804797023588 ) ) ;
#11666=ORIENTED_EDGE ( 'NONE', *, *, #38071, .T. ) ;
#11668=VERTEX_POINT ( 'NONE', #45956 ) ;
#11674=CARTESIAN_POINT ( 'NONE',  ( -332.3517673607765914, -121.8677111499054320, 59.97779283292990016 ) ) ;
#11675=AXIS2_PLACEMENT_3D ( 'NONE', #14132, #18825, #14638 ) ;
#11676=LINE ( 'NONE', #51623, #10280 ) ;
#11678=EDGE_LOOP ( 'NONE', ( #4255, #31241, #37597, #826 ) ) ;
#11679=PLANE ( 'NONE',  #25892 ) ;
#11682=AXIS2_PLACEMENT_3D ( 'NONE', #28311, #8352, #45399 ) ;
#11686=CARTESIAN_POINT ( 'NONE',  ( -332.3517673607765914, -176.9651911376907094, -25.08789112700655721 ) ) ;
#11689=VECTOR ( 'NONE', #47423, 1000.000000000000000 ) ;
#11690=ORIENTED_EDGE ( 'NONE', *, *, #49794, .T. ) ;
#11692=ORIENTED_EDGE ( 'NONE', *, *, #10578, .T. ) ;
#11695=EDGE_LOOP ( 'NONE', ( #20421, #35302, #32408, #15975 ) ) ;
#11700=DIRECTION ( 'NONE',  ( -1.000000000000000000, 0.000000000000000000, -0.000000000000000000 ) ) ;
#11703=DIRECTION ( 'NONE',  ( 0.000000000000000000, 0.000000000000000000, 1.000000000000000000 ) ) ;
#11705=EDGE_LOOP ( 'NONE', ( #33753, #1597, #24908, #37722 ) ) ;
#11708=AXIS2_PLACEMENT_3D ( 'NONE', #39189, #47343, #18453 ) ;
#11709=EDGE_CURVE ( 'NONE', #12667, #15472, #50658, .T. ) ;
#11713=VERTEX_POINT ( 'NONE', #2315 ) ;
#11715=ORIENTED_EDGE ( 'NONE', *, *, #14572, .F. ) ;
#11722=EDGE_LOOP ( 'NONE', ( #26985, #30872, #14721, #4242 ) ) ;
#11726=PLANE ( 'NONE',  #38203 ) ;
#11727=EDGE_LOOP ( 'NONE', ( #48651, #27922, #28704, #10580 ) ) ;
#11731=DIRECTION ( 'NONE',  ( -8.718379230999705894E-17, 0.2393156642875582940, 0.9709418174260519008 ) ) ;
#11734=VERTEX_POINT ( 'NONE', #18594 ) ;
#11736=VERTEX_POINT ( 'NONE', #50156 ) ;
#11737=ORIENTED_EDGE ( 'NONE', *, *, #17724, .F. ) ;
#11740=PLANE ( 'NONE',  #24884 ) ;
#11741=DIRECTION ( 'NONE',  ( -1.000000000000000000, 0.000000000000000000, 0.000000000000000000 ) ) ;
#11743=CARTESIAN_POINT ( 'NONE',  ( -336.3521761649654422, -146.8829211657874794, -54.23253582808848705 ) ) ;
#11750=DIRECTION ( 'NONE',  ( -0.000000000000000000, -0.6631226582407885317, 0.7485107481711069655 ) ) ;
#11752=ORIENTED_EDGE ( 'NONE', *, *, #21576, .T. ) ;
#11756=VECTOR ( 'NONE', #7470, 1000.000000000000000 ) ;
#11760=DIRECTION ( 'NONE',  ( 1.000000000000000000, 6.525800561034949817E-17, -5.781354811211897260E-17 ) ) ;
#11763=CARTESIAN_POINT ( 'NONE',  ( -336.3521761649654422, -176.9651911376907094, -25.08789112700655721 ) ) ;
#11766=ORIENTED_EDGE ( 'NONE', *, *, #39576, .F. ) ;
#11768=EDGE_CURVE ( 'NONE', #43264, #3693, #6522, .T. ) ;
#11769=VECTOR ( 'NONE', #48829, 1000.000000000000000 ) ;
#11770=ORIENTED_EDGE ( 'NONE', *, *, #7084, .F. ) ;
#11771=FACE_OUTER_BOUND ( 'NONE', #33769, .T. ) ;
#11772=DIRECTION ( 'NONE',  ( -0.000000000000000000, -0.4647231720437724478, -0.8854560256532078011 ) ) ;
#11782=DIRECTION ( 'NONE',  ( 0.000000000000000000, 0.1205366802553268363, 0.9927088740980534176 ) ) ;
#11788=ORIENTED_EDGE ( 'NONE', *, *, #5697, .F. ) ;
#11790=AXIS2_PLACEMENT_3D ( 'NONE', #40697, #41224, #33360 ) ;
#11792=VERTEX_POINT ( 'NONE', #18843 ) ;
#11799=EDGE_LOOP ( 'NONE', ( #20755, #28912, #49451, #31665 ) ) ;
#11801=CARTESIAN_POINT ( 'NONE',  ( -339.1964088526558498, -130.1153096980144426, 58.63009191191295599 ) ) ;
#11802=EDGE_CURVE ( 'NONE', #41880, #13092, #23564, .T. ) ;
#11806=LINE ( 'NONE', #52040, #48340 ) ;
#11808=DIRECTION ( 'NONE',  ( 1.000000000000000000, -0.000000000000000000, -0.000000000000000000 ) ) ;
#11809=CARTESIAN_POINT ( 'NONE',  ( -336.3521761649653854, -146.2946350401741711, -55.50139289590185854 ) ) ;
#11822=VERTEX_POINT ( 'NONE', #31443 ) ;
#11829=EDGE_CURVE ( 'NONE', #18286, #30079, #46941, .T. ) ;
#11830=ORIENTED_EDGE ( 'NONE', *, *, #32291, .F. ) ;
#11842=DIRECTION ( 'NONE',  ( 0.000000000000000000, 0.000000000000000000, 1.000000000000000000 ) ) ;
#11845=ORIENTED_EDGE ( 'NONE', *, *, #45396, .F. ) ;
#11847=CARTESIAN_POINT ( 'NONE',  ( -332.3517673607765914, -64.31210272782786319, -9.838334030657643225 ) ) ;
#11848=FACE_OUTER_BOUND ( 'NONE', #20271, .T. ) ;
#11856=DIRECTION ( 'NONE',  ( 1.000000000000000000, 0.000000000000000000, -0.000000000000000000 ) ) ;
#11859=VERTEX_POINT ( 'NONE', #51440 ) ;
#11862=CARTESIAN_POINT ( 'NONE',  ( -330.4913330509368166, -162.9984922102926532, -43.83057281297441676 ) ) ;
#11863=CIRCLE ( 'NONE', #38690, 60.00000000000000000 ) ;
#11865=CARTESIAN_POINT ( 'NONE',  ( -336.3521761649654422, -92.15051119686104641, -50.05135858667769355 ) ) ;
#11869=ADVANCED_FACE ( 'NONE', ( #43544 ), #7543, .F. ) ;
#11871=CARTESIAN_POINT ( 'NONE',  ( -332.3517673607765914, -140.1754235130667610, -56.65561927338005432 ) ) ;
#11872=DIRECTION ( 'NONE',  ( -0.000000000000000000, -0.9350162426854169428, -0.3546048870425300148 ) ) ;
#11875=EDGE_CURVE ( 'NONE', #24196, #37502, #40348, .T. ) ;
#11877=EDGE_CURVE ( 'NONE', #10455, #21654, #19210, .T. ) ;
#11880=CARTESIAN_POINT ( 'NONE',  ( -339.1964088526558498, -131.1080185721133660, -58.50955523165751515 ) ) ;
#11890=CARTESIAN_POINT ( 'NONE',  ( -336.3521761649654422, -65.24746378767824240, -9.724760635741734660 ) ) ;
#11891=DIRECTION ( 'NONE',  ( 0.000000000000000000, 0.3546048870425363986, 0.9350162426854146114 ) ) ;
#11897=ORIENTED_EDGE ( 'NONE', *, *, #36441, .T. ) ;
#11899=AXIS2_PLACEMENT_3D ( 'NONE', #4797, #20822, #25530 ) ;
#11900=ORIENTED_EDGE ( 'NONE', *, *, #52003, .F. ) ;
#11903=LINE ( 'NONE', #43967, #44256 ) ;
#11906=ORIENTED_EDGE ( 'NONE', *, *, #11651, .T. ) ;
#11912=ORIENTED_EDGE ( 'NONE', *, *, #18868, .F. ) ;
#11913=ORIENTED_EDGE ( 'NONE', *, *, #32353, .F. ) ;
#11915=ORIENTED_EDGE ( 'NONE', *, *, #41660, .F. ) ;
#11916=VECTOR ( 'NONE', #23496, 1000.000000000000000 ) ;
#11919=EDGE_LOOP ( 'NONE', ( #46264, #49208, #28591, #24805 ) ) ;
#11920=CARTESIAN_POINT ( 'NONE',  ( -330.4913330509368166, -150.9396941197148294, 53.35787839313412206 ) ) ;
#11923=EDGE_LOOP ( 'NONE', ( #20276, #47211, #2945, #19308 ) ) ;
#11925=ORIENTED_EDGE ( 'NONE', *, *, #1563, .T. ) ;
#11928=CARTESIAN_POINT ( 'NONE',  ( -339.1964088526558498, -75.22798428563991990, -33.92731199008514409 ) ) ;
#11930=ORIENTED_EDGE ( 'NONE', *, *, #32416, .T. ) ;
#11933=FACE_OUTER_BOUND ( 'NONE', #8577, .T. ) ;
#11934=LINE ( 'NONE', #32174, #40809 ) ;
#11938=VERTEX_POINT ( 'NONE', #13025 ) ;
#11939=FACE_OUTER_BOUND ( 'NONE', #6431, .T. ) ;
#11942=FACE_OUTER_BOUND ( 'NONE', #37826, .T. ) ;
#11943=CARTESIAN_POINT ( 'NONE',  ( -365.0000000000001137, -78.50000000000002842, -5.000000000000001776 ) ) ;
#11945=ORIENTED_EDGE ( 'NONE', *, *, #39691, .T. ) ;
#11946=LINE ( 'NONE', #9327, #42480 ) ;
#11948=AXIS2_PLACEMENT_3D ( 'NONE', #47942, #43989, #3785 ) ;
#11951=VECTOR ( 'NONE', #8576, 1000.000000000000000 ) ;
#11955=DIRECTION ( 'NONE',  ( 0.000000000000000000, -6.568819562365509110E-14, 1.000000000000000000 ) ) ;
#11957=ORIENTED_EDGE ( 'NONE', *, *, #47394, .F. ) ;
#11958=DIRECTION ( 'NONE',  ( -1.000000000000000000, 0.000000000000000000, 0.000000000000000000 ) ) ;
#11960=CARTESIAN_POINT ( 'NONE',  ( -339.1964088526558498, -123.5000000000000284, 0.000000000000000000 ) ) ;
#11964=EDGE_CURVE ( 'NONE', #50728, #5970, #28014, .T. ) ;
#11967=DIRECTION ( 'NONE',  ( -0.000000000000000000, -0.2393156642875482742, 0.9709418174260544543 ) ) ;
#11969=FACE_BOUND ( 'NONE', #36564, .T. ) ;
#11976=DIRECTION ( 'NONE',  ( 0.000000000000000000, -0.8854560256532062468, 0.4647231720437755564 ) ) ;
#11982=DIRECTION ( 'NONE',  ( -8.718379230999707126E-17, -0.1205366802553095307, 0.9927088740980556381 ) ) ;
#11983=EDGE_LOOP ( 'NONE', ( #27793, #17115, #25997, #46168 ) ) ;
#11986=ORIENTED_EDGE ( 'NONE', *, *, #14637, .F. ) ;
#11988=EDGE_CURVE ( 'NONE', #38775, #39946, #32746, .T. ) ;
#11991=CIRCLE ( 'NONE', #30454, 60.00000000000000000 ) ;
#11993=LINE ( 'NONE', #40116, #23205 ) ;
#11997=ADVANCED_FACE ( 'NONE', ( #48001 ), #28280, .F. ) ;
#11999=EDGE_LOOP ( 'NONE', ( #30901, #36558, #3917, #33661 ) ) ;
#12000=LINE ( 'NONE', #431, #38080 ) ;
#12003=ORIENTED_EDGE ( 'NONE', *, *, #14914, .F. ) ;
#12004=EDGE_CURVE ( 'NONE', #25971, #16316, #44052, .T. ) ;
#12005=DIRECTION ( 'NONE',  ( 1.000000000000000000, -7.175085443855143705E-17, -4.952603889763953902E-17 ) ) ;
#12007=PLANE ( 'NONE',  #49629 ) ;
#12009=DIRECTION ( 'NONE',  ( -0.000000000000000000, -3.491481338843133355E-15, -1.000000000000000000 ) ) ;
#12011=AXIS2_PLACEMENT_3D ( 'NONE', #29289, #22183, #45080 ) ;
#12017=DIRECTION ( 'NONE',  ( -0.000000000000000000, -0.8229838658936516893, 0.5680647467311626952 ) ) ;
#12027=ORIENTED_EDGE ( 'NONE', *, *, #7006, .F. ) ;
#12028=DIRECTION ( 'NONE',  ( -1.000000000000000000, 0.000000000000000000, 0.000000000000000000 ) ) ;
#12030=ORIENTED_EDGE ( 'NONE', *, *, #38401, .T. ) ;
#12036=EDGE_LOOP ( 'NONE', ( #21587, #49756, #7404, #31423 ) ) ;
#12040=ORIENTED_EDGE ( 'NONE', *, *, #305, .F. ) ;
#12041=CARTESIAN_POINT ( 'NONE',  ( -305.0000000000000568, -77.52356969168074841, 38.55084767037245541 ) ) ;
#12042=LINE ( 'NONE', #29120, #10701 ) ;
#12045=EDGE_LOOP ( 'NONE', ( #47661, #3834, #4684, #3790 ) ) ;
#12048=PLANE ( 'NONE',  #32230 ) ;
#12058=EDGE_CURVE ( 'NONE', #36418, #7888, #11657, .T. ) ;
#12061=ADVANCED_FACE ( 'NONE', ( #32995 ), #10380, .F. ) ;
#12063=DIRECTION ( 'NONE',  ( -0.000000000000000000, -0.8854560256532062468, 0.4647231720437755564 ) ) ;
#12067=ORIENTED_EDGE ( 'NONE', *, *, #4506, .F. ) ;
#12068=CARTESIAN_POINT ( 'NONE',  ( -339.1964088526558498, -182.0095552316576573, -7.608018572112655420 ) ) ;
#12071=CARTESIAN_POINT ( 'NONE',  ( -330.4913330509368166, -183.0001959263613571, 7.728304129925096966 ) ) ;
#12074=VECTOR ( 'NONE', #4192, 1000.000000000000000 ) ;
#12080=ORIENTED_EDGE ( 'NONE', *, *, #48430, .T. ) ;
#12081=CARTESIAN_POINT ( 'NONE',  ( -336.3521761649654422, -100.1170788342122080, 54.23253582808833073 ) ) ;
#12082=CIRCLE ( 'NONE', #41478, 60.00000000000000000 ) ;
#12084=DIRECTION ( 'NONE',  ( -1.000000000000000000, -1.258058860540462198E-15, 1.036104688092336837E-14 ) ) ;
#12085=CARTESIAN_POINT ( 'NONE',  ( 0.000000000000000000, -172.0560480877259408, -33.51582005713793677 ) ) ;
#12087=DIRECTION ( 'NONE',  ( 0.000000000000000000, 0.7485107481710977506, -0.6631226582407989678 ) ) ;
#12090=VERTEX_POINT ( 'NONE', #45882 ) ;
#12091=CARTESIAN_POINT ( 'NONE',  ( -339.1964088526558498, -66.09477493971917283, -13.63415328425296202 ) ) ;
#12097=LINE ( 'NONE', #43137, #30490 ) ;
#12098=DIRECTION ( 'NONE',  ( -0.000000000000000000, 0.2393156642875685636, 0.9709418174260492362 ) ) ;
#12101=EDGE_CURVE ( 'NONE', #34375, #3787, #18285, .T. ) ;
#12104=ORIENTED_EDGE ( 'NONE', *, *, #27726, .T. ) ;
#12112=ORIENTED_EDGE ( 'NONE', *, *, #12497, .T. ) ;
#12115=CARTESIAN_POINT ( 'NONE',  ( -339.1964088526558498, -167.3305728129748786, -39.49849221029221269 ) ) ;
#12119=DIRECTION ( 'NONE',  ( 1.000000000000000000, -0.000000000000000000, -0.000000000000000000 ) ) ;
#12125=DIRECTION ( 'NONE',  ( -0.000000000000000000, 1.000000000000000000, -1.047444401652940007E-14 ) ) ;
#12127=CARTESIAN_POINT ( 'NONE',  ( -330.4913330509368166, -162.2499814621216672, -44.49369547121515467 ) ) ;
#12128=AXIS2_PLACEMENT_3D ( 'NONE', #43969, #23245, #28192 ) ;
#12131=DIRECTION ( 'NONE',  ( -0.000000000000000000, -0.1205366802553268363, -0.9927088740980534176 ) ) ;
#12135=DIRECTION ( 'NONE',  ( -0.000000000000000000, 0.2393156642875547968, -0.9709418174260527890 ) ) ;
#12136=EDGE_CURVE ( 'NONE', #6991, #49014, #37463, .T. ) ;
#12138=VERTEX_POINT ( 'NONE', #13551 ) ;
#12142=FACE_OUTER_BOUND ( 'NONE', #8554, .T. ) ;
#12143=AXIS2_PLACEMENT_3D ( 'NONE', #45423, #33584, #16797 ) ;
#12150=EDGE_LOOP ( 'NONE', ( #49990, #42981, #38915, #24838 ) ) ;
#12155=VECTOR ( 'NONE', #12297, 1000.000000000000000 ) ;
#12156=CARTESIAN_POINT ( 'NONE',  ( -305.0000000000000568, -167.3116148657362032, 40.99441916720376611 ) ) ;
#12161=EDGE_CURVE ( 'NONE', #43135, #16449, #1980, .T. ) ;
#12162=EDGE_CURVE ( 'NONE', #40574, #44930, #46146, .T. ) ;
#12163=EDGE_CURVE ( 'NONE', #3974, #34018, #26808, .T. ) ;
#12164=PLANE ( 'NONE',  #5638 ) ;
#12165=AXIS2_PLACEMENT_3D ( 'NONE', #24992, #40472, #45235 ) ;
#12175=EDGE_LOOP ( 'NONE', ( #28272, #14676, #14904, #41259 ) ) ;
#12177=DIRECTION ( 'NONE',  ( 0.000000000000000000, 7.725301879683381348E-14, 1.000000000000000000 ) ) ;
#12179=DIRECTION ( 'NONE',  ( 0.000000000000000000, -0.9350162426854181641, -0.3546048870425267951 ) ) ;
#12180=EDGE_CURVE ( 'NONE', #28004, #19813, #39277, .T. ) ;
#12181=ORIENTED_EDGE ( 'NONE', *, *, #37833, .F. ) ;
#12183=ORIENTED_EDGE ( 'NONE', *, *, #51100, .F. ) ;
#12184=CARTESIAN_POINT ( 'NONE',  ( -330.4913330509368166, -84.75001853787871653, -44.49369547121542467 ) ) ;
#12186=CIRCLE ( 'NONE', #21428, 60.00000000000000000 ) ;
#12188=DIRECTION ( 'NONE',  ( -0.000000000000000000, -0.5680647467311596976, -0.8229838658936536877 ) ) ;
#12189=ORIENTED_EDGE ( 'NONE', *, *, #45194, .T. ) ;
#12191=AXIS2_PLACEMENT_3D ( 'NONE', #4784, #7680, #33145 ) ;
#12192=EDGE_CURVE ( 'NONE', #2225, #20894, #18534, .T. ) ;
#12194=FACE_OUTER_BOUND ( 'NONE', #379, .T. ) ;
#12196=CARTESIAN_POINT ( 'NONE',  ( -339.1964088526558498, -64.50000000000000000, 0.4999999999999543698 ) ) ;
#12200=DIRECTION ( 'NONE',  ( -8.718379230999707126E-17, -0.8854560256532141294, -0.4647231720437604574 ) ) ;
#12205=PLANE ( 'NONE',  #10204 ) ;
#12207=VECTOR ( 'NONE', #39493, 1000.000000000000000 ) ;
#12208=ORIENTED_EDGE ( 'NONE', *, *, #41732, .T. ) ;
#12211=EDGE_CURVE ( 'NONE', #18701, #4655, #39522, .T. ) ;
#12218=CARTESIAN_POINT ( 'NONE',  ( -330.4913330509368166, -124.0000000000001990, -59.99791663049643375 ) ) ;
#12222=ORIENTED_EDGE ( 'NONE', *, *, #18952, .T. ) ;
#12226=CARTESIAN_POINT ( 'NONE',  ( -365.0000000000001137, -168.5000000000000284, 10.00000000000000711 ) ) ;
#12228=DIRECTION ( 'NONE',  ( 0.000000000000000000, 0.000000000000000000, -1.000000000000000000 ) ) ;
#12229=AXIS2_PLACEMENT_3D ( 'NONE', #33343, #17582, #1270 ) ;
#12230=FACE_BOUND ( 'NONE', #33332, .T. ) ;
#12231=PLANE ( 'NONE',  #15495 ) ;
#12239=VERTEX_POINT ( 'NONE', #27444 ) ;
#12243=AXIS2_PLACEMENT_3D ( 'NONE', #29272, #45325, #49779 ) ;
#12244=DIRECTION ( 'NONE',  ( -1.000000000000000000, -0.000000000000000000, 0.000000000000000000 ) ) ;
#12251=ORIENTED_EDGE ( 'NONE', *, *, #39812, .F. ) ;
#12256=DIRECTION ( 'NONE',  ( -0.000000000000000000, -0.5680647467311596976, -0.8229838658936536877 ) ) ;
#12265=CIRCLE ( 'NONE', #24011, 60.00000000000000000 ) ;
#12268=VECTOR ( 'NONE', #37140, 1000.000000000000114 ) ;
#12270=DIRECTION ( 'NONE',  ( 0.000000000000000000, 0.000000000000000000, 1.000000000000000000 ) ) ;
#12276=DIRECTION ( 'NONE',  ( -0.000000000000000000, -0.3546048870425267951, 0.9350162426854181641 ) ) ;
#12277=AXIS2_PLACEMENT_3D ( 'NONE', #16867, #27644, #27884 ) ;
#12281=CIRCLE ( 'NONE', #41656, 60.00000000000000000 ) ;
#12283=DIRECTION ( 'NONE',  ( 1.000000000000000000, -0.000000000000000000, 0.000000000000000000 ) ) ;
#12284=ORIENTED_EDGE ( 'NONE', *, *, #18279, .F. ) ;
#12286=VECTOR ( 'NONE', #28710, 1000.000000000000000 ) ;
#12288=ORIENTED_EDGE ( 'NONE', *, *, #27431, .F. ) ;
#12291=CARTESIAN_POINT ( 'NONE',  ( -336.3521761649654422, -164.5945333327934463, -42.41660376256285048 ) ) ;
#12292=ADVANCED_FACE ( 'NONE', ( #3529 ), #3284, .F. ) ;
#12293=DIRECTION ( 'NONE',  ( -0.000000000000000000, -0.3546048870425267951, 0.9350162426854181641 ) ) ;
#12294=CARTESIAN_POINT ( 'NONE',  ( -336.3521761649654422, -76.43926241122620979, -35.68215131113738181 ) ) ;
#12297=DIRECTION ( 'NONE',  ( 1.000000000000000000, -0.000000000000000000, -0.000000000000000000 ) ) ;
#12302=DIRECTION ( 'NONE',  ( 1.000000000000000000, 4.952603889763975472E-17, -7.175085443855130147E-17 ) ) ;
#12307=FACE_OUTER_BOUND ( 'NONE', #40753, .T. ) ;
#12308=ORIENTED_EDGE ( 'NONE', *, *, #44941, .T. ) ;
#12316=VECTOR ( 'NONE', #31109, 1000.000000000000000 ) ;
#12320=DIRECTION ( 'NONE',  ( -0.000000000000000000, -0.1205366802553130001, 0.9927088740980551940 ) ) ;
#12321=VECTOR ( 'NONE', #24519, 1000.000000000000000 ) ;
#12322=VECTOR ( 'NONE', #31584, 1000.000000000000000 ) ;
#12324=ORIENTED_EDGE ( 'NONE', *, *, #17980, .T. ) ;
#12326=CARTESIAN_POINT ( 'NONE',  ( -339.1964088526558498, -182.1300919119129560, -6.615309698014600670 ) ) ;
#12327=CARTESIAN_POINT ( 'NONE',  ( -336.3521761649654422, -64.31210272782786319, -9.838334030657643225 ) ) ;
#12328=CIRCLE ( 'NONE', #20746, 60.00000000000000000 ) ;
#12331=PLANE ( 'NONE',  #18961 ) ;
#12333=DIRECTION ( 'NONE',  ( -0.000000000000000000, -0.6631226582407989678, -0.7485107481710977506 ) ) ;
#12334=VERTEX_POINT ( 'NONE', #43733 ) ;
#12335=VERTEX_POINT ( 'NONE', #7737 ) ;
#12339=VECTOR ( 'NONE', #12333, 1000.000000000000000 ) ;
#12346=CARTESIAN_POINT ( 'NONE',  ( -336.3521761649654422, -94.63601285149479736, 51.48334306143172512 ) ) ;
#12349=EDGE_LOOP ( 'NONE', ( #40209, #13863, #33091, #26003 ) ) ;
#12351=AXIS2_PLACEMENT_3D ( 'NONE', #23174, #43406, #6879 ) ;
#12352=ORIENTED_EDGE ( 'NONE', *, *, #49362, .T. ) ;
#12354=AXIS2_PLACEMENT_3D ( 'NONE', #36163, #47998, #43542 ) ;
#12357=ADVANCED_FACE ( 'NONE', ( #10905 ), #21319, .F. ) ;
#12363=VERTEX_POINT ( 'NONE', #32160 ) ;
#12366=EDGE_LOOP ( 'NONE', ( #15127, #47463, #5486, #7015 ) ) ;
#12367=PLANE ( 'NONE',  #7109 ) ;
#12381=CARTESIAN_POINT ( 'NONE',  ( -339.1964088526558498, -84.08827740916061089, 45.24064679492014562 ) ) ;
#12382=CARTESIAN_POINT ( 'NONE',  ( -336.3521761649654422, -113.6616659693417546, 59.18789727217205154 ) ) ;
#12384=CARTESIAN_POINT ( 'NONE',  ( 0.000000000000000000, -167.6621341420952547, -39.12423683620669124 ) ) ;
#12385=ORIENTED_EDGE ( 'NONE', *, *, #40701, .T. ) ;
#12387=DIRECTION ( 'NONE',  ( -0.000000000000000000, -0.6631226582407989678, -0.7485107481710977506 ) ) ;
#12388=ORIENTED_EDGE ( 'NONE', *, *, #15985, .F. ) ;
#12389=DIRECTION ( 'NONE',  ( -1.000000000000000000, 0.000000000000000000, 0.000000000000000000 ) ) ;
#12401=DIRECTION ( 'NONE',  ( -1.000000000000000000, 0.000000000000000000, 0.000000000000000000 ) ) ;
#12409=ORIENTED_EDGE ( 'NONE', *, *, #22952, .T. ) ;
#12416=AXIS2_PLACEMENT_3D ( 'NONE', #33510, #41900, #5917 ) ;
#12422=EDGE_CURVE ( 'NONE', #14384, #22837, #13180, .T. ) ;
#12429=EDGE_CURVE ( 'NONE', #37940, #4967, #15896, .T. ) ;
#12433=PLANE ( 'NONE',  #43148 ) ;
#12434=EDGE_CURVE ( 'NONE', #23911, #48950, #49184, .T. ) ;
#12439=ORIENTED_EDGE ( 'NONE', *, *, #25497, .F. ) ;
#12441=PLANE ( 'NONE',  #44967 ) ;
#12442=CARTESIAN_POINT ( 'NONE',  ( -336.3521761649654422, -105.0395444947681369, -56.09938080879045685 ) ) ;
#12443=ORIENTED_EDGE ( 'NONE', *, *, #49129, .F. ) ;
#12448=DIRECTION ( 'NONE',  ( 1.000000000000000000, -0.000000000000000000, -0.000000000000000000 ) ) ;
#12452=ADVANCED_FACE ( 'NONE', ( #49698 ), #43990, .F. ) ;
#12456=ORIENTED_EDGE ( 'NONE', *, *, #16409, .T. ) ;
#12461=CARTESIAN_POINT ( 'NONE',  ( -332.3517673607765914, -68.38646289696045244, -23.71704087764493707 ) ) ;
#12463=DIRECTION ( 'NONE',  ( -0.000000000000000000, 0.2393156642875652051, 0.9709418174260502354 ) ) ;
#12468=CARTESIAN_POINT ( 'NONE',  ( -336.3521761649653854, -94.18160986457394301, 52.34913561719000086 ) ) ;
#12469=DIRECTION ( 'NONE',  ( 0.000000000000000000, -0.9927088740980553050, -0.1205366802553130001 ) ) ;
#12473=ORIENTED_EDGE ( 'NONE', *, *, #16284, .T. ) ;
#12477=ADVANCED_FACE ( 'NONE', ( #23764 ), #26803, .F. ) ;
#12488=LINE ( 'NONE', #36394, #25259 ) ;
#12490=ORIENTED_EDGE ( 'NONE', *, *, #35002, .F. ) ;
#12492=EDGE_CURVE ( 'NONE', #42007, #31317, #30487, .T. ) ;
#12495=LINE ( 'NONE', #13537, #15156 ) ;
#12497=EDGE_CURVE ( 'NONE', #33568, #27241, #2633, .T. ) ;
#12500=FACE_BOUND ( 'NONE', #12366, .T. ) ;
#12504=ADVANCED_FACE ( 'NONE', ( #50482 ), #46795, .F. ) ;
#12511=ORIENTED_EDGE ( 'NONE', *, *, #50094, .T. ) ;
#12515=CARTESIAN_POINT ( 'NONE',  ( -339.1964088526558498, -64.50000000000000000, 0.4999999999999543698 ) ) ;
#12516=EDGE_LOOP ( 'NONE', ( #23569, #7702, #7399, #32912 ) ) ;
#12520=VECTOR ( 'NONE', #30100, 1000.000000000000000 ) ;
#12524=DIRECTION ( 'NONE',  ( -0.000000000000000000, 0.9350162426854146114, -0.3546048870425363986 ) ) ;
#12530=CARTESIAN_POINT ( 'NONE',  ( -339.1964088526558498, -172.5932850007654054, 34.49419324804723175 ) ) ;
#12531=DIRECTION ( 'NONE',  ( 0.000000000000000000, -0.9709418174260535661, -0.2393156642875516327 ) ) ;
#12537=EDGE_LOOP ( 'NONE', ( #14146, #9395, #37843, #27791, #46630 ) ) ;
#12540=EDGE_CURVE ( 'NONE', #32868, #41179, #38378, .T. ) ;
#12544=ADVANCED_FACE ( 'NONE', ( #14729 ), #18157, .F. ) ;
#12545=EDGE_CURVE ( 'NONE', #23080, #20926, #26035, .T. ) ;
#12546=CARTESIAN_POINT ( 'NONE',  ( -332.3517673607765914, -154.8494888031386836, 50.05135858667791382 ) ) ;
#12548=CARTESIAN_POINT ( 'NONE',  ( -336.3521761649654422, -107.7955183043589500, 56.89493493766750731 ) ) ;
#12549=ORIENTED_EDGE ( 'NONE', *, *, #46337, .T. ) ;
#12550=LINE ( 'NONE', #730, #47059 ) ;
#12552=VECTOR ( 'NONE', #33764, 1000.000000000000114 ) ;
#12559=DIRECTION ( 'NONE',  ( 1.000000000000000000, -0.000000000000000000, 0.000000000000000000 ) ) ;
#12564=VERTEX_POINT ( 'NONE', #981 ) ;
#12565=LINE ( 'NONE', #13084, #19791 ) ;
#12566=DIRECTION ( 'NONE',  ( 0.000000000000000000, -9.251858538542971828E-16, -1.000000000000000000 ) ) ;
#12569=CARTESIAN_POINT ( 'NONE',  ( -339.1964088526558498, -144.3080463282014136, 56.27632902032101470 ) ) ;
#12571=LINE ( 'NONE', #20986, #2111 ) ;
#12576=CARTESIAN_POINT ( 'NONE',  ( -336.3521761649654422, -176.9651911376907094, -25.08789112700655721 ) ) ;
#12581=CARTESIAN_POINT ( 'NONE',  ( -330.4913330509368166, -84.75001853787871653, -44.49369547121542467 ) ) ;
#12582=DIRECTION ( 'NONE',  ( 0.000000000000000000, -0.4647231720437573488, 0.8854560256532157947 ) ) ;
#12587=LINE ( 'NONE', #4198, #15411 ) ;
#12591=CARTESIAN_POINT ( 'NONE',  ( -305.0000000000000568, -137.3729703655840524, -58.37414404713467064 ) ) ;
#12596=FACE_OUTER_BOUND ( 'NONE', #21113, .T. ) ;
#12600=ORIENTED_EDGE ( 'NONE', *, *, #43645, .T. ) ;
#12605=CARTESIAN_POINT ( 'NONE',  ( -330.4913330509368166, -71.02573290043841325, 26.97593913775512320 ) ) ;
#12607=CARTESIAN_POINT ( 'NONE',  ( 0.000000000000000000, -84.37576316379318087, -44.16213414209506283 ) ) ;
#12608=DIRECTION ( 'NONE',  ( -1.000000000000000000, -0.000000000000000000, 0.000000000000000000 ) ) ;
#12609=ORIENTED_EDGE ( 'NONE', *, *, #49547, .T. ) ;
#12612=ORIENTED_EDGE ( 'NONE', *, *, #49412, .F. ) ;
#12618=DIRECTION ( 'NONE',  ( 0.000000000000000000, -0.9927088740980526405, 0.1205366802553337890 ) ) ;
#12619=DIRECTION ( 'NONE',  ( 1.000000000000000000, -0.000000000000000000, -0.000000000000000000 ) ) ;
#12621=CARTESIAN_POINT ( 'NONE',  ( -336.3521761649653854, -158.9146170832377720, -48.43351006119259949 ) ) ;
#12622=ORIENTED_EDGE ( 'NONE', *, *, #37934, .F. ) ;
#12624=CARTESIAN_POINT ( 'NONE',  ( -330.4913330509368166, -143.9541802141664562, 55.34326076196094135 ) ) ;
#12627=EDGE_CURVE ( 'NONE', #37301, #25289, #9921, .T. ) ;
#12629=CARTESIAN_POINT ( 'NONE',  ( -336.3521761649654422, -123.5000000000000284, 0.000000000000000000 ) ) ;
#12632=CARTESIAN_POINT ( 'NONE',  ( -332.3517673607765914, -141.9604555052315220, 56.09938080879057765 ) ) ;
#12635=AXIS2_PLACEMENT_3D ( 'NONE', #15413, #18566, #26709 ) ;
#12636=ORIENTED_EDGE ( 'NONE', *, *, #11391, .F. ) ;
#12640=ORIENTED_EDGE ( 'NONE', *, *, #7353, .T. ) ;
#12641=DIRECTION ( 'NONE',  ( 0.000000000000000000, 0.000000000000000000, -1.000000000000000000 ) ) ;
#12646=DIRECTION ( 'NONE',  ( -0.000000000000000000, -0.1205366802553164696, 0.9927088740980548609 ) ) ;
#12649=DIRECTION ( 'NONE',  ( -1.000000000000000000, 0.000000000000000000, 0.000000000000000000 ) ) ;
#12650=DIRECTION ( 'NONE',  ( 0.000000000000000000, -4.394632805807911569E-15, -1.000000000000000000 ) ) ;
#12652=EDGE_CURVE ( 'NONE', #31272, #40382, #1235, .T. ) ;
#12654=CIRCLE ( 'NONE', #47076, 60.00000000000000000 ) ;
#12655=LINE ( 'NONE', #45001, #8666 ) ;
#12657=DIRECTION ( 'NONE',  ( -0.000000000000000000, 0.9709418174260553425, 0.2393156642875449158 ) ) ;
#12658=DIRECTION ( 'NONE',  ( 0.000000000000000000, 0.4647231720437695057, 0.8854560256532093554 ) ) ;
#12660=VERTEX_POINT ( 'NONE', #49605 ) ;
#12661=VERTEX_POINT ( 'NONE', #45936 ) ;
#12665=VERTEX_POINT ( 'NONE', #49863 ) ;
#12667=VERTEX_POINT ( 'NONE', #49354 ) ;
#12678=ORIENTED_EDGE ( 'NONE', *, *, #155, .T. ) ;
#12679=LINE ( 'NONE', #28451, #39597 ) ;
#12686=LINE ( 'NONE', #13228, #3665 ) ;
#12689=EDGE_LOOP ( 'NONE', ( #329, #41353, #46147, #4498 ) ) ;
#12691=FACE_OUTER_BOUND ( 'NONE', #18022, .T. ) ;
#12698=LINE ( 'NONE', #24288, #46882 ) ;
#12701=ORIENTED_EDGE ( 'NONE', *, *, #6275, .F. ) ;
#12705=PLANE ( 'NONE',  #13597 ) ;
#12706=VERTEX_POINT ( 'NONE', #9398 ) ;
#12716=ORIENTED_EDGE ( 'NONE', *, *, #13516, .T. ) ;
#12720=ORIENTED_EDGE ( 'NONE', *, *, #8357, .F. ) ;
#12721=VECTOR ( 'NONE', #47627, 1000.000000000000227 ) ;
#12724=DIRECTION ( 'NONE',  ( 0.000000000000000000, 0.000000000000000000, -1.000000000000000000 ) ) ;
#12729=FACE_OUTER_BOUND ( 'NONE', #51482, .T. ) ;
#12731=DIRECTION ( 'NONE',  ( -1.000000000000000000, 0.000000000000000000, 0.000000000000000000 ) ) ;
#12733=CARTESIAN_POINT ( 'NONE',  ( -339.1964088526558498, -162.2499814621209850, 44.49369547121574442 ) ) ;
#12739=CARTESIAN_POINT ( 'NONE',  ( -330.4913330509368166, -74.65991953890876687, -33.10432812419148263 ) ) ;
#12741=VECTOR ( 'NONE', #42755, 1000.000000000000114 ) ;
#12743=FACE_BOUND ( 'NONE', #43955, .T. ) ;
#12744=FACE_OUTER_BOUND ( 'NONE', #47664, .T. ) ;
#12749=ORIENTED_EDGE ( 'NONE', *, *, #34509, .T. ) ;
#12755=DIRECTION ( 'NONE',  ( -1.000000000000000000, 0.000000000000000000, -0.000000000000000000 ) ) ;
#12757=EDGE_CURVE ( 'NONE', #28909, #20222, #22778, .T. ) ;
#12762=EDGE_CURVE ( 'NONE', #8786, #51399, #39043, .T. ) ;
#12769=FACE_OUTER_BOUND ( 'NONE', #31155, .T. ) ;
#12779=CARTESIAN_POINT ( 'NONE',  ( -330.4913330509368166, -71.02573290043841325, 26.97593913775512320 ) ) ;
#12787=DIRECTION ( 'NONE',  ( 0.000000000000000000, -0.1205366802553268640, -0.9927088740980535286 ) ) ;
#12791=ORIENTED_EDGE ( 'NONE', *, *, #38812, .T. ) ;
#12792=ADVANCED_FACE ( 'NONE', ( #50904 ), #14909, .F. ) ;
#12793=PLANE ( 'NONE',  #14236 ) ;
#12794=DIRECTION ( 'NONE',  ( 0.000000000000000000, -1.119474883163699554E-13, -1.000000000000000000 ) ) ;
#12798=DIRECTION ( 'NONE',  ( 0.000000000000000000, 0.000000000000000000, -1.000000000000000000 ) ) ;
#12801=AXIS2_PLACEMENT_3D ( 'NONE', #25279, #33437, #1360 ) ;
#12802=ORIENTED_EDGE ( 'NONE', *, *, #240, .T. ) ;
#12803=LINE ( 'NONE', #8867, #24219 ) ;
#12819=ORIENTED_EDGE ( 'NONE', *, *, #21208, .T. ) ;
#12820=DIRECTION ( 'NONE',  ( -0.000000000000000000, 0.5680647467311656929, 0.8229838658936495799 ) ) ;
#12831=CARTESIAN_POINT ( 'NONE',  ( -336.3521761649654422, -123.5000000000000284, 0.000000000000000000 ) ) ;
#12832=FACE_OUTER_BOUND ( 'NONE', #34144, .T. ) ;
#12833=VERTEX_POINT ( 'NONE', #35114 ) ;
#12837=DIRECTION ( 'NONE',  ( -0.000000000000000000, 0.000000000000000000, -1.000000000000000000 ) ) ;
#12838=LINE ( 'NONE', #29127, #38941 ) ;
#12840=ORIENTED_EDGE ( 'NONE', *, *, #22405, .F. ) ;
#12844=DIRECTION ( 'NONE',  ( 1.000000000000000000, 0.000000000000000000, -0.000000000000000000 ) ) ;
#12845=CARTESIAN_POINT ( 'NONE',  ( -339.1964088526558498, -108.8949048983213004, -57.16590939599337418 ) ) ;
#12847=AXIS2_PLACEMENT_3D ( 'NONE', #19287, #42672, #6682 ) ;
#12848=LINE ( 'NONE', #43870, #24901 ) ;
#12849=ORIENTED_EDGE ( 'NONE', *, *, #22279, .F. ) ;
#12850=VERTEX_POINT ( 'NONE', #30143 ) ;
#12856=EDGE_LOOP ( 'NONE', ( #27139, #7475, #25058, #9653 ) ) ;
#12857=VERTEX_POINT ( 'NONE', #44313 ) ;
#12859=ORIENTED_EDGE ( 'NONE', *, *, #39344, .F. ) ;
#12860=VECTOR ( 'NONE', #18047, 1000.000000000000000 ) ;
#12861=EDGE_CURVE ( 'NONE', #42654, #47556, #27741, .T. ) ;
#12862=LINE ( 'NONE', #28882, #41039 ) ;
#12868=DIRECTION ( 'NONE',  ( 0.000000000000000000, 0.8854560256532157947, 0.4647231720437573488 ) ) ;
#12869=VECTOR ( 'NONE', #48026, 1000.000000000000000 ) ;
#12876=LINE ( 'NONE', #33631, #30960 ) ;
#12880=LINE ( 'NONE', #9214, #36976 ) ;
#12883=ORIENTED_EDGE ( 'NONE', *, *, #7791, .T. ) ;
#12885=ORIENTED_EDGE ( 'NONE', *, *, #30442, .F. ) ;
#12890=ADVANCED_FACE ( 'NONE', ( #27217 ), #28000, .T. ) ;
#12902=FACE_OUTER_BOUND ( 'NONE', #17523, .T. ) ;
#12905=VERTEX_POINT ( 'NONE', #51425 ) ;
#12907=FACE_OUTER_BOUND ( 'NONE', #42358, .T. ) ;
#12914=CARTESIAN_POINT ( 'NONE',  ( -339.1964088526558498, -116.7644047441726656, 59.62073260661660612 ) ) ;
#12917=EDGE_CURVE ( 'NONE', #36663, #24196, #36148, .T. ) ;
#12921=DIRECTION ( 'NONE',  ( 1.000000000000000000, 0.000000000000000000, 0.000000000000000000 ) ) ;
#12926=ORIENTED_EDGE ( 'NONE', *, *, #35337, .F. ) ;
#12928=VERTEX_POINT ( 'NONE', #12226 ) ;
#12929=FACE_OUTER_BOUND ( 'NONE', #46649, .T. ) ;
#12932=ORIENTED_EDGE ( 'NONE', *, *, #18250, .T. ) ;
#12939=AXIS2_PLACEMENT_3D ( 'NONE', #36089, #48711, #8237 ) ;
#12945=DIRECTION ( 'NONE',  ( -1.000000000000000000, 0.000000000000000000, 0.000000000000000000 ) ) ;
#12952=LINE ( 'NONE', #28976, #39905 ) ;
#12954=ORIENTED_EDGE ( 'NONE', *, *, #19492, .T. ) ;
#12960=CARTESIAN_POINT ( 'NONE',  ( -336.3521761649654422, -135.0638248728647852, 57.91551518289418254 ) ) ;
#12965=CARTESIAN_POINT ( 'NONE',  ( -339.1964088526558498, -182.0095552316576573, -7.608018572112655420 ) ) ;
#12971=CARTESIAN_POINT ( 'NONE',  ( -305.0000000000000568, -113.6616659693417546, 59.18789727217205154 ) ) ;
#12972=PLANE ( 'NONE',  #5619 ) ;
#12976=ORIENTED_EDGE ( 'NONE', *, *, #20373, .T. ) ;
#12984=DIRECTION ( 'NONE',  ( 1.000000000000000000, 0.000000000000000000, 0.000000000000000000 ) ) ;
#12986=DIRECTION ( 'NONE',  ( 0.000000000000000000, 0.9927088740980539727, -0.1205366802553233252 ) ) ;
#12989=DIRECTION ( 'NONE',  ( -0.000000000000000000, 0.8229838658936634577, 0.5680647467311457088 ) ) ;
#12990=CIRCLE ( 'NONE', #44896, 60.00000000000000000 ) ;
#12992=CARTESIAN_POINT ( 'NONE',  ( -330.4913330509368166, -182.1300919119128423, 6.615309698015510165 ) ) ;
#12993=CARTESIAN_POINT ( 'NONE',  ( -339.1964088526558498, -78.25935320507889514, 39.41172259083828777 ) ) ;
#12994=AXIS2_PLACEMENT_3D ( 'NONE', #28755, #48508, #41120 ) ;
#12996=LINE ( 'NONE', #16716, #29445 ) ;
#13002=EDGE_CURVE ( 'NONE', #16187, #25920, #35366, .T. ) ;
#13013=DIRECTION ( 'NONE',  ( -8.718379230999708359E-17, -0.2393156642875652051, -0.9709418174260502354 ) ) ;
#13024=DIRECTION ( 'NONE',  ( -1.000000000000000000, -0.000000000000000000, 0.000000000000000000 ) ) ;
#13025=CARTESIAN_POINT ( 'NONE',  ( -330.4913330509368166, -143.9541802141672235, -55.34326076196065003 ) ) ;
#13026=EDGE_LOOP ( 'NONE', ( #31259, #28413, #34326, #49616 ) ) ;
#13029=AXIS2_PLACEMENT_3D ( 'NONE', #9902, #37744, #13046 ) ;
#13031=CARTESIAN_POINT ( 'NONE',  ( -336.3521761649654422, -65.58448481710581746, 11.56382487286456140 ) ) ;
#13033=PLANE ( 'NONE',  #39580 ) ;
#13036=CARTESIAN_POINT ( 'NONE',  ( -330.4913330509368166, -116.8846903019851311, -58.63009191191288494 ) ) ;
#13037=DIRECTION ( 'NONE',  ( -1.000000000000000000, 0.000000000000000000, 0.000000000000000000 ) ) ;
#13038=ORIENTED_EDGE ( 'NONE', *, *, #17516, .F. ) ;
#13039=AXIS2_PLACEMENT_3D ( 'NONE', #29430, #22325, #45483 ) ;
#13045=ORIENTED_EDGE ( 'NONE', *, *, #11224, .T. ) ;
#13046=DIRECTION ( 'NONE',  ( 0.000000000000000000, -2.567390744445674500E-14, 1.000000000000000000 ) ) ;
#13047=ORIENTED_EDGE ( 'NONE', *, *, #7681, .T. ) ;
#13049=ORIENTED_EDGE ( 'NONE', *, *, #22700, .T. ) ;
#13050=CARTESIAN_POINT ( 'NONE',  ( -305.0000000000000568, -67.57827586672165410, -21.74306257088711547 ) ) ;
#13053=AXIS2_PLACEMENT_3D ( 'NONE', #39217, #30817, #14280 ) ;
#13058=AXIS2_PLACEMENT_3D ( 'NONE', #50547, #27123, #47118 ) ;
#13062=LINE ( 'NONE', #41177, #862 ) ;
#13064=VERTEX_POINT ( 'NONE', #32728 ) ;
#13065=EDGE_CURVE ( 'NONE', #46710, #36128, #45612, .T. ) ;
#13072=ADVANCED_FACE ( 'NONE', ( #16724 ), #29029, .F. ) ;
#13074=CARTESIAN_POINT ( 'NONE',  ( -339.1964088526558498, -123.5000000000000284, 0.000000000000000000 ) ) ;
#13075=CARTESIAN_POINT ( 'NONE',  ( -330.4913330509368166, -68.15673923803900891, 20.45418021416622878 ) ) ;
#13076=ORIENTED_EDGE ( 'NONE', *, *, #38803, .T. ) ;
#13077=EDGE_CURVE ( 'NONE', #8870, #22194, #12495, .T. ) ;
#13084=CARTESIAN_POINT ( 'NONE',  ( -336.3521761649654422, -127.9985676343858501, 58.88711093124869222 ) ) ;
#13085=DIRECTION ( 'NONE',  ( -0.000000000000000000, -0.9709418174260511236, 0.2393156642875615969 ) ) ;
#13086=ORIENTED_EDGE ( 'NONE', *, *, #37473, .F. ) ;
#13087=ORIENTED_EDGE ( 'NONE', *, *, #22931, .T. ) ;
#13092=VERTEX_POINT ( 'NONE', #16971 ) ;
#13098=ORIENTED_EDGE ( 'NONE', *, *, #788, .F. ) ;
#13100=LINE ( 'NONE', #45187, #27871 ) ;
#13102=FACE_OUTER_BOUND ( 'NONE', #25452, .T. ) ;
#13110=CARTESIAN_POINT ( 'NONE',  ( -330.4913330509368166, -83.33976666098958219, 44.57752413667940772 ) ) ;
#13111=CARTESIAN_POINT ( 'NONE',  ( 0.000000000000000000, -68.33404168156025094, 20.92168833550889673 ) ) ;
#13112=FACE_OUTER_BOUND ( 'NONE', #16011, .T. ) ;
#13113=ADVANCED_FACE ( 'NONE', ( #33243 ), #36936, .F. ) ;
#13115=DIRECTION ( 'NONE',  ( 0.000000000000000000, 0.2393156642875482742, -0.9709418174260544543 ) ) ;
#13118=VECTOR ( 'NONE', #39704, 1000.000000000000000 ) ;
#13120=AXIS2_PLACEMENT_3D ( 'NONE', #47309, #43359, #11023 ) ;
#13122=CARTESIAN_POINT ( 'NONE',  ( -336.3521761649653854, -183.4777928329299357, 1.632288850093980725 ) ) ;
#13124=DIRECTION ( 'NONE',  ( -0.000000000000000000, 0.1205366802553303196, 0.9927088740980530845 ) ) ;
#13126=VERTEX_POINT ( 'NONE', #17503 ) ;
#13131=DIRECTION ( 'NONE',  ( 1.000000000000000000, -0.000000000000000000, -0.000000000000000000 ) ) ;
#13133=VERTEX_POINT ( 'NONE', #49810 ) ;
#13140=DIRECTION ( 'NONE',  ( -1.000000000000000000, 0.000000000000000000, 0.000000000000000000 ) ) ;
#13141=ORIENTED_EDGE ( 'NONE', *, *, #7360, .F. ) ;
#13145=VERTEX_POINT ( 'NONE', #5926 ) ;
#13147=EDGE_CURVE ( 'NONE', #3885, #21496, #42157, .T. ) ;
#13151=DIRECTION ( 'NONE',  ( 0.000000000000000000, 6.476300976980080240E-14, -1.000000000000000000 ) ) ;
#13152=DIRECTION ( 'NONE',  ( 1.000000000000000000, -0.000000000000000000, 0.000000000000000000 ) ) ;
#13156=AXIS2_PLACEMENT_3D ( 'NONE', #51677, #15676, #4610 ) ;
#13157=ADVANCED_FACE ( 'NONE', ( #34530 ), #38488, .F. ) ;
#13158=VECTOR ( 'NONE', #26281, 1000.000000000000000 ) ;
#13164=DIRECTION ( 'NONE',  ( 0.000000000000000000, -0.9709418174260492362, 0.2393156642875685636 ) ) ;
#13168=DIRECTION ( 'NONE',  ( 0.000000000000000000, 0.3546048870425363986, 0.9350162426854146114 ) ) ;
#13170=DIRECTION ( 'NONE',  ( 1.000000000000000000, -0.000000000000000000, -0.000000000000000000 ) ) ;
#13173=AXIS2_PLACEMENT_3D ( 'NONE', #10065, #50277, #1662 ) ;
#13174=DIRECTION ( 'NONE',  ( -0.000000000000000000, -0.9350162426854169428, -0.3546048870425300148 ) ) ;
#13178=CARTESIAN_POINT ( 'NONE',  ( -339.1964088526558498, -182.5000000000000568, 0.5000000000000457412 ) ) ;
#13180=LINE ( 'NONE', #13433, #7501 ) ;
#13181=CARTESIAN_POINT ( 'NONE',  ( -365.0000000000001137, -168.5000000000000284, 10.00000000000000711 ) ) ;
#13183=DIRECTION ( 'NONE',  ( -1.000000000000000000, 0.000000000000000000, -0.000000000000000000 ) ) ;
#13191=AXIS2_PLACEMENT_3D ( 'NONE', #51863, #31343, #40254 ) ;
#13192=LINE ( 'NONE', #306, #10942 ) ;
#13197=LINE ( 'NONE', #29219, #36208 ) ;
#13199=DIRECTION ( 'NONE',  ( -1.000000000000000000, 0.000000000000000000, 0.000000000000000000 ) ) ;
#13210=ORIENTED_EDGE ( 'NONE', *, *, #26302, .F. ) ;
#13216=LINE ( 'NONE', #4547, #1714 ) ;
#13218=DIRECTION ( 'NONE',  ( 0.000000000000000000, 0.000000000000000000, -1.000000000000000000 ) ) ;
#13223=EDGE_LOOP ( 'NONE', ( #39125, #24687, #20891, #24250 ) ) ;
#13224=DIRECTION ( 'NONE',  ( -1.000000000000000000, 0.000000000000000000, 0.000000000000000000 ) ) ;
#13228=CARTESIAN_POINT ( 'NONE',  ( -339.1964088526558498, -75.22798428563991990, -33.92731199008514409 ) ) ;
#13231=EDGE_LOOP ( 'NONE', ( #18728, #30871, #36443, #30692 ) ) ;
#13235=DIRECTION ( 'NONE',  ( 0.000000000000000000, -0.7485107481710999711, 0.6631226582407964143 ) ) ;
#13238=FACE_OUTER_BOUND ( 'NONE', #33496, .T. ) ;
#13241=ORIENTED_EDGE ( 'NONE', *, *, #1457, .T. ) ;
#13242=FACE_BOUND ( 'NONE', #47033, .T. ) ;
#13244=LINE ( 'NONE', #12960, #6358 ) ;
#13250=VERTEX_POINT ( 'NONE', #11386 ) ;
#13251=CARTESIAN_POINT ( 'NONE',  ( 0.000000000000000000, -137.6196241929653752, 57.28556722813723212 ) ) ;
#13252=LINE ( 'NONE', #12971, #10442 ) ;
#13254=CARTESIAN_POINT ( 'NONE',  ( -336.3521761649654422, -113.7752393642576720, 58.25253621232167944 ) ) ;
#13255=ORIENTED_EDGE ( 'NONE', *, *, #24896, .T. ) ;
#13260=VECTOR ( 'NONE', #4371, 1000.000000000000000 ) ;
#13261=CARTESIAN_POINT ( 'NONE',  ( -305.0000000000000568, -182.3303666475049170, -11.78931550685388707 ) ) ;
#13266=DIRECTION ( 'NONE',  ( 1.000000000000000000, 0.000000000000000000, -0.000000000000000000 ) ) ;
#13268=PLANE ( 'NONE',  #33817 ) ;
#13270=AXIS2_PLACEMENT_3D ( 'NONE', #38600, #2604, #14694 ) ;
#13273=VERTEX_POINT ( 'NONE', #32140 ) ;
#13275=CARTESIAN_POINT ( 'NONE',  ( -305.0000000000000568, -144.3080463282022663, -56.27632902032068785 ) ) ;
#13276=CARTESIAN_POINT ( 'NONE',  ( -332.3517673607765914, -65.58448481710581746, 11.56382487286456140 ) ) ;
#13278=EDGE_LOOP ( 'NONE', ( #26018, #18347, #11986, #14401 ) ) ;
#13280=ORIENTED_EDGE ( 'NONE', *, *, #50656, .T. ) ;
#13283=DIRECTION ( 'NONE',  ( -8.718379230999708359E-17, -0.7485107481710934207, 0.6631226582408039638 ) ) ;
#13289=CARTESIAN_POINT ( 'NONE',  ( -339.1964088526558498, -180.6659093959932250, 14.60509510167942437 ) ) ;
#13290=VERTEX_POINT ( 'NONE', #23740 ) ;
#13296=AXIS2_PLACEMENT_3D ( 'NONE', #18702, #30518, #46062 ) ;
#13299=DIRECTION ( 'NONE',  ( 1.000000000000000000, -0.000000000000000000, -0.000000000000000000 ) ) ;
#13300=ORIENTED_EDGE ( 'NONE', *, *, #42632, .F. ) ;
#13301=CARTESIAN_POINT ( 'NONE',  ( -332.3517673607765914, -123.5000000000000284, 0.000000000000000000 ) ) ;
#13303=EDGE_LOOP ( 'NONE', ( #4619, #17060, #35404, #45950 ) ) ;
#13305=CARTESIAN_POINT ( 'NONE',  ( -332.3517673607765914, -113.7752393642576720, 58.25253621232167944 ) ) ;
#13312=CARTESIAN_POINT ( 'NONE',  ( -339.1964088526558498, -67.22367097967925531, -20.80804632820203182 ) ) ;
#13313=FACE_OUTER_BOUND ( 'NONE', #2906, .T. ) ;
#13320=CARTESIAN_POINT ( 'NONE',  ( -339.1964088526558498, -66.09477493971894546, 13.63415328425207917 ) ) ;
#13324=DIRECTION ( 'NONE',  ( 0.000000000000000000, -0.8854560256532126861, -0.4647231720437631775 ) ) ;
#13334=LINE ( 'NONE', #25667, #7797 ) ;
#13337=DIRECTION ( 'NONE',  ( -1.000000000000000000, 0.000000000000000000, 0.000000000000000000 ) ) ;
#13339=VERTEX_POINT ( 'NONE', #3268 ) ;
#13345=ADVANCED_FACE ( 'NONE', ( #7717 ), #19301, .F. ) ;
#13348=CARTESIAN_POINT ( 'NONE',  ( -330.4913330509368166, -96.52406086224361559, 52.47426709956096147 ) ) ;
#13355=DIRECTION ( 'NONE',  ( 0.000000000000000000, 0.9927088740980527515, -0.1205366802553337890 ) ) ;
#13356=VERTEX_POINT ( 'NONE', #15105 ) ;
#13358=ORIENTED_EDGE ( 'NONE', *, *, #43214, .F. ) ;
#13360=VERTEX_POINT ( 'NONE', #19793 ) ;
#13365=ORIENTED_EDGE ( 'NONE', *, *, #17072, .F. ) ;
#13366=EDGE_LOOP ( 'NONE', ( #20291, #22411, #25181, #48559 ) ) ;
#13369=VECTOR ( 'NONE', #21276, 1000.000000000000000 ) ;
#13370=DIRECTION ( 'NONE',  ( 0.000000000000000000, -0.8229838658936596829, -0.5680647467311510379 ) ) ;
#13373=LINE ( 'NONE', #6262, #30956 ) ;
#13376=EDGE_CURVE ( 'NONE', #19012, #11792, #3764, .T. ) ;
#13382=DIRECTION ( 'NONE',  ( 0.000000000000000000, 0.000000000000000000, 1.000000000000000000 ) ) ;
#13383=VERTEX_POINT ( 'NONE', #43966 ) ;
#13387=VERTEX_POINT ( 'NONE', #43468 ) ;
#13391=EDGE_CURVE ( 'NONE', #33271, #22773, #13216, .T. ) ;
#13398=ADVANCED_FACE ( 'NONE', ( #28448 ), #8738, .F. ) ;
#13399=ORIENTED_EDGE ( 'NONE', *, *, #44171, .T. ) ;
#13403=ORIENTED_EDGE ( 'NONE', *, *, #3657, .F. ) ;
#13407=DIRECTION ( 'NONE',  ( -1.000000000000000000, -0.000000000000000000, -0.000000000000000000 ) ) ;
#13413=DIRECTION ( 'NONE',  ( -0.000000000000000000, 0.3546048870425463906, 0.9350162426854107256 ) ) ;
#13419=DIRECTION ( 'NONE',  ( -1.000000000000000000, -0.000000000000000000, 0.000000000000000000 ) ) ;
#13433=CARTESIAN_POINT ( 'NONE',  ( -305.0000000000000568, -130.2355952558269223, -59.62073260661665586 ) ) ;
#13434=DIRECTION ( 'NONE',  ( -0.9993908270190956511, 0.000000000000000000, 0.03489949670250096919 ) ) ;
#13435=EDGE_CURVE ( 'NONE', #44829, #21855, #25210, .T. ) ;
#13438=EDGE_CURVE ( 'NONE', #22275, #16038, #36339, .T. ) ;
#13442=CARTESIAN_POINT ( 'NONE',  ( -339.1964088526558498, -168.7406467949202806, 39.41172259083927543 ) ) ;
#13443=ORIENTED_EDGE ( 'NONE', *, *, #2155, .F. ) ;
#13445=DIRECTION ( 'NONE',  ( -1.000000000000000000, 0.000000000000000000, 0.000000000000000000 ) ) ;
#13447=DIRECTION ( 'NONE',  ( 0.000000000000000000, 0.8229838658936516893, -0.5680647467311626952 ) ) ;
#13450=EDGE_CURVE ( 'NONE', #45109, #31967, #41314, .T. ) ;
#13452=CARTESIAN_POINT ( 'NONE',  ( -339.1964088526558498, -144.8891964568526305, -54.98865587491811624 ) ) ;
#13455=CARTESIAN_POINT ( 'NONE',  ( -336.3521761649654422, -177.7994952405510389, -25.52576769896207054 ) ) ;
#13462=AXIS2_PLACEMENT_3D ( 'NONE', #29485, #36870, #32662 ) ;
#13476=ORIENTED_EDGE ( 'NONE', *, *, #13522, .T. ) ;
#13477=VECTOR ( 'NONE', #46959, 1000.000000000000000 ) ;
#13480=CARTESIAN_POINT ( 'NONE',  ( -305.0000000000000568, -170.1129345408508868, -37.77875505479702412 ) ) ;
#13484=CARTESIAN_POINT ( 'NONE',  ( -336.3521761649654422, -133.2247606357419443, -58.25253621232173629 ) ) ;
#13487=LINE ( 'NONE', #29505, #448 ) ;
#13488=CARTESIAN_POINT ( 'NONE',  ( -336.3521761649654422, -149.4733471526596134, 53.00046796564699036 ) ) ;
#13489=VERTEX_POINT ( 'NONE', #5077 ) ;
#13490=CARTESIAN_POINT ( 'NONE',  ( -332.3517673607765914, -155.6724726690323450, 49.48329383994676078 ) ) ;
#13493=ADVANCED_FACE ( 'NONE', ( #18709 ), #42619, .F. ) ;
#13495=DIRECTION ( 'NONE',  ( 0.000000000000000000, 0.000000000000000000, 1.000000000000000000 ) ) ;
#13496=CARTESIAN_POINT ( 'NONE',  ( -336.3521761649654422, -182.5000000000000568, 1.632288850093980725 ) ) ;
#13499=AXIS2_PLACEMENT_3D ( 'NONE', #32574, #25215, #5251 ) ;
#13504=DIRECTION ( 'NONE',  ( -1.000000000000000000, -0.000000000000000000, 0.000000000000000000 ) ) ;
#13514=VERTEX_POINT ( 'NONE', #6119 ) ;
#13516=EDGE_CURVE ( 'NONE', #3140, #32119, #35282, .T. ) ;
#13517=DIRECTION ( 'NONE',  ( 0.000000000000000000, -0.7485107481710934207, 0.6631226582408039638 ) ) ;
#13520=ORIENTED_EDGE ( 'NONE', *, *, #10646, .T. ) ;
#13522=EDGE_CURVE ( 'NONE', #10774, #6991, #22395, .T. ) ;
#13526=VERTEX_POINT ( 'NONE', #34222 ) ;
#13532=ORIENTED_EDGE ( 'NONE', *, *, #18375, .T. ) ;
#13533=ORIENTED_EDGE ( 'NONE', *, *, #7502, .F. ) ;
#13537=CARTESIAN_POINT ( 'NONE',  ( -305.0000000000000568, -67.22367097967925531, -20.80804632820203182 ) ) ;
#13539=PLANE ( 'NONE',  #46558 ) ;
#13543=DIRECTION ( 'NONE',  ( 0.000000000000000000, 0.9709418174260502354, -0.2393156642875652051 ) ) ;
#13546=AXIS2_PLACEMENT_3D ( 'NONE', #14312, #31101, #6691 ) ;
#13551=CARTESIAN_POINT ( 'NONE',  ( -330.4913330509368166, -156.6043281241916816, -48.84008046109114076 ) ) ;
#13553=ORIENTED_EDGE ( 'NONE', *, *, #22747, .F. ) ;
#13556=APPLICATION_CONTEXT ( 'automotive_design' ) ;
#13558=DIRECTION ( 'NONE',  ( -1.000000000000000000, -0.000000000000000000, -0.000000000000000000 ) ) ;
#13561=VECTOR ( 'NONE', #16163, 999.9999999999998863 ) ;
#13562=DIRECTION ( 'NONE',  ( -0.000000000000000000, 0.9927088740980556381, 0.1205366802553095307 ) ) ;
#13563=LINE ( 'NONE', #21191, #21334 ) ;
#13564=PLANE ( 'NONE',  #27899 ) ;
#13565=VECTOR ( 'NONE', #2260, 1000.000000000000000 ) ;
#13566=CARTESIAN_POINT ( 'NONE',  ( -339.1964088526558498, -123.5000000000000284, 0.000000000000000000 ) ) ;
#13568=DIRECTION ( 'NONE',  ( 1.000000000000000000, 1.050884489711663158E-17, 8.654812430365575371E-17 ) ) ;
#13573=ORIENTED_EDGE ( 'NONE', *, *, #14342, .T. ) ;
#13578=EDGE_CURVE ( 'NONE', #1973, #31995, #30524, .T. ) ;
#13582=CARTESIAN_POINT ( 'NONE',  ( -330.4913330509368166, -167.3305728129748786, -39.49849221029221269 ) ) ;
#13593=DIRECTION ( 'NONE',  ( 0.000000000000000000, 1.410908427127803051E-14, -1.000000000000000000 ) ) ;
#13597=AXIS2_PLACEMENT_3D ( 'NONE', #4855, #28991, #44522 ) ;
#13601=DIRECTION ( 'NONE',  ( -1.000000000000000000, 0.000000000000000000, -0.000000000000000000 ) ) ;
#13603=LINE ( 'NONE', #30152, #32345 ) ;
#13607=DIRECTION ( 'NONE',  ( -1.000000000000000000, 0.000000000000000000, 0.000000000000000000 ) ) ;
#13608=CARTESIAN_POINT ( 'NONE',  ( -339.1964088526558498, -156.6043281241916816, -48.84008046109114076 ) ) ;
#13613=EDGE_LOOP ( 'NONE', ( #16565, #29025, #14364, #19222 ) ) ;
#13615=CARTESIAN_POINT ( 'NONE',  ( -332.3517673607765914, -136.2687678316390532, 58.62557946887775273 ) ) ;
#13618=ORIENTED_EDGE ( 'NONE', *, *, #28215, .F. ) ;
#13619=DIRECTION ( 'NONE',  ( 0.000000000000000000, 9.598803233738333010E-14, 1.000000000000000000 ) ) ;
#13620=VECTOR ( 'NONE', #25207, 999.9999999999998863 ) ;
#13623=CIRCLE ( 'NONE', #42986, 60.00000000000000000 ) ;
#13625=LINE ( 'NONE', #25970, #21534 ) ;
#13626=ORIENTED_EDGE ( 'NONE', *, *, #35004, .F. ) ;
#13630=CARTESIAN_POINT ( 'NONE',  ( -330.4913330509368166, -83.33976666099020747, -44.57752413667996194 ) ) ;
#13633=LINE ( 'NONE', #12845, #22154 ) ;
#13642=ORIENTED_EDGE ( 'NONE', *, *, #47140, .F. ) ;
#13644=ORIENTED_EDGE ( 'NONE', *, *, #25660, .T. ) ;
#13646=FACE_OUTER_BOUND ( 'NONE', #12537, .T. ) ;
#13647=FACE_OUTER_BOUND ( 'NONE', #24347, .T. ) ;
#13657=CARTESIAN_POINT ( 'NONE',  ( -339.1964088526558498, -167.3305728129742249, 39.49849221029288060 ) ) ;
#13660=EDGE_LOOP ( 'NONE', ( #3303, #41834, #49728, #24493 ) ) ;
#13662=ADVANCED_FACE ( 'NONE', ( #51289 ), #3198, .F. ) ;
#13664=EDGE_CURVE ( 'NONE', #43748, #19848, #32775, .T. ) ;
#13665=AXIS2_PLACEMENT_3D ( 'NONE', #22577, #10463, #19142 ) ;
#13666=DIRECTION ( 'NONE',  ( 0.000000000000000000, 0.9709418174260519008, -0.2393156642875582940 ) ) ;
#13667=PLANE ( 'NONE',  #3071 ) ;
#13669=CARTESIAN_POINT ( 'NONE',  ( -330.4913330509368166, -157.1712093821534211, -49.66134974749665076 ) ) ;
#13672=CARTESIAN_POINT ( 'NONE',  ( -332.3517673607765914, -64.50000000000000000, -2.632288850093980503 ) ) ;
#13678=LINE ( 'NONE', #21833, #20859 ) ;
#13679=LINE ( 'NONE', #25250, #35853 ) ;
#13684=VECTOR ( 'NONE', #1161, 1000.000000000000000 ) ;
#13689=VERTEX_POINT ( 'NONE', #47344 ) ;
#13691=LINE ( 'NONE', #46031, #8126 ) ;
#13695=AXIS2_PLACEMENT_3D ( 'NONE', #40759, #48928, #20277 ) ;
#13698=CARTESIAN_POINT ( 'NONE',  ( -332.3517673607765914, -165.9166037625627439, 41.09453333279358134 ) ) ;
#13699=PLANE ( 'NONE',  #33825 ) ;
#13705=CARTESIAN_POINT ( 'NONE',  ( -330.4913330509368166, -180.9052250602809693, -13.63415328425256945 ) ) ;
#13706=CIRCLE ( 'NONE', #23790, 60.00000000000000000 ) ;
#13712=VECTOR ( 'NONE', #42585, 1000.000000000000000 ) ;
#13715=VECTOR ( 'NONE', #13716, 1000.000000000000227 ) ;
#13716=DIRECTION ( 'NONE',  ( -0.000000000000000000, -0.1205366802553268363, -0.9927088740980534176 ) ) ;
#13721=CYLINDRICAL_SURFACE ( 'NONE', #33453, 5.000000000000001776 ) ;
#13722=EDGE_CURVE ( 'NONE', #33271, #49077, #39943, .T. ) ;
#13723=EDGE_CURVE ( 'NONE', #36786, #38315, #15281, .T. ) ;
#13725=CARTESIAN_POINT ( 'NONE',  ( -339.1964088526558498, -123.5000000000000284, 0.000000000000000000 ) ) ;
#13732=EDGE_LOOP ( 'NONE', ( #15123, #32280, #19041, #373 ) ) ;
#13733=AXIS2_PLACEMENT_3D ( 'NONE', #412, #48540, #4368 ) ;
#13737=VERTEX_POINT ( 'NONE', #31297 ) ;
#13744=ADVANCED_FACE ( 'NONE', ( #36024 ), #27353, .F. ) ;
#13746=EDGE_CURVE ( 'NONE', #27241, #16769, #11063, .T. ) ;
#13748=DIRECTION ( 'NONE',  ( 1.000000000000000000, -0.000000000000000000, -0.000000000000000000 ) ) ;
#13749=ADVANCED_FACE ( 'NONE', ( #23432 ), #3437, .F. ) ;
#13751=VERTEX_POINT ( 'NONE', #35492 ) ;
#13754=ADVANCED_FACE ( 'NONE', ( #51541 ), #15539, .T. ) ;
#13760=LINE ( 'NONE', #34247, #22433 ) ;
#13761=VERTEX_POINT ( 'NONE', #8169 ) ;
#13762=FACE_OUTER_BOUND ( 'NONE', #42865, .T. ) ;
#13774=ORIENTED_EDGE ( 'NONE', *, *, #28314, .T. ) ;
#13776=CARTESIAN_POINT ( 'NONE',  ( -339.1964088526558498, -64.50000000000000000, -0.5000000000000457412 ) ) ;
#13778=ORIENTED_EDGE ( 'NONE', *, *, #18279, .T. ) ;
#13779=ADVANCED_FACE ( 'NONE', ( #1314 ), #5278, .F. ) ;
#13781=ORIENTED_EDGE ( 'NONE', *, *, #15348, .F. ) ;
#13783=ORIENTED_EDGE ( 'NONE', *, *, #31167, .F. ) ;
#13785=CARTESIAN_POINT ( 'NONE',  ( -336.3521761649654422, -158.3591674452439122, -47.62880233550485087 ) ) ;
#13787=CIRCLE ( 'NONE', #29720, 60.00000000000000000 ) ;
#13788=EDGE_CURVE ( 'NONE', #41973, #27368, #12880, .T. ) ;
#13791=DIRECTION ( 'NONE',  ( 1.000000000000000000, -0.000000000000000000, -0.000000000000000000 ) ) ;
#13792=DIRECTION ( 'NONE',  ( -0.000000000000000000, -0.2393156642875482742, 0.9709418174260544543 ) ) ;
#13794=EDGE_LOOP ( 'NONE', ( #51810, #4944, #5868, #45662 ) ) ;
#13796=ADVANCED_FACE ( 'NONE', ( #28116 ), #44166, .F. ) ;
#13797=ORIENTED_EDGE ( 'NONE', *, *, #32558, .T. ) ;
#13800=EDGE_CURVE ( 'NONE', #17216, #13387, #25238, .T. ) ;
#13803=ORIENTED_EDGE ( 'NONE', *, *, #5757, .T. ) ;
#13805=ADVANCED_FACE ( 'NONE', ( #8684 ), #36272, .F. ) ;
#13808=FACE_OUTER_BOUND ( 'NONE', #5065, .T. ) ;
#13811=EDGE_CURVE ( 'NONE', #44417, #39056, #44960, .T. ) ;
#13813=PLANE ( 'NONE',  #39226 ) ;
#13814=EDGE_CURVE ( 'NONE', #45414, #34872, #21295, .T. ) ;
#13817=EDGE_LOOP ( 'NONE', ( #46826, #9716, #21865, #13210 ) ) ;
#13818=DIRECTION ( 'NONE',  ( -1.000000000000000000, -0.000000000000000000, 0.000000000000000000 ) ) ;
#13820=EDGE_CURVE ( 'NONE', #4093, #11150, #32849, .T. ) ;
#13825=ORIENTED_EDGE ( 'NONE', *, *, #6628, .T. ) ;
#13826=AXIS2_PLACEMENT_3D ( 'NONE', #36536, #534, #27361 ) ;
#13834=PLANE ( 'NONE',  #46296 ) ;
#13835=DIRECTION ( 'NONE',  ( -0.000000000000000000, -0.4647231720437695057, -0.8854560256532093554 ) ) ;
#13838=CARTESIAN_POINT ( 'NONE',  ( -180.0000000000000568, -123.5000000000000284, -20.00000000000002132 ) ) ;
#13843=VERTEX_POINT ( 'NONE', #803 ) ;
#13851=CARTESIAN_POINT ( 'NONE',  ( -305.0000000000000568, -164.4944191672036311, -43.81161486573634534 ) ) ;
#13852=CARTESIAN_POINT ( 'NONE',  ( -336.3521761649654422, -111.9361751271348879, -57.91551518289410438 ) ) ;
#13853=ORIENTED_EDGE ( 'NONE', *, *, #3538, .F. ) ;
#13859=FACE_OUTER_BOUND ( 'NONE', #38407, .T. ) ;
#13861=CARTESIAN_POINT ( 'NONE',  ( -340.0000000000000568, -168.5000000000000284, 0.000000000000000000 ) ) ;
#13862=DIRECTION ( 'NONE',  ( -0.000000000000000000, 0.4647231720437789981, 0.8854560256532044704 ) ) ;
#13863=ORIENTED_EDGE ( 'NONE', *, *, #24102, .T. ) ;
#13874=CARTESIAN_POINT ( 'NONE',  ( -336.3521761649654422, -123.5000000000000284, 0.000000000000000000 ) ) ;
#13881=CARTESIAN_POINT ( 'NONE',  ( -332.3517673607765914, -123.5000000000000284, 0.000000000000000000 ) ) ;
#13883=EDGE_LOOP ( 'NONE', ( #41043, #32424, #38076, #20000 ) ) ;
#13885=VECTOR ( 'NONE', #46008, 1000.000000000000000 ) ;
#13891=ORIENTED_EDGE ( 'NONE', *, *, #50713, .T. ) ;
#13892=FACE_OUTER_BOUND ( 'NONE', #36566, .T. ) ;
#13895=CARTESIAN_POINT ( 'NONE',  ( -330.4913330509368166, -109.6270296344164308, -58.37414404713478433 ) ) ;
#13898=CARTESIAN_POINT ( 'NONE',  ( -332.3517673607765914, -66.84438072661991725, -16.67542351306652648 ) ) ;
#13899=DIRECTION ( 'NONE',  ( -1.000000000000000000, 0.000000000000000000, 0.000000000000000000 ) ) ;
#13903=VECTOR ( 'NONE', #43144, 1000.000000000000000 ) ;
#13904=VECTOR ( 'NONE', #13445, 1000.000000000000000 ) ;
#13907=EDGE_LOOP ( 'NONE', ( #35196, #46135, #46115, #41747 ) ) ;
#13909=VERTEX_POINT ( 'NONE', #41510 ) ;
#13914=AXIS2_PLACEMENT_3D ( 'NONE', #9370, #45380, #25396 ) ;
#13918=DIRECTION ( 'NONE',  ( 1.000000000000000000, -0.000000000000000000, -0.000000000000000000 ) ) ;
#13922=CIRCLE ( 'NONE', #28150, 60.00000000000000000 ) ;
#13923=PLANE ( 'NONE',  #9111 ) ;
#13928=FACE_OUTER_BOUND ( 'NONE', #35056, .T. ) ;
#13941=DIRECTION ( 'NONE',  ( 1.000000000000000000, -4.051632851310755856E-17, -7.719741424018455803E-17 ) ) ;
#13942=CARTESIAN_POINT ( 'NONE',  ( -336.3521761649654422, -123.5000000000000284, 0.000000000000000000 ) ) ;
#13943=CARTESIAN_POINT ( 'NONE',  ( -330.4913330509368166, -175.5095439275173419, 27.86139516340933042 ) ) ;
#13948=FACE_OUTER_BOUND ( 'NONE', #11923, .T. ) ;
#13949=CARTESIAN_POINT ( 'NONE',  ( 0.000000000000000000, -102.5783116644897888, 55.16595831843925879 ) ) ;
#13950=ORIENTED_EDGE ( 'NONE', *, *, #5431, .F. ) ;
#13951=AXIS2_PLACEMENT_3D ( 'NONE', #8965, #815, #44449 ) ;
#13952=DIRECTION ( 'NONE',  ( 1.043714542225393381E-14, -0.000000000000000000, 1.000000000000000000 ) ) ;
#13956=ORIENTED_EDGE ( 'NONE', *, *, #17602, .T. ) ;
#13957=VECTOR ( 'NONE', #39389, 1000.000000000000000 ) ;
#13959=CARTESIAN_POINT ( 'NONE',  ( -330.4913330509368166, -167.3305728129743102, 39.49849221029282376 ) ) ;
#13962=VERTEX_POINT ( 'NONE', #6301 ) ;
#13963=LINE ( 'NONE', #9251, #13904 ) ;
#13964=CARTESIAN_POINT ( 'NONE',  ( -339.1964088526558498, -178.4886558749180949, 21.38919645685277970 ) ) ;
#13967=LINE ( 'NONE', #5315, #36700 ) ;
#13969=ADVANCED_FACE ( 'NONE', ( #13928 ), #6571, .T. ) ;
#13970=VECTOR ( 'NONE', #31732, 1000.000000000000000 ) ;
#13975=ORIENTED_EDGE ( 'NONE', *, *, #17246, .F. ) ;
#13976=VECTOR ( 'NONE', #43092, 1000.000000000000000 ) ;
#13979=EDGE_CURVE ( 'NONE', #19422, #34734, #29951, .T. ) ;
#13980=PLANE ( 'NONE',  #16234 ) ;
#13983=VECTOR ( 'NONE', #17959, 1000.000000000000000 ) ;
#13985=EDGE_CURVE ( 'NONE', #39919, #31214, #10237, .T. ) ;
#13987=EDGE_LOOP ( 'NONE', ( #20426, #22401, #46762, #41062 ) ) ;
#13989=VECTOR ( 'NONE', #2057, 1000.000000000000000 ) ;
#13994=ORIENTED_EDGE ( 'NONE', *, *, #12434, .F. ) ;
#13999=EDGE_LOOP ( 'NONE', ( #8584, #23369, #40528, #20372 ) ) ;
#14001=CARTESIAN_POINT ( 'NONE',  ( -336.3521761649654422, -101.0520950768976149, 54.58714071513087873 ) ) ;
#14002=ORIENTED_EDGE ( 'NONE', *, *, #26895, .T. ) ;
#14003=CYLINDRICAL_SURFACE ( 'NONE', #33098, 15.24495751795539000 ) ;
#14004=ORIENTED_EDGE ( 'NONE', *, *, #39321, .F. ) ;
#14005=VECTOR ( 'NONE', #3818, 1000.000000000000114 ) ;
#14006=CARTESIAN_POINT ( 'NONE',  ( -336.3521761649654422, -93.75055682584159911, 51.01861988938794923 ) ) ;
#14007=DIRECTION ( 'NONE',  ( 1.000000000000000000, -0.000000000000000000, -0.000000000000000000 ) ) ;
#14008=PLANE ( 'NONE',  #39153 ) ;
#14010=CIRCLE ( 'NONE', #14847, 60.00000000000000000 ) ;
#14011=ORIENTED_EDGE ( 'NONE', *, *, #32944, .F. ) ;
#14013=AXIS2_PLACEMENT_3D ( 'NONE', #31334, #38700, #38452 ) ;
#14015=ORIENTED_EDGE ( 'NONE', *, *, #14509, .F. ) ;
#14029=VERTEX_POINT ( 'NONE', #22594 ) ;
#14030=AXIS2_PLACEMENT_3D ( 'NONE', #36283, #8178, #47874 ) ;
#14033=ADVANCED_FACE ( 'NONE', ( #18394 ), #38083, .F. ) ;
#14035=DIRECTION ( 'NONE',  ( 0.000000000000000000, 0.000000000000000000, 1.000000000000000000 ) ) ;
#14036=ADVANCED_FACE ( 'NONE', ( #30461 ), #14198, .F. ) ;
#14042=ORIENTED_EDGE ( 'NONE', *, *, #49179, .F. ) ;
#14045=ORIENTED_EDGE ( 'NONE', *, *, #45769, .F. ) ;
#14049=ADVANCED_FACE ( 'NONE', ( #49674 ), #13667, .F. ) ;
#14056=ORIENTED_EDGE ( 'NONE', *, *, #259, .F. ) ;
#14059=AXIS2_PLACEMENT_3D ( 'NONE', #6288, #3563, #51669 ) ;
#14061=CARTESIAN_POINT ( 'NONE',  ( -339.1964088526558498, -122.9999999999993747, 59.00000000000002132 ) ) ;
#14064=ORIENTED_EDGE ( 'NONE', *, *, #42836, .T. ) ;
#14073=VERTEX_POINT ( 'NONE', #41790 ) ;
#14074=VECTOR ( 'NONE', #48609, 999.9999999999998863 ) ;
#14076=ORIENTED_EDGE ( 'NONE', *, *, #4263, .F. ) ;
#14077=CARTESIAN_POINT ( 'NONE',  ( -336.3521761649654422, -73.44864141332200802, 31.34948880313848107 ) ) ;
#14079=DIRECTION ( 'NONE',  ( -0.000000000000000000, 0.5680647467311656929, 0.8229838658936495799 ) ) ;
#14081=LINE ( 'NONE', #2250, #14494 ) ;
#14083=EDGE_LOOP ( 'NONE', ( #27054, #19455, #3727, #7281 ) ) ;
#14084=DIRECTION ( 'NONE',  ( 0.000000000000000000, -0.5680647467311457088, 0.8229838658936633466 ) ) ;
#14087=ORIENTED_EDGE ( 'NONE', *, *, #10136, .T. ) ;
#14089=AXIS2_PLACEMENT_3D ( 'NONE', #12442, #43481, #8245 ) ;
#14090=AXIS2_PLACEMENT_3D ( 'NONE', #17886, #33899, #6060 ) ;
#14092=EDGE_LOOP ( 'NONE', ( #41357, #49937, #24539, #11069 ) ) ;
#14100=LINE ( 'NONE', #9626, #51790 ) ;
#14104=AXIS2_PLACEMENT_3D ( 'NONE', #387, #15668, #31682 ) ;
#14106=CARTESIAN_POINT ( 'NONE',  ( -339.1964088526558498, -63.87926739338324467, 6.735595255825790773 ) ) ;
#14111=ORIENTED_EDGE ( 'NONE', *, *, #28881, .F. ) ;
#14122=LINE ( 'NONE', #26439, #50051 ) ;
#14123=ORIENTED_EDGE ( 'NONE', *, *, #33253, .F. ) ;
#14124=EDGE_LOOP ( 'NONE', ( #34654, #43783, #27098, #25702 ) ) ;
#14125=EDGE_CURVE ( 'NONE', #32017, #44417, #51231, .T. ) ;
#14132=CARTESIAN_POINT ( 'NONE',  ( -332.3517673607765914, -123.5000000000000284, 0.000000000000000000 ) ) ;
#14135=ORIENTED_EDGE ( 'NONE', *, *, #21040, .F. ) ;
#14137=ADVANCED_FACE ( 'NONE', ( #47287 ), #18895, .F. ) ;
#14144=ORIENTED_EDGE ( 'NONE', *, *, #25133, .F. ) ;
#14146=ORIENTED_EDGE ( 'NONE', *, *, #17032, .T. ) ;
#14149=FACE_OUTER_BOUND ( 'NONE', #31369, .T. ) ;
#14155=ORIENTED_EDGE ( 'NONE', *, *, #16851, .T. ) ;
#14158=CARTESIAN_POINT ( 'NONE',  ( -339.1964088526558498, -95.17484985463171654, -52.89315522109019696 ) ) ;
#14165=LINE ( 'NONE', #17074, #29685 ) ;
#14166=CARTESIAN_POINT ( 'NONE',  ( -330.4913330509368166, -74.40671499923438148, -34.49419324804681253 ) ) ;
#14169=PLANE ( 'NONE',  #27345 ) ;
#14175=VECTOR ( 'NONE', #34801, 1000.000000000000114 ) ;
#14176=AXIS2_PLACEMENT_3D ( 'NONE', #10236, #18894, #50204 ) ;
#14182=ORIENTED_EDGE ( 'NONE', *, *, #27234, .T. ) ;
#14184=CARTESIAN_POINT ( 'NONE',  ( -330.0000000000000568, -123.5000000000000284, 0.000000000000000000 ) ) ;
#14188=CARTESIAN_POINT ( 'NONE',  ( -336.3521761649654422, -123.5000000000000284, 0.000000000000000000 ) ) ;
#14189=ORIENTED_EDGE ( 'NONE', *, *, #22742, .F. ) ;
#14190=EDGE_CURVE ( 'NONE', #37305, #2972, #30979, .T. ) ;
#14191=AXIS2_PLACEMENT_3D ( 'NONE', #8319, #11982, #15956 ) ;
#14192=DIRECTION ( 'NONE',  ( -0.000000000000000000, 0.6631226582408039638, 0.7485107481710934207 ) ) ;
#14193=VERTEX_POINT ( 'NONE', #27028 ) ;
#14194=LINE ( 'NONE', #42025, #29208 ) ;
#14196=LINE ( 'NONE', #6297, #5819 ) ;
#14198=PLANE ( 'NONE',  #9679 ) ;
#14206=CIRCLE ( 'NONE', #11675, 60.00000000000000000 ) ;
#14207=EDGE_LOOP ( 'NONE', ( #2417, #9207, #22009, #5045 ) ) ;
#14208=CARTESIAN_POINT ( 'NONE',  ( -332.3517673607765914, -67.40061919120938683, 18.46045550523129819 ) ) ;
#14216=CARTESIAN_POINT ( 'NONE',  ( -332.3517673607765914, -168.7445418633863596, -37.90245108779149064 ) ) ;
#14220=CARTESIAN_POINT ( 'NONE',  ( -336.3521761649654422, -173.5513585866778214, -31.34948880313881503 ) ) ;
#14222=CARTESIAN_POINT ( 'NONE',  ( -336.3521761649654422, -80.42027357919624819, -40.34602258462219027 ) ) ;
#14224=ORIENTED_EDGE ( 'NONE', *, *, #24584, .T. ) ;
#14236=AXIS2_PLACEMENT_3D ( 'NONE', #28816, #6220, #29602 ) ;
#14243=PLANE ( 'NONE',  #15962 ) ;
#14245=CARTESIAN_POINT ( 'NONE',  ( -330.0000000000000568, -123.5000000000000284, 0.000000000000000000 ) ) ;
#14254=VECTOR ( 'NONE', #18573, 1000.000000000000000 ) ;
#14265=CARTESIAN_POINT ( 'NONE',  ( -336.3521761649654422, -181.7525362123217292, 9.724760635742144999 ) ) ;
#14279=EDGE_CURVE ( 'NONE', #12905, #39518, #48313, .T. ) ;
#14280=DIRECTION ( 'NONE',  ( 0.000000000000000000, 1.000000000000000000, -3.491481338843133355E-15 ) ) ;
#14283=DIRECTION ( 'NONE',  ( -0.000000000000000000, -0.2393156642875615969, -0.9709418174260511236 ) ) ;
#14285=EDGE_CURVE ( 'NONE', #4817, #23416, #36210, .T. ) ;
#14292=AXIS2_PLACEMENT_3D ( 'NONE', #5340, #20307, #45294 ) ;
#14297=DIRECTION ( 'NONE',  ( -1.000000000000000000, 0.000000000000000000, -0.000000000000000000 ) ) ;
#14302=ORIENTED_EDGE ( 'NONE', *, *, #48751, .F. ) ;
#14304=EDGE_CURVE ( 'NONE', #34791, #19790, #36996, .T. ) ;
#14306=EDGE_LOOP ( 'NONE', ( #9048, #45523, #22142, #46659 ) ) ;
#14312=CARTESIAN_POINT ( 'NONE',  ( -332.3517673607765914, -123.5000000000000284, 0.000000000000000000 ) ) ;
#14314=VERTEX_POINT ( 'NONE', #40401 ) ;
#14325=FACE_OUTER_BOUND ( 'NONE', #3276, .T. ) ;
#14326=VECTOR ( 'NONE', #45795, 1000.000000000000000 ) ;
#14327=VECTOR ( 'NONE', #18233, 1000.000000000000000 ) ;
#14333=DIRECTION ( 'NONE',  ( -1.000000000000000000, 0.000000000000000000, 0.000000000000000000 ) ) ;
#14335=ORIENTED_EDGE ( 'NONE', *, *, #10062, .T. ) ;
#14338=EDGE_LOOP ( 'NONE', ( #44953, #37118, #47559, #19551 ) ) ;
#14339=ADVANCED_FACE ( 'NONE', ( #8880 ), #24917, .T. ) ;
#14340=ORIENTED_EDGE ( 'NONE', *, *, #39930, .T. ) ;
#14341=CARTESIAN_POINT ( 'NONE',  ( -336.3521761649654422, -77.59233547837267508, 37.15394033962009246 ) ) ;
#14342=EDGE_CURVE ( 'NONE', #25441, #10943, #4958, .T. ) ;
#14346=EDGE_CURVE ( 'NONE', #13514, #18828, #5216, .T. ) ;
#14353=LINE ( 'NONE', #43504, #33059 ) ;
#14358=VERTEX_POINT ( 'NONE', #3001 ) ;
#14362=DIRECTION ( 'NONE',  ( 1.000000000000000000, -0.000000000000000000, -0.000000000000000000 ) ) ;
#14363=CARTESIAN_POINT ( 'NONE',  ( -336.3521761649654422, -149.4733471526596134, 53.00046796564699036 ) ) ;
#14364=ORIENTED_EDGE ( 'NONE', *, *, #20088, .F. ) ;
#14370=EDGE_LOOP ( 'NONE', ( #19562, #14335, #20704, #11055 ) ) ;
#14373=VECTOR ( 'NONE', #42683, 1000.000000000000114 ) ;
#14375=CARTESIAN_POINT ( 'NONE',  ( -336.3521761649654422, -80.37812621821328207, -41.71934804796994456 ) ) ;
#14376=LINE ( 'NONE', #51177, #5194 ) ;
#14379=EDGE_CURVE ( 'NONE', #23944, #3885, #48311, .T. ) ;
#14381=ADVANCED_FACE ( 'NONE', ( #17566 ), #31116, .F. ) ;
#14384=VERTEX_POINT ( 'NONE', #38991 ) ;
#14388=EDGE_CURVE ( 'NONE', #45944, #17630, #19043, .T. ) ;
#14392=DIRECTION ( 'NONE',  ( 1.000000000000000000, -0.000000000000000000, -0.000000000000000000 ) ) ;
#14394=ORIENTED_EDGE ( 'NONE', *, *, #50887, .T. ) ;
#14398=EDGE_CURVE ( 'NONE', #28486, #23944, #5740, .T. ) ;
#14400=VECTOR ( 'NONE', #4914, 1000.000000000000114 ) ;
#14401=ORIENTED_EDGE ( 'NONE', *, *, #30458, .F. ) ;
#14416=CARTESIAN_POINT ( 'NONE',  ( -332.3517673607765914, -93.75055682584159911, 51.01861988938794923 ) ) ;
#14421=EDGE_CURVE ( 'NONE', #2171, #41684, #33321, .T. ) ;
#14424=AXIS2_PLACEMENT_3D ( 'NONE', #9401, #9656, #13593 ) ;
#14429=EDGE_LOOP ( 'NONE', ( #21958, #30085, #45470, #16901 ) ) ;
#14431=PLANE ( 'NONE',  #9175 ) ;
#14433=CARTESIAN_POINT ( 'NONE',  ( -305.0000000000000568, -123.5000000000000284, -20.00000000000001066 ) ) ;
#14435=CARTESIAN_POINT ( 'NONE',  ( -336.3521761649654422, -126.1322888500942270, -59.00000000000001421 ) ) ;
#14437=PLANE ( 'NONE',  #23495 ) ;
#14441=ORIENTED_EDGE ( 'NONE', *, *, #43976, .F. ) ;
#14443=CARTESIAN_POINT ( 'NONE',  ( -336.3521761649654422, -140.4009141470556870, -57.57047073799078873 ) ) ;
#14446=EDGE_CURVE ( 'NONE', #232, #51884, #10894, .T. ) ;
#14459=PLANE ( 'NONE',  #13039 ) ;
#14461=CARTESIAN_POINT ( 'NONE',  ( -305.0000000000000568, -111.7106844931459761, -58.83036664750484590 ) ) ;
#14464=PLANE ( 'NONE',  #31652 ) ;
#14466=EDGE_LOOP ( 'NONE', ( #1231, #3427, #49212, #20497 ) ) ;
#14467=ORIENTED_EDGE ( 'NONE', *, *, #25595, .F. ) ;
#14474=LINE ( 'NONE', #38375, #2034 ) ;
#14476=PLANE ( 'NONE',  #26574 ) ;
#14478=VECTOR ( 'NONE', #29382, 1000.000000000000114 ) ;
#14482=DIRECTION ( 'NONE',  ( 0.000000000000000000, 0.000000000000000000, -1.000000000000000000 ) ) ;
#14483=CARTESIAN_POINT ( 'NONE',  ( -332.3517673607765914, -180.1556192733800117, 16.67542351306693149 ) ) ;
#14488=DIRECTION ( 'NONE',  ( -0.000000000000000000, 1.000000000000000000, -0.000000000000000000 ) ) ;
#14494=VECTOR ( 'NONE', #25897, 1000.000000000000000 ) ;
#14497=VECTOR ( 'NONE', #44241, 1000.000000000000000 ) ;
#14500=LINE ( 'NONE', #51032, #5266 ) ;
#14504=EDGE_LOOP ( 'NONE', ( #25439, #47748, #44519, #2033 ) ) ;
#14506=ORIENTED_EDGE ( 'NONE', *, *, #50726, .T. ) ;
#14509=EDGE_CURVE ( 'NONE', #26098, #7181, #13922, .T. ) ;
#14513=ORIENTED_EDGE ( 'NONE', *, *, #15402, .F. ) ;
#14515=LINE ( 'NONE', #27090, #43492 ) ;
#14518=CARTESIAN_POINT ( 'NONE',  ( -336.3521761649654422, -173.5513585866778214, -31.34948880313881503 ) ) ;
#14519=ORIENTED_EDGE ( 'NONE', *, *, #44887, .T. ) ;
#14522=LINE ( 'NONE', #26592, #38974 ) ;
#14539=DIRECTION ( 'NONE',  ( 0.000000000000000000, 0.000000000000000000, 1.000000000000000000 ) ) ;
#14541=DIRECTION ( 'NONE',  ( 0.000000000000000000, -0.7485107481711046340, -0.6631226582407911962 ) ) ;
#14544=CARTESIAN_POINT ( 'NONE',  ( -339.1964088526558498, -64.86990808808704401, 6.615309698014191220 ) ) ;
#14546=CARTESIAN_POINT ( 'NONE',  ( -332.3517673607765914, -93.31268025388605736, 51.85292399224828586 ) ) ;
#14547=CARTESIAN_POINT ( 'NONE',  ( -330.4913330509368166, -171.7720157143604069, -33.92731199008473197 ) ) ;
#14549=AXIS2_PLACEMENT_3D ( 'NONE', #51509, #30491, #14482 ) ;
#14551=LINE ( 'NONE', #38699, #49092 ) ;
#14553=AXIS2_PLACEMENT_3D ( 'NONE', #3489, #35541, #40257 ) ;
#14555=LINE ( 'NONE', #42132, #17051 ) ;
#14556=ORIENTED_EDGE ( 'NONE', *, *, #2601, .T. ) ;
#14565=PLANE ( 'NONE',  #12847 ) ;
#14569=ORIENTED_EDGE ( 'NONE', *, *, #3479, .T. ) ;
#14572=EDGE_CURVE ( 'NONE', #2925, #32843, #11664, .T. ) ;
#14577=ORIENTED_EDGE ( 'NONE', *, *, #50340, .T. ) ;
#14579=LINE ( 'NONE', #23239, #18269 ) ;
#14584=ORIENTED_EDGE ( 'NONE', *, *, #41744, .T. ) ;
#14587=LINE ( 'NONE', #11665, #39106 ) ;
#14589=VERTEX_POINT ( 'NONE', #4047 ) ;
#14591=LINE ( 'NONE', #43206, #34223 ) ;
#14592=ADVANCED_FACE ( 'NONE', ( #28456 ), #7723, .F. ) ;
#14593=CARTESIAN_POINT ( 'NONE',  ( -332.3517673607765914, -86.34605966037949543, -45.90766452162698386 ) ) ;
#14596=VERTEX_POINT ( 'NONE', #3776 ) ;
#14599=ORIENTED_EDGE ( 'NONE', *, *, #30745, .T. ) ;
#14601=PLANE ( 'NONE',  #19448 ) ;
#14604=CARTESIAN_POINT ( 'NONE',  ( -332.3517673607765914, -123.5000000000000284, 0.000000000000000000 ) ) ;
#14606=FACE_OUTER_BOUND ( 'NONE', #5364, .T. ) ;
#14609=LINE ( 'NONE', #51154, #47439 ) ;
#14617=ORIENTED_EDGE ( 'NONE', *, *, #14898, .F. ) ;
#14628=VECTOR ( 'NONE', #4111, 1000.000000000000000 ) ;
#14634=VERTEX_POINT ( 'NONE', #9029 ) ;
#14637=EDGE_CURVE ( 'NONE', #15465, #16147, #29249, .T. ) ;
#14638=DIRECTION ( 'NONE',  ( 0.000000000000000000, 0.000000000000000000, -1.000000000000000000 ) ) ;
#14639=DIRECTION ( 'NONE',  ( 0.000000000000000000, -0.2393156642875652051, -0.9709418174260502354 ) ) ;
#14640=PLANE ( 'NONE',  #46520 ) ;
#14645=ORIENTED_EDGE ( 'NONE', *, *, #35188, .T. ) ;
#14647=CARTESIAN_POINT ( 'NONE',  ( -339.1964088526558498, -96.52406086224443982, -52.47426709956138069 ) ) ;
#14663=LINE ( 'NONE', #34873, #45865 ) ;
#14666=DIRECTION ( 'NONE',  ( 0.000000000000000000, 0.5680647467311658039, 0.8229838658936494689 ) ) ;
#14670=LINE ( 'NONE', #13898, #38260 ) ;
#14676=ORIENTED_EDGE ( 'NONE', *, *, #26949, .F. ) ;
#14678=PLANE ( 'NONE',  #41339 ) ;
#14682=PLANE ( 'NONE',  #23684 ) ;
#14688=CARTESIAN_POINT ( 'NONE',  ( -330.4913330509368166, -71.49045607248250178, -27.86139516340898581 ) ) ;
#14689=ORIENTED_EDGE ( 'NONE', *, *, #45842, .T. ) ;
#14692=DIRECTION ( 'NONE',  ( -1.000000000000000000, 1.258058860540606954E-15, 1.036104688092335102E-14 ) ) ;
#14694=DIRECTION ( 'NONE',  ( 0.000000000000000000, 0.000000000000000000, 1.000000000000000000 ) ) ;
#14695=EDGE_CURVE ( 'NONE', #16038, #37674, #12686, .T. ) ;
#14697=AXIS2_PLACEMENT_3D ( 'NONE', #48316, #40161, #28584 ) ;
#14698=DIRECTION ( 'NONE',  ( 1.000000000000000000, -0.000000000000000000, -0.000000000000000000 ) ) ;
#14706=ORIENTED_EDGE ( 'NONE', *, *, #30628, .F. ) ;
#14708=CARTESIAN_POINT ( 'NONE',  ( -336.3521761649654422, -180.1556192733800117, 16.67542351306693149 ) ) ;
#14711=ORIENTED_EDGE ( 'NONE', *, *, #9942, .T. ) ;
#14714=PLANE ( 'NONE',  #4922 ) ;
#14716=PLANE ( 'NONE',  #50189 ) ;
#14717=ORIENTED_EDGE ( 'NONE', *, *, #32888, .T. ) ;
#14720=LINE ( 'NONE', #22339, #51733 ) ;
#14721=ORIENTED_EDGE ( 'NONE', *, *, #48807, .F. ) ;
#14727=DIRECTION ( 'NONE',  ( -0.000000000000000000, 0.000000000000000000, 1.000000000000000000 ) ) ;
#14728=CARTESIAN_POINT ( 'NONE',  ( -332.3517673607765914, -123.5000000000000284, 0.000000000000000000 ) ) ;
#14729=FACE_OUTER_BOUND ( 'NONE', #26441, .T. ) ;
#14731=DIRECTION ( 'NONE',  ( 0.000000000000000000, 0.000000000000000000, 1.000000000000000000 ) ) ;
#14740=DIRECTION ( 'NONE',  ( -1.000000000000000000, -0.000000000000000000, -0.000000000000000000 ) ) ;
#14749=ORIENTED_EDGE ( 'NONE', *, *, #29495, .T. ) ;
#14753=DIRECTION ( 'NONE',  ( -0.000000000000000000, -0.9709418174260534551, -0.2393156642875516327 ) ) ;
#14758=EDGE_LOOP ( 'NONE', ( #48712, #49267, #49566, #15520 ) ) ;
#14761=ADVANCED_FACE ( 'NONE', ( #46849 ), #27141, .T. ) ;
#14763=VERTEX_POINT ( 'NONE', #10064 ) ;
#14764=ORIENTED_EDGE ( 'NONE', *, *, #45781, .F. ) ;
#14770=AXIS2_PLACEMENT_3D ( 'NONE', #50805, #35522, #30823 ) ;
#14776=DIRECTION ( 'NONE',  ( -8.718379230999707126E-17, -0.9709418174260493473, 0.2393156642875685913 ) ) ;
#14784=PLANE ( 'NONE',  #15514 ) ;
#14790=EDGE_LOOP ( 'NONE', ( #11945, #2496, #39432, #44904 ) ) ;
#14795=DIRECTION ( 'NONE',  ( 1.000000000000000000, 0.000000000000000000, -0.000000000000000000 ) ) ;
#14801=CARTESIAN_POINT ( 'NONE',  ( -336.3521761649654422, -120.8677111499054320, 59.00000000000000000 ) ) ;
#14808=CARTESIAN_POINT ( 'NONE',  ( -332.3517673607765914, -182.5000000000000568, 2.632288850093980503 ) ) ;
#14812=EDGE_CURVE ( 'NONE', #22921, #15605, #46585, .T. ) ;
#14814=DIRECTION ( 'NONE',  ( 0.000000000000000000, 3.491481338843133355E-15, 1.000000000000000000 ) ) ;
#14815=CARTESIAN_POINT ( 'NONE',  ( -336.3521761649654422, -176.5004679656469477, -25.97334715265976612 ) ) ;
#14816=EDGE_CURVE ( 'NONE', #27018, #1163, #6383, .T. ) ;
#14819=ADVANCED_FACE ( 'NONE', ( #30800 ), #10569, .F. ) ;
#14820=VECTOR ( 'NONE', #30876, 1000.000000000000000 ) ;
#14821=AXIS2_PLACEMENT_3D ( 'NONE', #49273, #13266, #9576 ) ;
#14822=FACE_BOUND ( 'NONE', #35495, .T. ) ;
#14824=PLANE ( 'NONE',  #24485 ) ;
#14826=AXIS2_PLACEMENT_3D ( 'NONE', #23074, #42520, #35664 ) ;
#14828=ORIENTED_EDGE ( 'NONE', *, *, #47338, .F. ) ;
#14832=DIRECTION ( 'NONE',  ( 0.000000000000000000, -0.7485107481711046340, -0.6631226582407911962 ) ) ;
#14834=CARTESIAN_POINT ( 'NONE',  ( -330.4913330509368166, -123.5000000000000284, 0.000000000000000000 ) ) ;
#14836=ORIENTED_EDGE ( 'NONE', *, *, #32944, .T. ) ;
#14840=DIRECTION ( 'NONE',  ( 0.000000000000000000, -0.9927088740980538617, 0.1205366802553232974 ) ) ;
#14841=ORIENTED_EDGE ( 'NONE', *, *, #42916, .T. ) ;
#14847=AXIS2_PLACEMENT_3D ( 'NONE', #42844, #29527, #21916 ) ;
#14848=DIRECTION ( 'NONE',  ( -0.000000000000000000, 0.8229838658936634577, 0.5680647467311457088 ) ) ;
#14857=ORIENTED_EDGE ( 'NONE', *, *, #16642, .T. ) ;
#14863=VECTOR ( 'NONE', #18921, 999.9999999999998863 ) ;
#14872=VECTOR ( 'NONE', #39693, 1000.000000000000114 ) ;
#14873=ORIENTED_EDGE ( 'NONE', *, *, #40757, .T. ) ;
#14883=ORIENTED_EDGE ( 'NONE', *, *, #10579, .T. ) ;
#14897=LINE ( 'NONE', #46683, #48957 ) ;
#14898=EDGE_CURVE ( 'NONE', #4373, #43725, #2438, .T. ) ;
#14904=ORIENTED_EDGE ( 'NONE', *, *, #10665, .F. ) ;
#14905=VERTEX_POINT ( 'NONE', #7656 ) ;
#14909=PLANE ( 'NONE',  #9232 ) ;
#14914=EDGE_CURVE ( 'NONE', #30320, #48811, #31051, .T. ) ;
#14919=AXIS2_PLACEMENT_3D ( 'NONE', #7484, #32155, #24015 ) ;
#14920=ORIENTED_EDGE ( 'NONE', *, *, #22815, .F. ) ;
#14928=CARTESIAN_POINT ( 'NONE',  ( -332.3517673607765914, -69.20050475944881896, 25.52576769896171882 ) ) ;
#14933=AXIS2_PLACEMENT_3D ( 'NONE', #29547, #25110, #17493 ) ;
#14939=CARTESIAN_POINT ( 'NONE',  ( -330.4913330509368166, -68.51134412508150717, 21.38919645685156112 ) ) ;
#14943=EDGE_CURVE ( 'NONE', #26571, #46931, #7145, .T. ) ;
#14948=VECTOR ( 'NONE', #8963, 1000.000000000000114 ) ;
#14949=CARTESIAN_POINT ( 'NONE',  ( -332.3517673607765914, -69.26746417191145611, -23.38292116578723068 ) ) ;
#14950=ORIENTED_EDGE ( 'NONE', *, *, #6179, .T. ) ;
#14952=CARTESIAN_POINT ( 'NONE',  ( -339.1964088526558498, -176.3931552210898985, 28.32515014536894071 ) ) ;
#14958=VECTOR ( 'NONE', #27758, 1000.000000000000227 ) ;
#14961=EDGE_CURVE ( 'NONE', #11472, #19701, #47353, .T. ) ;
#14964=LINE ( 'NONE', #19920, #26044 ) ;
#14966=VERTEX_POINT ( 'NONE', #11847 ) ;
#14969=EDGE_LOOP ( 'NONE', ( #41707, #49761, #31013, #46734 ) ) ;
#14972=LINE ( 'NONE', #2863, #32605 ) ;
#14975=LINE ( 'NONE', #22843, #10728 ) ;
#14976=LINE ( 'NONE', #46510, #9667 ) ;
#14977=VERTEX_POINT ( 'NONE', #39446 ) ;
#14979=ORIENTED_EDGE ( 'NONE', *, *, #46567, .T. ) ;
#14983=EDGE_CURVE ( 'NONE', #48057, #36746, #48124, .T. ) ;
#14984=DIRECTION ( 'NONE',  ( -0.000000000000000000, 0.9350162426854194964, 0.3546048870425235200 ) ) ;
#14985=ORIENTED_EDGE ( 'NONE', *, *, #1586, .T. ) ;
#14987=DIRECTION ( 'NONE',  ( -1.000000000000000000, 0.000000000000000000, 0.000000000000000000 ) ) ;
#14988=ORIENTED_EDGE ( 'NONE', *, *, #50363, .F. ) ;
#14998=DIRECTION ( 'NONE',  ( 0.000000000000000000, -3.469446951953614189E-15, 1.000000000000000000 ) ) ;
#15003=EDGE_CURVE ( 'NONE', #8786, #34048, #15551, .T. ) ;
#15004=CARTESIAN_POINT ( 'NONE',  ( -330.4913330509368166, -143.9541802141664562, 55.34326076196094135 ) ) ;
#15005=DIRECTION ( 'NONE',  ( -1.000000000000000000, -0.000000000000000000, 0.000000000000000000 ) ) ;
#15006=EDGE_CURVE ( 'NONE', #49077, #77, #12097, .T. ) ;
#15008=ORIENTED_EDGE ( 'NONE', *, *, #10535, .T. ) ;
#15010=ADVANCED_FACE ( 'NONE', ( #11074 ), #44181, .T. ) ;
#15014=ADVANCED_FACE ( 'NONE', ( #8179 ), #27100, .F. ) ;
#15019=LINE ( 'NONE', #3177, #43840 ) ;
#15020=DIRECTION ( 'NONE',  ( 0.000000000000000000, 0.9927088740980544168, 0.1205366802553199251 ) ) ;
#15026=VERTEX_POINT ( 'NONE', #39958 ) ;
#15031=DIRECTION ( 'NONE',  ( 0.000000000000000000, 0.9927088740980539727, -0.1205366802553233252 ) ) ;
#15035=ADVANCED_FACE ( 'NONE', ( #3981 ), #15050, .T. ) ;
#15040=DIRECTION ( 'NONE',  ( 1.043714542225393381E-14, -0.5680647467311510379, 0.8229838658936596829 ) ) ;
#15041=ORIENTED_EDGE ( 'NONE', *, *, #41504, .T. ) ;
#15045=ORIENTED_EDGE ( 'NONE', *, *, #6179, .F. ) ;
#15046=EDGE_CURVE ( 'NONE', #27857, #29243, #44324, .T. ) ;
#15049=DIRECTION ( 'NONE',  ( 1.000000000000000000, 0.000000000000000000, -0.000000000000000000 ) ) ;
#15050=PLANE ( 'NONE',  #46445 ) ;
#15051=CARTESIAN_POINT ( 'NONE',  ( -336.3521761649654422, -70.03480886230919111, 25.08789112700620194 ) ) ;
#15052=FACE_OUTER_BOUND ( 'NONE', #11727, .T. ) ;
#15058=PLANE ( 'NONE',  #50220 ) ;
#15062=CARTESIAN_POINT ( 'NONE',  ( -332.3517673607765914, -90.77207769297352513, -50.28800156563430335 ) ) ;
#15069=CARTESIAN_POINT ( 'NONE',  ( -336.3521761649654422, -123.5000000000000284, 0.000000000000000000 ) ) ;
#15072=VECTOR ( 'NONE', #28369, 1000.000000000000000 ) ;
#15082=ORIENTED_EDGE ( 'NONE', *, *, #31394, .F. ) ;
#15086=FACE_OUTER_BOUND ( 'NONE', #21712, .T. ) ;
#15092=CARTESIAN_POINT ( 'NONE',  ( -336.3521761649654422, -72.48138011061176655, -29.74944317415788930 ) ) ;
#15093=ORIENTED_EDGE ( 'NONE', *, *, #29796, .T. ) ;
#15094=ORIENTED_EDGE ( 'NONE', *, *, #6452, .T. ) ;
#15095=DIRECTION ( 'NONE',  ( 0.000000000000000000, 0.2393156642875516604, -0.9709418174260535661 ) ) ;
#15099=LINE ( 'NONE', #27412, #14373 ) ;
#15103=EDGE_LOOP ( 'NONE', ( #26753, #23251, #25623, #11752 ) ) ;
#15105=CARTESIAN_POINT ( 'NONE',  ( -339.1964088526558498, -162.2499814621216672, -44.49369547121515467 ) ) ;
#15119=CARTESIAN_POINT ( 'NONE',  ( -339.1964088526558498, -182.0095552316576573, -7.608018572112655420 ) ) ;
#15120=CARTESIAN_POINT ( 'NONE',  ( -336.3521761649654422, -181.8730728925770563, 8.732051761644092025 ) ) ;
#15123=ORIENTED_EDGE ( 'NONE', *, *, #21867, .T. ) ;
#15125=AXIS2_PLACEMENT_3D ( 'NONE', #16124, #39747, #35307 ) ;
#15127=ORIENTED_EDGE ( 'NONE', *, *, #42830, .F. ) ;
#15129=EDGE_CURVE ( 'NONE', #10851, #7810, #38918, .T. ) ;
#15130=DIRECTION ( 'NONE',  ( -0.000000000000000000, 0.9350162426854194964, 0.3546048870425235200 ) ) ;
#15143=ORIENTED_EDGE ( 'NONE', *, *, #31598, .F. ) ;
#15144=DIRECTION ( 'NONE',  ( 1.000000000000000000, -3.091579882402700648E-17, -8.151826190875878101E-17 ) ) ;
#15145=EDGE_LOOP ( 'NONE', ( #15150, #31653, #12385, #21538 ) ) ;
#15149=DIRECTION ( 'NONE',  ( -0.000000000000000000, 0.3546048870425331789, -0.9350162426854158326 ) ) ;
#15150=ORIENTED_EDGE ( 'NONE', *, *, #39785, .T. ) ;
#15151=DIRECTION ( 'NONE',  ( -0.000000000000000000, -1.000000000000000000, -0.000000000000000000 ) ) ;
#15154=VERTEX_POINT ( 'NONE', #33696 ) ;
#15156=VECTOR ( 'NONE', #28513, 1000.000000000000000 ) ;
#15159=DIRECTION ( 'NONE',  ( -0.000000000000000000, -0.3546048870425267951, 0.9350162426854181641 ) ) ;
#15163=FACE_OUTER_BOUND ( 'NONE', #9168, .T. ) ;
#15164=EDGE_LOOP ( 'NONE', ( #42701, #20685, #18225, #29202 ) ) ;
#15167=CARTESIAN_POINT ( 'NONE',  ( -336.3521761649653854, -110.7312321683605916, -58.62557946887767457 ) ) ;
#15168=ORIENTED_EDGE ( 'NONE', *, *, #14190, .T. ) ;
#15176=DIRECTION ( 'NONE',  ( 1.000000000000000000, 0.000000000000000000, -0.000000000000000000 ) ) ;
#15179=ORIENTED_EDGE ( 'NONE', *, *, #26181, .T. ) ;
#15186=PLANE ( 'NONE',  #41640 ) ;
#15199=DIRECTION ( 'NONE',  ( 0.000000000000000000, 2.148744145576605138E-13, -1.000000000000000000 ) ) ;
#15201=FACE_OUTER_BOUND ( 'NONE', #19471, .T. ) ;
#15203=EDGE_LOOP ( 'NONE', ( #8476, #25000, #36593, #35173 ) ) ;
#15204=LINE ( 'NONE', #50960, #40208 ) ;
#15209=EDGE_LOOP ( 'NONE', ( #2603, #45785, #39627, #19644 ) ) ;
#15218=AXIS2_PLACEMENT_3D ( 'NONE', #38837, #30961, #15199 ) ;
#15223=DIRECTION ( 'NONE',  ( 0.000000000000000000, 0.9350162426854169428, 0.3546048870425300148 ) ) ;
#15224=ORIENTED_EDGE ( 'NONE', *, *, #5088, .F. ) ;
#15225=EDGE_CURVE ( 'NONE', #23268, #42035, #15997, .T. ) ;
#15228=PLANE ( 'NONE',  #33997 ) ;
#15231=ORIENTED_EDGE ( 'NONE', *, *, #29077, .F. ) ;
#15232=LINE ( 'NONE', #2876, #2294 ) ;
#15240=VERTEX_POINT ( 'NONE', #201 ) ;
#15243=DIRECTION ( 'NONE',  ( 0.000000000000000000, 0.9927088740980538617, -0.1205366802553232974 ) ) ;
#15250=CARTESIAN_POINT ( 'NONE',  ( -339.1964088526558498, -108.6560878169895403, 58.13482838284700449 ) ) ;
#15251=ORIENTED_EDGE ( 'NONE', *, *, #29793, .F. ) ;
#15255=LINE ( 'NONE', #34954, #34494 ) ;
#15259=VECTOR ( 'NONE', #46156, 1000.000000000000000 ) ;
#15261=DIRECTION ( 'NONE',  ( 1.000000000000000000, 0.000000000000000000, -0.000000000000000000 ) ) ;
#15263=CARTESIAN_POINT ( 'NONE',  ( -330.4913330509368166, -67.57827586672175357, -21.74306257088736061 ) ) ;
#15266=ORIENTED_EDGE ( 'NONE', *, *, #39470, .T. ) ;
#15267=EDGE_CURVE ( 'NONE', #19264, #16302, #51742, .T. ) ;
#15270=VERTEX_POINT ( 'NONE', #44096 ) ;
#15272=ORIENTED_EDGE ( 'NONE', *, *, #6685, .F. ) ;
#15273=VECTOR ( 'NONE', #38018, 1000.000000000000114 ) ;
#15280=DIRECTION ( 'NONE',  ( 1.000000000000000000, -0.000000000000000000, -0.000000000000000000 ) ) ;
#15281=LINE ( 'NONE', #18965, #20204 ) ;
#15282=LINE ( 'NONE', #31298, #7361 ) ;
#15284=VERTEX_POINT ( 'NONE', #12291 ) ;
#15285=EDGE_CURVE ( 'NONE', #51297, #6623, #47799, .T. ) ;
#15290=VERTEX_POINT ( 'NONE', #52007 ) ;
#15293=AXIS2_PLACEMENT_3D ( 'NONE', #35335, #6969, #51914 ) ;
#15294=LINE ( 'NONE', #39201, #11460 ) ;
#15299=ORIENTED_EDGE ( 'NONE', *, *, #23102, .F. ) ;
#15301=ORIENTED_EDGE ( 'NONE', *, *, #10879, .F. ) ;
#15311=ORIENTED_EDGE ( 'NONE', *, *, #26251, .F. ) ;
#15321=CARTESIAN_POINT ( 'NONE',  ( -336.3521761649654422, -166.5797264208035244, 40.34602258462248159 ) ) ;
#15326=ADVANCED_FACE ( 'NONE', ( #30786 ), #24642, .F. ) ;
#15333=DIRECTION ( 'NONE',  ( 0.000000000000000000, 0.8229838658936536877, -0.5680647467311596976 ) ) ;
#15334=ORIENTED_EDGE ( 'NONE', *, *, #29022, .F. ) ;
#15336=DIRECTION ( 'NONE',  ( 0.000000000000000000, 0.9709418174260534551, 0.2393156642875516327 ) ) ;
#15343=DIRECTION ( 'NONE',  ( 0.000000000000000000, -0.8229838658936495799, 0.5680647467311656929 ) ) ;
#15348=EDGE_CURVE ( 'NONE', #36071, #11143, #1514, .T. ) ;
#15351=CARTESIAN_POINT ( 'NONE',  ( -365.0000000000001137, -168.5000000000000284, 5.000000000000001776 ) ) ;
#15357=PLANE ( 'NONE',  #12128 ) ;
#15358=EDGE_LOOP ( 'NONE', ( #9929, #18712, #24159, #20826 ) ) ;
#15359=EDGE_CURVE ( 'NONE', #21361, #13514, #25176, .T. ) ;
#15360=UNCERTAINTY_MEASURE_WITH_UNIT (LENGTH_MEASURE( 1.000000000000000082E-05 ), #35774, 'distance_accuracy_value', 'NONE');
#15363=CARTESIAN_POINT ( 'NONE',  ( -336.3521761649654422, -179.5993808087905279, -18.46045550523168899 ) ) ;
#15369=CARTESIAN_POINT ( 'NONE',  ( -305.0000000000000568, -73.83865025250327108, -33.67120938215323633 ) ) ;
#15370=AXIS2_PLACEMENT_3D ( 'NONE', #18291, #6202, #30603 ) ;
#15371=DIRECTION ( 'NONE',  ( -1.000000000000000000, 0.000000000000000000, 0.000000000000000000 ) ) ;
#15373=EDGE_LOOP ( 'NONE', ( #4566, #15546, #39368, #29987 ) ) ;
#15376=CIRCLE ( 'NONE', #14553, 60.00000000000000000 ) ;
#15385=CARTESIAN_POINT ( 'NONE',  ( -339.1964088526558498, -123.5000000000000284, 0.000000000000000000 ) ) ;
#15387=FACE_OUTER_BOUND ( 'NONE', #3490, .T. ) ;
#15388=VERTEX_POINT ( 'NONE', #17040 ) ;
#15389=EDGE_CURVE ( 'NONE', #12090, #10873, #9150, .T. ) ;
#15398=EDGE_CURVE ( 'NONE', #9161, #49147, #41186, .T. ) ;
#15402=EDGE_CURVE ( 'NONE', #10873, #26098, #44883, .T. ) ;
#15403=DIRECTION ( 'NONE',  ( -1.000000000000000000, 0.000000000000000000, 0.000000000000000000 ) ) ;
#15411=VECTOR ( 'NONE', #40686, 1000.000000000000000 ) ;
#15412=EDGE_CURVE ( 'NONE', #46461, #26719, #33901, .T. ) ;
#15413=CARTESIAN_POINT ( 'NONE',  ( -339.1964088526558498, -167.9936954712156592, -38.74998146212110584 ) ) ;
#15424=CARTESIAN_POINT ( 'NONE',  ( -332.3517673607765914, -64.73342574900661361, 5.491276508483657892 ) ) ;
#15427=EDGE_CURVE ( 'NONE', #30276, #3919, #34351, .T. ) ;
#15428=VECTOR ( 'NONE', #27365, 1000.000000000000000 ) ;
#15429=EDGE_CURVE ( 'NONE', #186, #43501, #38280, .T. ) ;
#15433=EDGE_LOOP ( 'NONE', ( #6826, #2354, #22798, #24010 ) ) ;
#15442=ORIENTED_EDGE ( 'NONE', *, *, #23915, .F. ) ;
#15443=ADVANCED_FACE ( 'NONE', ( #26970 ), #14640, .T. ) ;
#15445=LINE ( 'NONE', #28727, #32295 ) ;
#15446=DIRECTION ( 'NONE',  ( 1.000000000000000000, 0.000000000000000000, 0.000000000000000000 ) ) ;
#15454=DIRECTION ( 'NONE',  ( 0.000000000000000000, 0.000000000000000000, -1.000000000000000000 ) ) ;
#15463=LINE ( 'NONE', #35410, #6950 ) ;
#15465=VERTEX_POINT ( 'NONE', #30923 ) ;
#15466=CARTESIAN_POINT ( 'NONE',  ( -336.3521761649654422, -64.50000000000000000, -1.632288850093980725 ) ) ;
#15470=CARTESIAN_POINT ( 'NONE',  ( -336.3521761649654422, -171.1288023355047585, 34.85916744524404720 ) ) ;
#15472=VERTEX_POINT ( 'NONE', #19105 ) ;
#15474=ORIENTED_EDGE ( 'NONE', *, *, #51284, .F. ) ;
#15477=VECTOR ( 'NONE', #13224, 1000.000000000000000 ) ;
#15479=AXIS2_PLACEMENT_3D ( 'NONE', #8265, #24295, #20341 ) ;
#15495=AXIS2_PLACEMENT_3D ( 'NONE', #36405, #400, #16456 ) ;
#15501=DIRECTION ( 'NONE',  ( 0.000000000000000000, 0.000000000000000000, -1.000000000000000000 ) ) ;
#15503=PLANE ( 'NONE',  #22380 ) ;
#15506=ORIENTED_EDGE ( 'NONE', *, *, #1199, .F. ) ;
#15509=FACE_OUTER_BOUND ( 'NONE', #39824, .T. ) ;
#15510=DIRECTION ( 'NONE',  ( 1.000000000000000000, 0.000000000000000000, -0.000000000000000000 ) ) ;
#15514=AXIS2_PLACEMENT_3D ( 'NONE', #47095, #26075, #6125 ) ;
#15520=ORIENTED_EDGE ( 'NONE', *, *, #25374, .T. ) ;
#15521=ORIENTED_EDGE ( 'NONE', *, *, #34965, .F. ) ;
#15524=DIRECTION ( 'NONE',  ( 0.000000000000000000, 6.753856733136369375E-14, 1.000000000000000000 ) ) ;
#15529=CIRCLE ( 'NONE', #34015, 60.00000000000000000 ) ;
#15531=VERTEX_POINT ( 'NONE', #23032 ) ;
#15533=ORIENTED_EDGE ( 'NONE', *, *, #3578, .T. ) ;
#15534=ADVANCED_FACE ( 'NONE', ( #15163 ), #22782, .F. ) ;
#15536=CARTESIAN_POINT ( 'NONE',  ( -332.3517673607765914, -169.4076645216271402, -37.15394033962039089 ) ) ;
#15537=VERTEX_POINT ( 'NONE', #10692 ) ;
#15539=PLANE ( 'NONE',  #3395 ) ;
#15543=VECTOR ( 'NONE', #9301, 999.9999999999998863 ) ;
#15544=PLANE ( 'NONE',  #24788 ) ;
#15545=CIRCLE ( 'NONE', #7999, 60.00000000000000000 ) ;
#15546=ORIENTED_EDGE ( 'NONE', *, *, #5882, .F. ) ;
#15547=DIRECTION ( 'NONE',  ( 1.000000000000000000, 2.086444717177546192E-17, 8.465038975556398759E-17 ) ) ;
#15549=VECTOR ( 'NONE', #5893, 1000.000000000000000 ) ;
#15550=DIRECTION ( 'NONE',  ( 1.000000000000000000, -0.000000000000000000, -0.000000000000000000 ) ) ;
#15551=LINE ( 'NONE', #11605, #50644 ) ;
#15555=ORIENTED_EDGE ( 'NONE', *, *, #37713, .T. ) ;
#15557=DIRECTION ( 'NONE',  ( -0.000000000000000000, 0.7485107481710999711, -0.6631226582407964143 ) ) ;
#15561=AXIS2_PLACEMENT_3D ( 'NONE', #14834, #38716, #50828 ) ;
#15564=VERTEX_POINT ( 'NONE', #38550 ) ;
#15567=CARTESIAN_POINT ( 'NONE',  ( -339.1964088526558498, -131.1080185721124849, 58.50955523165764305 ) ) ;
#15571=VERTEX_POINT ( 'NONE', #42219 ) ;
#15580=EDGE_CURVE ( 'NONE', #12334, #10851, #34848, .T. ) ;
#15583=CIRCLE ( 'NONE', #25624, 60.00000000000000000 ) ;
#15588=VECTOR ( 'NONE', #37917, 1000.000000000000000 ) ;
#15589=VECTOR ( 'NONE', #14488, 1000.000000000000000 ) ;
#15594=ORIENTED_EDGE ( 'NONE', *, *, #34209, .F. ) ;
#15595=CARTESIAN_POINT ( 'NONE',  ( -336.3521761649654422, -66.84438072661991725, -16.67542351306652648 ) ) ;
#15598=EDGE_CURVE ( 'NONE', #30219, #28004, #43777, .T. ) ;
#15599=CARTESIAN_POINT ( 'NONE',  ( -339.1964088526558498, -64.50000000000000000, 0.4999999999999543698 ) ) ;
#15605=VERTEX_POINT ( 'NONE', #28269 ) ;
#15609=CARTESIAN_POINT ( 'NONE',  ( -332.3517673607765914, -178.6135371030394481, 23.71704087764532076 ) ) ;
#15611=CARTESIAN_POINT ( 'NONE',  ( -336.3521761649654422, -74.01670616005314685, 32.17247266903214609 ) ) ;
#15617=CARTESIAN_POINT ( 'NONE',  ( -336.3521761649654422, -160.6539403396202772, 45.90766452162722544 ) ) ;
#15621=ORIENTED_EDGE ( 'NONE', *, *, #36259, .T. ) ;
#15624=CARTESIAN_POINT ( 'NONE',  ( -339.1964088526558498, -182.5000000000000568, 0.5000000000000457412 ) ) ;
#15626=LINE ( 'NONE', #40032, #45875 ) ;
#15628=FACE_OUTER_BOUND ( 'NONE', #8703, .T. ) ;
#15630=EDGE_CURVE ( 'NONE', #18239, #14029, #20122, .T. ) ;
#15631=DIRECTION ( 'NONE',  ( 1.000000000000000000, 0.000000000000000000, -0.000000000000000000 ) ) ;
#15634=EDGE_LOOP ( 'NONE', ( #40731, #2770, #26377, #38656 ) ) ;
#15635=FACE_OUTER_BOUND ( 'NONE', #19318, .T. ) ;
#15638=VERTEX_POINT ( 'NONE', #39819 ) ;
#15643=CARTESIAN_POINT ( 'NONE',  ( -332.3517673607765914, -77.59233547837267508, 37.15394033962009246 ) ) ;
#15649=VERTEX_POINT ( 'NONE', #19358 ) ;
#15653=ORIENTED_EDGE ( 'NONE', *, *, #25660, .F. ) ;
#15654=EDGE_CURVE ( 'NONE', #16440, #27371, #47990, .T. ) ;
#15656=DIRECTION ( 'NONE',  ( 0.000000000000000000, 0.000000000000000000, 1.000000000000000000 ) ) ;
#15659=VERTEX_POINT ( 'NONE', #35370 ) ;
#15660=DIRECTION ( 'NONE',  ( 1.043714542225393381E-14, 0.000000000000000000, -1.000000000000000000 ) ) ;
#15663=VECTOR ( 'NONE', #22688, 1000.000000000000000 ) ;
#15666=CARTESIAN_POINT ( 'NONE',  ( -332.3517673607765914, -98.41210887299327226, -53.46519113769058151 ) ) ;
#15668=DIRECTION ( 'NONE',  ( 1.000000000000000000, -0.000000000000000000, -0.000000000000000000 ) ) ;
#15671=LINE ( 'NONE', #3048, #69 ) ;
#15674=EDGE_LOOP ( 'NONE', ( #1310, #15822, #759, #2806 ) ) ;
#15676=DIRECTION ( 'NONE',  ( 1.000000000000000000, 0.000000000000000000, 0.000000000000000000 ) ) ;
#15681=CIRCLE ( 'NONE', #29923, 10.00000000000000711 ) ;
#15682=FACE_OUTER_BOUND ( 'NONE', #1103, .T. ) ;
#15683=VECTOR ( 'NONE', #51907, 1000.000000000000227 ) ;
#15684=CARTESIAN_POINT ( 'NONE',  ( -339.1964088526558498, -90.39567187580880159, -48.84008046109142498 ) ) ;
#15685=ORIENTED_EDGE ( 'NONE', *, *, #11202, .T. ) ;
#15690=VERTEX_POINT ( 'NONE', #32209 ) ;
#15691=CARTESIAN_POINT ( 'NONE',  ( 0.000000000000000000, -175.7419055135392227, 27.41866715058277038 ) ) ;
#15692=EDGE_LOOP ( 'NONE', ( #48850, #26011, #4505, #41159 ) ) ;
#15697=DIRECTION ( 'NONE',  ( -0.000000000000000000, -0.4647231720437604574, 0.8854560256532141294 ) ) ;
#15698=EDGE_CURVE ( 'NONE', #15649, #4141, #34758, .T. ) ;
#15703=EDGE_CURVE ( 'NONE', #34344, #18494, #28003, .T. ) ;
#15709=CARTESIAN_POINT ( 'NONE',  ( -339.1964088526558498, -123.5000000000000284, 0.000000000000000000 ) ) ;
#15712=CARTESIAN_POINT ( 'NONE',  ( -332.3517673607765914, -123.5000000000000284, 0.000000000000000000 ) ) ;
#15714=ADVANCED_FACE ( 'NONE', ( #20380 ), #12231, .F. ) ;
#15715=VERTEX_POINT ( 'NONE', #32476 ) ;
#15717=LINE ( 'NONE', #32236, #13970 ) ;
#15721=VECTOR ( 'NONE', #32139, 1000.000000000000000 ) ;
#15724=CARTESIAN_POINT ( 'NONE',  ( -339.1964088526558498, -131.1080185721133660, -58.50955523165751515 ) ) ;
#15725=AXIS2_PLACEMENT_3D ( 'NONE', #39445, #15049, #19477 ) ;
#15730=LINE ( 'NONE', #31739, #43066 ) ;
#15740=LINE ( 'NONE', #30703, #5913 ) ;
#15746=AXIS2_PLACEMENT_3D ( 'NONE', #31806, #20753, #44414 ) ;
#15747=ORIENTED_EDGE ( 'NONE', *, *, #49983, .F. ) ;
#15749=CARTESIAN_POINT ( 'NONE',  ( -305.0000000000000568, -120.8677111499054320, 59.94223098458771659 ) ) ;
#15750=CIRCLE ( 'NONE', #45123, 60.00000000000000000 ) ;
#15751=DIRECTION ( 'NONE',  ( 1.000000000000000000, 7.719741424018497712E-17, 4.051632851310676353E-17 ) ) ;
#15753=ORIENTED_EDGE ( 'NONE', *, *, #47155, .F. ) ;
#15758=VERTEX_POINT ( 'NONE', #32732 ) ;
#15765=ADVANCED_FACE ( 'NONE', ( #33521 ), #45614, .T. ) ;
#15767=AXIS2_PLACEMENT_3D ( 'NONE', #13178, #13952, #1851 ) ;
#15776=CARTESIAN_POINT ( 'NONE',  ( -332.3517673607765914, -166.5797264208035244, 40.34602258462248159 ) ) ;
#15778=CARTESIAN_POINT ( 'NONE',  ( -339.1964088526558498, -65.36517161715286761, -14.84391218300986282 ) ) ;
#15795=DIRECTION ( 'NONE',  ( -1.000000000000000000, -6.921107616850788183E-15, -7.812315528781864579E-15 ) ) ;
#15799=ADVANCED_FACE ( 'NONE', ( #12744 ), #49560, .F. ) ;
#15802=CARTESIAN_POINT ( 'NONE',  ( -336.3521761649654422, -181.7525362123217292, 9.724760635742144999 ) ) ;
#15803=ORIENTED_EDGE ( 'NONE', *, *, #38401, .F. ) ;
#15810=VERTEX_POINT ( 'NONE', #9090 ) ;
#15813=LINE ( 'NONE', #48649, #11546 ) ;
#15814=CARTESIAN_POINT ( 'NONE',  ( -339.1964088526558498, -109.8658467157464571, 57.40522506028071348 ) ) ;
#15818=LINE ( 'NONE', #39686, #9677 ) ;
#15820=DIRECTION ( 'NONE',  ( 1.043714542225393381E-14, 0.8854560256532141294, 0.4647231720437604574 ) ) ;
#15822=ORIENTED_EDGE ( 'NONE', *, *, #3341, .T. ) ;
#15825=DIRECTION ( 'NONE',  ( 0.000000000000000000, -0.6631226582407885317, 0.7485107481711069655 ) ) ;
#15832=LINE ( 'NONE', #23687, #11593 ) ;
#15838=CARTESIAN_POINT ( 'NONE',  ( -330.4913330509368166, -79.66942718702493664, 39.49849221029193558 ) ) ;
#15839=DIRECTION ( 'NONE',  ( -8.718379230999707126E-17, -0.9927088740980551940, -0.1205366802553130001 ) ) ;
#15840=AXIS2_PLACEMENT_3D ( 'NONE', #7848, #23377, #39891 ) ;
#15844=DIRECTION ( 'NONE',  ( -1.000000000000000000, 0.000000000000000000, 0.000000000000000000 ) ) ;
#15845=CARTESIAN_POINT ( 'NONE',  ( -330.4913330509368166, -65.36517161715264024, 14.84391218300897286 ) ) ;
#15859=LINE ( 'NONE', #19772, #36666 ) ;
#15860=ADVANCED_FACE ( 'NONE', ( #44822 ), #13539, .F. ) ;
#15862=ORIENTED_EDGE ( 'NONE', *, *, #21158, .T. ) ;
#15864=VERTEX_POINT ( 'NONE', #37968 ) ;
#15867=DIRECTION ( 'NONE',  ( 0.000000000000000000, -0.9709418174260527890, -0.2393156642875547968 ) ) ;
#15872=VERTEX_POINT ( 'NONE', #46387 ) ;
#15873=AXIS2_PLACEMENT_3D ( 'NONE', #11471, #15176, #11212 ) ;
#15878=DIRECTION ( 'NONE',  ( 0.000000000000000000, 0.8229838658936596829, 0.5680647467311510379 ) ) ;
#15879=CARTESIAN_POINT ( 'NONE',  ( -339.1964088526558498, -79.66942718702553350, -39.49849221029258928 ) ) ;
#15880=EDGE_LOOP ( 'NONE', ( #8923, #19583, #40599, #44234 ) ) ;
#15892=ORIENTED_EDGE ( 'NONE', *, *, #793, .F. ) ;
#15893=CARTESIAN_POINT ( 'NONE',  ( -336.3521761649654422, -87.81784868886214213, 47.06073758877343494 ) ) ;
#15894=VECTOR ( 'NONE', #34086, 1000.000000000000000 ) ;
#15895=DIRECTION ( 'NONE',  ( 0.000000000000000000, 0.9350162426854169428, 0.3546048870425300148 ) ) ;
#15896=LINE ( 'NONE', #47943, #38554 ) ;
#15898=DIRECTION ( 'NONE',  ( -0.000000000000000000, -0.3546048870425267951, 0.9350162426854181641 ) ) ;
#15904=EDGE_CURVE ( 'NONE', #978, #32381, #30335, .T. ) ;
#15911=ORIENTED_EDGE ( 'NONE', *, *, #19299, .T. ) ;
#15915=CARTESIAN_POINT ( 'NONE',  ( -330.4913330509368166, -115.8919814278871598, -58.50955523165758621 ) ) ;
#15919=CARTESIAN_POINT ( 'NONE',  ( -330.4913330509368166, -168.0775241366801254, -40.16023333900968595 ) ) ;
#15923=PLANE ( 'NONE',  #5825 ) ;
#15924=DIRECTION ( 'NONE',  ( 1.000000000000000000, 0.000000000000000000, -0.000000000000000000 ) ) ;
#15926=CARTESIAN_POINT ( 'NONE',  ( -336.3521761649654422, -169.4076645216271402, -37.15394033962039089 ) ) ;
#15931=CARTESIAN_POINT ( 'NONE',  ( -336.3521761649654422, -85.59754891220836726, -45.24454186338619621 ) ) ;
#15940=CARTESIAN_POINT ( 'NONE',  ( -336.3521761649654422, -173.5513585866778214, -31.34948880313881503 ) ) ;
#15941=VERTEX_POINT ( 'NONE', #46134 ) ;
#15946=ORIENTED_EDGE ( 'NONE', *, *, #39419, .T. ) ;
#15951=EDGE_CURVE ( 'NONE', #38828, #4817, #2737, .T. ) ;
#15956=DIRECTION ( 'NONE',  ( 0.000000000000000000, -0.9927088740980556381, -0.1205366802553095307 ) ) ;
#15957=EDGE_LOOP ( 'NONE', ( #20090, #13280, #10656, #30798 ) ) ;
#15958=CARTESIAN_POINT ( 'NONE',  ( -330.4913330509368166, -183.0001959263614424, -7.728304129924260302 ) ) ;
#15959=ORIENTED_EDGE ( 'NONE', *, *, #32729, .F. ) ;
#15960=ORIENTED_EDGE ( 'NONE', *, *, #1154, .T. ) ;
#15962=AXIS2_PLACEMENT_3D ( 'NONE', #6353, #22374, #9071 ) ;
#15973=CARTESIAN_POINT ( 'NONE',  ( -336.3521761649654422, -105.0395444947681369, -56.09938080879045685 ) ) ;
#15974=CARTESIAN_POINT ( 'NONE',  ( -336.3521761649653854, -84.94915232962709695, -45.97643030831888211 ) ) ;
#15975=ORIENTED_EDGE ( 'NONE', *, *, #11875, .F. ) ;
#15983=ORIENTED_EDGE ( 'NONE', *, *, #18329, .F. ) ;
#15985=EDGE_CURVE ( 'NONE', #46519, #33480, #12082, .T. ) ;
#15987=LINE ( 'NONE', #8861, #25221 ) ;
#15988=ORIENTED_EDGE ( 'NONE', *, *, #33037, .T. ) ;
#15989=EDGE_CURVE ( 'NONE', #29431, #41564, #21943, .T. ) ;
#15992=AXIS2_PLACEMENT_3D ( 'NONE', #34078, #2011, #9913 ) ;
#15997=LINE ( 'NONE', #15749, #6227 ) ;
#16005=ORIENTED_EDGE ( 'NONE', *, *, #14398, .F. ) ;
#16006=ORIENTED_EDGE ( 'NONE', *, *, #22337, .T. ) ;
#16007=ADVANCED_FACE ( 'NONE', ( #27160 ), #16128, .F. ) ;
#16011=EDGE_LOOP ( 'NONE', ( #41207, #50333, #13476, #31775 ) ) ;
#16014=EDGE_LOOP ( 'NONE', ( #21462, #47819, #11915, #40011 ) ) ;
#16016=CARTESIAN_POINT ( 'NONE',  ( -339.1964088526558498, -116.8846903019852164, -58.63009191191289915 ) ) ;
#16023=LINE ( 'NONE', #27313, #47364 ) ;
#16024=FACE_OUTER_BOUND ( 'NONE', #30012, .T. ) ;
#16026=DIRECTION ( 'NONE',  ( 0.000000000000000000, 0.9350162426854181641, 0.3546048870425267951 ) ) ;
#16029=ADVANCED_FACE ( 'NONE', ( #19541 ), #15357, .F. ) ;
#16031=DIRECTION ( 'NONE',  ( -0.000000000000000000, -0.1205366802553268363, -0.9927088740980534176 ) ) ;
#16035=DIRECTION ( 'NONE',  ( 0.000000000000000000, 0.000000000000000000, 1.000000000000000000 ) ) ;
#16038=VERTEX_POINT ( 'NONE', #39751 ) ;
#16047=ADVANCED_FACE ( 'NONE', ( #47161, #39507 ), #43196, .F. ) ;
#16053=AXIS2_PLACEMENT_3D ( 'NONE', #10862, #6920, #26107 ) ;
#16054=EDGE_LOOP ( 'NONE', ( #39383, #40702, #19248, #46009 ) ) ;
#16057=CARTESIAN_POINT ( 'NONE',  ( -336.3521761649654422, -178.0871407151310279, 22.44790492310219676 ) ) ;
#16059=ORIENTED_EDGE ( 'NONE', *, *, #5927, .F. ) ;
#16061=CARTESIAN_POINT ( 'NONE',  ( -339.1964088526558498, -66.33409060400673241, -14.60509510167901404 ) ) ;
#16070=ORIENTED_EDGE ( 'NONE', *, *, #40606, .F. ) ;
#16074=CARTESIAN_POINT ( 'NONE',  ( -339.1964088526558498, -180.6659093959932250, 14.60509510167942437 ) ) ;
#16077=EDGE_CURVE ( 'NONE', #15270, #11472, #24269, .T. ) ;
#16079=DIRECTION ( 'NONE',  ( -0.000000000000000000, 0.000000000000000000, 1.000000000000000000 ) ) ;
#16080=VERTEX_POINT ( 'NONE', #4043 ) ;
#16087=VECTOR ( 'NONE', #15446, 1000.000000000000000 ) ;
#16088=DIRECTION ( 'NONE',  ( 0.000000000000000000, 0.1205366802553130001, -0.9927088740980551940 ) ) ;
#16096=CARTESIAN_POINT ( 'NONE',  ( -330.4913330509368166, -122.9999999999994600, 59.00000000000002132 ) ) ;
#16099=CIRCLE ( 'NONE', #30339, 60.00000000000000000 ) ;
#16100=PLANE ( 'NONE',  #26291 ) ;
#16105=ORIENTED_EDGE ( 'NONE', *, *, #40394, .T. ) ;
#16106=ORIENTED_EDGE ( 'NONE', *, *, #24142, .T. ) ;
#16109=DIRECTION ( 'NONE',  ( -0.000000000000000000, 0.2393156642875685636, 0.9709418174260492362 ) ) ;
#16112=ORIENTED_EDGE ( 'NONE', *, *, #14285, .T. ) ;
#16113=ORIENTED_EDGE ( 'NONE', *, *, #11829, .F. ) ;
#16115=PLANE ( 'NONE',  #43460 ) ;
#16120=ORIENTED_EDGE ( 'NONE', *, *, #17371, .F. ) ;
#16124=CARTESIAN_POINT ( 'NONE',  ( -336.3521761649654422, -104.1045282520827300, -55.74477592174792306 ) ) ;
#16128=PLANE ( 'NONE',  #39849 ) ;
#16131=DIRECTION ( 'NONE',  ( -0.000000000000000000, 0.9709418174260519008, -0.2393156642875582940 ) ) ;
#16135=EDGE_CURVE ( 'NONE', #7602, #37376, #9279, .T. ) ;
#16141=DIRECTION ( 'NONE',  ( -1.000000000000000000, -9.241633304753541364E-15, 4.850383327711987764E-15 ) ) ;
#16143=ORIENTED_EDGE ( 'NONE', *, *, #35795, .F. ) ;
#16147=VERTEX_POINT ( 'NONE', #16660 ) ;
#16150=CARTESIAN_POINT ( 'NONE',  ( -332.3517673607765914, -120.8677111499054320, 59.00000000000000000 ) ) ;
#16151=ORIENTED_EDGE ( 'NONE', *, *, #368, .T. ) ;
#16153=DIRECTION ( 'NONE',  ( -1.000000000000000000, 0.000000000000000000, 0.000000000000000000 ) ) ;
#16158=PLANE ( 'NONE',  #45723 ) ;
#16159=DIRECTION ( 'NONE',  ( 0.000000000000000000, 0.000000000000000000, 1.000000000000000000 ) ) ;
#16163=DIRECTION ( 'NONE',  ( 0.000000000000000000, 0.1205366802553164696, -0.9927088740980548609 ) ) ;
#16166=DIRECTION ( 'NONE',  ( -0.000000000000000000, 0.4647231720437664526, -0.8854560256532110207 ) ) ;
#16173=LINE ( 'NONE', #32189, #40241 ) ;
#16174=ADVANCED_FACE ( 'NONE', ( #24515 ), #44499, .T. ) ;
#16175=AXIS2_PLACEMENT_3D ( 'NONE', #10861, #41887, #9834 ) ;
#16177=CARTESIAN_POINT ( 'NONE',  ( -339.1964088526558498, -182.5000000000000568, 0.5000000000000457412 ) ) ;
#16183=DIRECTION ( 'NONE',  ( 0.000000000000000000, 0.5680647467311569221, 0.8229838658936556861 ) ) ;
#16184=PLANE ( 'NONE',  #20697 ) ;
#16185=ORIENTED_EDGE ( 'NONE', *, *, #40859, .T. ) ;
#16187=VERTEX_POINT ( 'NONE', #20577 ) ;
#16191=DIRECTION ( 'NONE',  ( -1.000000000000000000, 0.000000000000000000, 0.000000000000000000 ) ) ;
#16192=FACE_BOUND ( 'NONE', #4163, .T. ) ;
#16195=ORIENTED_EDGE ( 'NONE', *, *, #46202, .F. ) ;
#16196=VECTOR ( 'NONE', #37571, 1000.000000000000000 ) ;
#16198=FACE_OUTER_BOUND ( 'NONE', #46233, .T. ) ;
#16202=CARTESIAN_POINT ( 'NONE',  ( -339.1964088526558498, -66.09477493971917283, -13.63415328425296202 ) ) ;
#16204=CARTESIAN_POINT ( 'NONE',  ( -305.0000000000000568, -125.1322888500942554, -59.97779283292990016 ) ) ;
#16205=ORIENTED_EDGE ( 'NONE', *, *, #240, .F. ) ;
#16206=DIRECTION ( 'NONE',  ( -0.000000000000000000, 1.047444401652940007E-14, 1.000000000000000000 ) ) ;
#16214=LINE ( 'NONE', #8832, #33245 ) ;
#16215=LINE ( 'NONE', #51704, #37372 ) ;
#16222=DIRECTION ( 'NONE',  ( -1.000000000000000000, -0.000000000000000000, -0.000000000000000000 ) ) ;
#16225=ORIENTED_EDGE ( 'NONE', *, *, #43260, .T. ) ;
#16234=AXIS2_PLACEMENT_3D ( 'NONE', #17426, #847, #30008 ) ;
#16238=CARTESIAN_POINT ( 'NONE',  ( -336.3521761649654422, -160.6539403396202772, 45.90766452162722544 ) ) ;
#16242=ORIENTED_EDGE ( 'NONE', *, *, #14421, .T. ) ;
#16243=ORIENTED_EDGE ( 'NONE', *, *, #47155, .T. ) ;
#16251=CARTESIAN_POINT ( 'NONE',  ( -339.1964088526558498, -89.57268800991437274, 48.27201571435973904 ) ) ;
#16253=LINE ( 'NONE', #4423, #24165 ) ;
#16255=ORIENTED_EDGE ( 'NONE', *, *, #7857, .T. ) ;
#16256=CARTESIAN_POINT ( 'NONE',  ( -339.1964088526558498, -172.3400804610910200, 33.10432812419180948 ) ) ;
#16257=VERTEX_POINT ( 'NONE', #49228 ) ;
#16259=AXIS2_PLACEMENT_3D ( 'NONE', #16815, #37023, #8907 ) ;
#16260=ORIENTED_EDGE ( 'NONE', *, *, #37951, .T. ) ;
#16274=EDGE_CURVE ( 'NONE', #11192, #8568, #30623, .T. ) ;
#16276=EDGE_CURVE ( 'NONE', #21483, #30086, #5344, .T. ) ;
#16282=ORIENTED_EDGE ( 'NONE', *, *, #18717, .F. ) ;
#16284=EDGE_CURVE ( 'NONE', #24073, #9161, #2672, .T. ) ;
#16287=ORIENTED_EDGE ( 'NONE', *, *, #40464, .F. ) ;
#16288=ORIENTED_EDGE ( 'NONE', *, *, #12180, .T. ) ;
#16291=EDGE_CURVE ( 'NONE', #3877, #21100, #38147, .T. ) ;
#16294=CARTESIAN_POINT ( 'NONE',  ( -330.4913330509368166, -167.3305728129743102, 39.49849221029282376 ) ) ;
#16299=ORIENTED_EDGE ( 'NONE', *, *, #21789, .F. ) ;
#16301=CARTESIAN_POINT ( 'NONE',  ( -336.3521761649654422, -64.73342574900661361, 5.491276508483657892 ) ) ;
#16302=VERTEX_POINT ( 'NONE', #34727 ) ;
#16312=CARTESIAN_POINT ( 'NONE',  ( -305.0000000000000568, -87.28260048324004572, 47.83617848703421771 ) ) ;
#16316=VERTEX_POINT ( 'NONE', #22400 ) ;
#16317=CARTESIAN_POINT ( 'NONE',  ( -332.3517673607765914, -101.0520950768976149, 54.58714071513087873 ) ) ;
#16318=ORIENTED_EDGE ( 'NONE', *, *, #7688, .T. ) ;
#16320=DIRECTION ( 'NONE',  ( 0.000000000000000000, -0.2393156642875448881, 0.9709418174260553425 ) ) ;
#16323=VERTEX_POINT ( 'NONE', #18204 ) ;
#16325=LINE ( 'NONE', #12632, #30748 ) ;
#16330=LINE ( 'NONE', #28661, #49214 ) ;
#16332=CARTESIAN_POINT ( 'NONE',  ( -332.3517673607765914, -182.5000000000000568, 2.632288850093980503 ) ) ;
#16340=DIRECTION ( 'NONE',  ( 1.000000000000000000, -4.952603889764075929E-17, -7.175085443855059889E-17 ) ) ;
#16351=CARTESIAN_POINT ( 'NONE',  ( -332.3517673607765914, -66.60506506233235768, -15.70448169564047092 ) ) ;
#16352=EDGE_CURVE ( 'NONE', #29838, #38530, #46578, .T. ) ;
#16355=LINE ( 'NONE', #29217, #3628 ) ;
#16364=EDGE_CURVE ( 'NONE', #3547, #44417, #15529, .T. ) ;
#16365=LINE ( 'NONE', #51587, #46437 ) ;
#16366=EDGE_LOOP ( 'NONE', ( #17521, #51341, #38510, #35389 ) ) ;
#16367=ORIENTED_EDGE ( 'NONE', *, *, #36926, .F. ) ;
#16368=CIRCLE ( 'NONE', #5465, 60.00000000000000000 ) ;
#16370=DIRECTION ( 'NONE',  ( -0.000000000000000000, -0.3546048870425396182, -0.9350162426854132791 ) ) ;
#16371=CIRCLE ( 'NONE', #44924, 14.36509618646847386 ) ;
#16372=AXIS2_PLACEMENT_3D ( 'NONE', #19633, #19378, #51451 ) ;
#16375=ORIENTED_EDGE ( 'NONE', *, *, #7084, .T. ) ;
#16377=EDGE_CURVE ( 'NONE', #32161, #33399, #47093, .T. ) ;
#16394=LINE ( 'NONE', #43979, #35811 ) ;
#16396=ORIENTED_EDGE ( 'NONE', *, *, #38803, .F. ) ;
#16406=ORIENTED_EDGE ( 'NONE', *, *, #44992, .F. ) ;
#16407=FACE_OUTER_BOUND ( 'NONE', #15164, .T. ) ;
#16408=DIRECTION ( 'NONE',  ( 0.000000000000000000, -0.6631226582407885317, 0.7485107481711069655 ) ) ;
#16409=EDGE_CURVE ( 'NONE', #12138, #41880, #15818, .T. ) ;
#16411=ORIENTED_EDGE ( 'NONE', *, *, #40430, .F. ) ;
#16418=VECTOR ( 'NONE', #16141, 1000.000000000000000 ) ;
#16422=DIRECTION ( 'NONE',  ( 0.000000000000000000, -0.6631226582407937498, 0.7485107481711024136 ) ) ;
#16423=LINE ( 'NONE', #4860, #4782 ) ;
#16424=EDGE_LOOP ( 'NONE', ( #6480, #50075, #50965, #23498 ) ) ;
#16425=CARTESIAN_POINT ( 'NONE',  ( -336.3521761649654422, -174.5186198893880771, 29.74944317415823392 ) ) ;
#16430=DIRECTION ( 'NONE',  ( 1.000000000000000000, -0.000000000000000000, 0.000000000000000000 ) ) ;
#16432=VERTEX_POINT ( 'NONE', #31302 ) ;
#16433=CIRCLE ( 'NONE', #36553, 60.00000000000000000 ) ;
#16437=ADVANCED_FACE ( 'NONE', ( #31831 ), #15544, .F. ) ;
#16438=AXIS2_PLACEMENT_3D ( 'NONE', #20065, #8239, #32405 ) ;
#16440=VERTEX_POINT ( 'NONE', #11068 ) ;
#16441=DIRECTION ( 'NONE',  ( 0.000000000000000000, 0.000000000000000000, -1.000000000000000000 ) ) ;
#16445=CARTESIAN_POINT ( 'NONE',  ( -339.1964088526558498, -175.9742670995615015, -26.97593913775538965 ) ) ;
#16449=VERTEX_POINT ( 'NONE', #27359 ) ;
#16451=CARTESIAN_POINT ( 'NONE',  ( -336.3521761649654422, -125.1322888500942270, -59.00000000000002132 ) ) ;
#16452=AXIS2_PLACEMENT_3D ( 'NONE', #24952, #40964, #17077 ) ;
#16455=FACE_BOUND ( 'NONE', #28987, .T. ) ;
#16456=DIRECTION ( 'NONE',  ( 0.000000000000000000, 0.4647231720437664526, -0.8854560256532110207 ) ) ;
#16457=ORIENTED_EDGE ( 'NONE', *, *, #35318, .F. ) ;
#16459=DIRECTION ( 'NONE',  ( 1.043714542225393381E-14, -0.4647231720437631775, 0.8854560256532126861 ) ) ;
#16463=AXIS2_PLACEMENT_3D ( 'NONE', #13289, #1463, #29311 ) ;
#16470=DIRECTION ( 'NONE',  ( 0.000000000000000000, 0.000000000000000000, 1.000000000000000000 ) ) ;
#16475=DIRECTION ( 'NONE',  ( -0.000000000000000000, 0.4647231720437695057, 0.8854560256532093554 ) ) ;
#16476=CARTESIAN_POINT ( 'NONE',  ( -336.3521761649654422, -123.5000000000000284, 0.000000000000000000 ) ) ;
#16478=CARTESIAN_POINT ( 'NONE',  ( -332.3517673607765914, -154.8494888031386836, 50.05135858667791382 ) ) ;
#16487=VECTOR ( 'NONE', #26418, 1000.000000000000000 ) ;
#16490=CARTESIAN_POINT ( 'NONE',  ( -339.1964088526558498, -157.4273119900845757, 48.27201571436049932 ) ) ;
#16492=CARTESIAN_POINT ( 'NONE',  ( -339.1964088526558498, -176.3931552210903249, -28.32515014536811293 ) ) ;
#16494=CARTESIAN_POINT ( 'NONE',  ( -330.4913330509368166, -171.7720157143599238, 33.92731199008539278 ) ) ;
#16500=VERTEX_POINT ( 'NONE', #7413 ) ;
#16505=AXIS2_PLACEMENT_3D ( 'NONE', #22243, #30635, #46690 ) ;
#16506=CARTESIAN_POINT ( 'NONE',  ( -339.1964088526558498, -156.6043281241916816, -48.84008046109114076 ) ) ;
#16511=ADVANCED_FACE ( 'NONE', ( #27626 ), #24209, .F. ) ;
#16512=ORIENTED_EDGE ( 'NONE', *, *, #12861, .T. ) ;
#16518=CARTESIAN_POINT ( 'NONE',  ( -336.3521761649654422, -119.0014323656137947, -58.88711093124865670 ) ) ;
#16529=DIRECTION ( 'NONE',  ( 0.000000000000000000, 0.000000000000000000, -1.000000000000000000 ) ) ;
#16530=VERTEX_POINT ( 'NONE', #12621 ) ;
#16537=CARTESIAN_POINT ( 'NONE',  ( -339.1964088526558498, -123.5000000000000284, 0.000000000000000000 ) ) ;
#16539=ADVANCED_FACE ( 'NONE', ( #29180 ), #21300, .F. ) ;
#16544=CARTESIAN_POINT ( 'NONE',  ( -330.4913330509368166, -182.1300919119129560, -6.615309698014691264 ) ) ;
#16554=VECTOR ( 'NONE', #39741, 1000.000000000000000 ) ;
#16555=LINE ( 'NONE', #51779, #28810 ) ;
#16557=CIRCLE ( 'NONE', #23267, 15.24495751795539000 ) ;
#16559=VERTEX_POINT ( 'NONE', #20254 ) ;
#16560=ORIENTED_EDGE ( 'NONE', *, *, #33253, .T. ) ;
#16561=DIRECTION ( 'NONE',  ( 0.000000000000000000, 0.1205366802553199251, -0.9927088740980544168 ) ) ;
#16563=CARTESIAN_POINT ( 'NONE',  ( -330.4913330509368166, -84.00150778970706256, 43.83057281297416097 ) ) ;
#16565=ORIENTED_EDGE ( 'NONE', *, *, #36879, .T. ) ;
#16568=AXIS2_PLACEMENT_3D ( 'NONE', #29570, #17761, #46143 ) ;
#16569=DIRECTION ( 'NONE',  ( 0.000000000000000000, 0.9927088740980548609, 0.1205366802553164696 ) ) ;
#16570=AXIS2_PLACEMENT_3D ( 'NONE', #20283, #308, #44729 ) ;
#16573=AXIS2_PLACEMENT_3D ( 'NONE', #45995, #38072, #17857 ) ;
#16574=ORIENTED_EDGE ( 'NONE', *, *, #24704, .F. ) ;
#16576=CARTESIAN_POINT ( 'NONE',  ( -330.4913330509368166, -71.49045607248250178, -27.86139516340898581 ) ) ;
#16577=DIRECTION ( 'NONE',  ( 0.000000000000000000, -7.632783294297951215E-14, 1.000000000000000000 ) ) ;
#16580=AXIS2_PLACEMENT_3D ( 'NONE', #33700, #25819, #41851 ) ;
#16581=EDGE_LOOP ( 'NONE', ( #24177, #42783, #17528, #43843 ) ) ;
#16586=AXIS2_PLACEMENT_3D ( 'NONE', #39903, #7860, #228 ) ;
#16588=FACE_OUTER_BOUND ( 'NONE', #12349, .T. ) ;
#16591=CARTESIAN_POINT ( 'NONE',  ( -339.1964088526558498, -167.9936954712156592, -38.74998146212110584 ) ) ;
#16595=PLANE ( 'NONE',  #48229 ) ;
#16596=PLANE ( 'NONE',  #43418 ) ;
#16597=VERTEX_POINT ( 'NONE', #28391 ) ;
#16598=CARTESIAN_POINT ( 'NONE',  ( -336.3521761649654422, -177.7325358280884586, 23.38292116578760726 ) ) ;
#16603=EDGE_LOOP ( 'NONE', ( #16255, #33891, #46527, #12080 ) ) ;
#16604=ADVANCED_FACE ( 'NONE', ( #8957 ), #17381, .F. ) ;
#16617=ORIENTED_EDGE ( 'NONE', *, *, #2401, .T. ) ;
#16619=DIRECTION ( 'NONE',  ( 1.000000000000000000, 0.000000000000000000, 0.000000000000000000 ) ) ;
#16621=CARTESIAN_POINT ( 'NONE',  ( -332.3517673607765914, -145.9479049231020440, -54.58714071513102795 ) ) ;
#16628=DIRECTION ( 'NONE',  ( 0.000000000000000000, -0.2393156642875652051, -0.9709418174260502354 ) ) ;
#16640=VERTEX_POINT ( 'NONE', #1055 ) ;
#16641=ORIENTED_EDGE ( 'NONE', *, *, #402, .F. ) ;
#16642=EDGE_CURVE ( 'NONE', #1163, #23236, #25609, .T. ) ;
#16646=ADVANCED_FACE ( 'NONE', ( #48653 ), #44174, .F. ) ;
#16647=EDGE_CURVE ( 'NONE', #48164, #11058, #29959, .T. ) ;
#16654=CARTESIAN_POINT ( 'NONE',  ( -332.3517673607765914, -165.9166037625627439, 41.09453333279358134 ) ) ;
#16660=CARTESIAN_POINT ( 'NONE',  ( -330.4913330509368166, -65.12585595286510909, 13.87297036558300078 ) ) ;
#16661=ORIENTED_EDGE ( 'NONE', *, *, #21040, .T. ) ;
#16662=CARTESIAN_POINT ( 'NONE',  ( -330.4913330509368166, -157.4273119900852578, -48.27201571436002325 ) ) ;
#16663=VERTEX_POINT ( 'NONE', #18136 ) ;
#16665=EDGE_CURVE ( 'NONE', #23203, #44669, #17634, .T. ) ;
#16668=ADVANCED_FACE ( 'NONE', ( #22601 ), #14459, .F. ) ;
#16671=ORIENTED_EDGE ( 'NONE', *, *, #8520, .T. ) ;
#16677=EDGE_CURVE ( 'NONE', #7946, #809, #25498, .T. ) ;
#16680=FACE_OUTER_BOUND ( 'NONE', #49607, .T. ) ;
#16681=EDGE_CURVE ( 'NONE', #41662, #4093, #34162, .T. ) ;
#16682=CARTESIAN_POINT ( 'NONE',  ( -332.3517673607765914, -106.8245764869328980, 56.65561927337994064 ) ) ;
#16683=ORIENTED_EDGE ( 'NONE', *, *, #4429, .T. ) ;
#16686=CIRCLE ( 'NONE', #23386, 5.000000000000001776 ) ;
#16694=CARTESIAN_POINT ( 'NONE',  ( -339.1964088526558498, -183.0001959263614424, -7.728304129924259414 ) ) ;
#16696=ORIENTED_EDGE ( 'NONE', *, *, #51726, .F. ) ;
#16699=EDGE_LOOP ( 'NONE', ( #6440, #11737, #24637, #1521 ) ) ;
#16700=AXIS2_PLACEMENT_3D ( 'NONE', #42752, #43251, #7005 ) ;
#16701=DIRECTION ( 'NONE',  ( 1.000000000000000000, -0.000000000000000000, -0.000000000000000000 ) ) ;
#16704=VERTEX_POINT ( 'NONE', #50210 ) ;
#16706=VECTOR ( 'NONE', #25958, 1000.000000000000000 ) ;
#16707=ADVANCED_FACE ( 'NONE', ( #21828 ), #46013, .F. ) ;
#16709=ORIENTED_EDGE ( 'NONE', *, *, #2023, .T. ) ;
#16716=CARTESIAN_POINT ( 'NONE',  ( -336.3521761649654422, -135.0638248728647852, 57.91551518289418254 ) ) ;
#16719=ORIENTED_EDGE ( 'NONE', *, *, #10367, .F. ) ;
#16722=EDGE_CURVE ( 'NONE', #33480, #13761, #2615, .T. ) ;
#16724=FACE_OUTER_BOUND ( 'NONE', #23995, .T. ) ;
#16727=DIRECTION ( 'NONE',  ( 1.000000000000000000, -0.000000000000000000, -0.000000000000000000 ) ) ;
#16729=EDGE_LOOP ( 'NONE', ( #17580, #25340, #45988, #25585 ) ) ;
#16731=ORIENTED_EDGE ( 'NONE', *, *, #15427, .F. ) ;
#16732=DIRECTION ( 'NONE',  ( 0.000000000000000000, -0.6631226582408039638, -0.7485107481710934207 ) ) ;
#16734=CIRCLE ( 'NONE', #11682, 60.00000000000000000 ) ;
#16736=ORIENTED_EDGE ( 'NONE', *, *, #44978, .F. ) ;
#16737=EDGE_CURVE ( 'NONE', #32906, #50838, #35700, .T. ) ;
#16741=FACE_OUTER_BOUND ( 'NONE', #15373, .T. ) ;
#16745=ORIENTED_EDGE ( 'NONE', *, *, #6680, .T. ) ;
#16747=VECTOR ( 'NONE', #44986, 1000.000000000000000 ) ;
#16749=CARTESIAN_POINT ( 'NONE',  ( -332.3517673607765914, -123.5000000000000284, 0.000000000000000000 ) ) ;
#16756=ORIENTED_EDGE ( 'NONE', *, *, #6695, .F. ) ;
#16761=ORIENTED_EDGE ( 'NONE', *, *, #27407, .T. ) ;
#16762=VECTOR ( 'NONE', #48505, 1000.000000000000000 ) ;
#16763=LINE ( 'NONE', #16490, #41572 ) ;
#16765=CIRCLE ( 'NONE', #29309, 60.00000000000000000 ) ;
#16769=VERTEX_POINT ( 'NONE', #19941 ) ;
#16770=CARTESIAN_POINT ( 'NONE',  ( -332.3517673607765914, -78.25545813661345562, 37.90245108779119931 ) ) ;
#16772=LINE ( 'NONE', #12548, #20398 ) ;
#16779=ORIENTED_EDGE ( 'NONE', *, *, #31143, .F. ) ;
#16780=DIRECTION ( 'NONE',  ( -1.000000000000000000, -0.000000000000000000, -0.000000000000000000 ) ) ;
#16782=ORIENTED_EDGE ( 'NONE', *, *, #38165, .T. ) ;
#16785=DIRECTION ( 'NONE',  ( 0.000000000000000000, 0.000000000000000000, 1.000000000000000000 ) ) ;
#16786=CARTESIAN_POINT ( 'NONE',  ( -332.3517673607765914, -126.1322888500942270, -59.00000000000001421 ) ) ;
#16789=DIRECTION ( 'NONE',  ( -1.000000000000000000, 0.000000000000000000, 0.000000000000000000 ) ) ;
#16795=CARTESIAN_POINT ( 'NONE',  ( -339.1964088526558498, -171.7720157143604069, -33.92731199008472487 ) ) ;
#16797=DIRECTION ( 'NONE',  ( 0.000000000000000000, 0.000000000000000000, -1.000000000000000000 ) ) ;
#16801=ORIENTED_EDGE ( 'NONE', *, *, #28544, .T. ) ;
#16806=ORIENTED_EDGE ( 'NONE', *, *, #9758, .T. ) ;
#16807=CARTESIAN_POINT ( 'NONE',  ( -339.1964088526558498, -175.5095439275173135, 27.86139516340941213 ) ) ;
#16808=CARTESIAN_POINT ( 'NONE',  ( -336.3521761649654422, -63.67752800890095699, 4.612141029301496609 ) ) ;
#16809=CARTESIAN_POINT ( 'NONE',  ( -339.1964088526558498, -123.5000000000000284, 0.000000000000000000 ) ) ;
#16815=CARTESIAN_POINT ( 'NONE',  ( -339.1964088526558498, -138.1050951016792681, -57.16590939599323917 ) ) ;
#16821=VERTEX_POINT ( 'NONE', #47810 ) ;
#16830=AXIS2_PLACEMENT_3D ( 'NONE', #31479, #6807, #35168 ) ;
#16835=DIRECTION ( 'NONE',  ( 1.000000000000000000, 0.000000000000000000, 0.000000000000000000 ) ) ;
#16837=DIRECTION ( 'NONE',  ( -0.000000000000000000, -0.8854560256532126861, -0.4647231720437631775 ) ) ;
#16845=AXIS2_PLACEMENT_3D ( 'NONE', #28156, #44204, #8204 ) ;
#16847=DIRECTION ( 'NONE',  ( -1.000000000000000000, 0.000000000000000000, 0.000000000000000000 ) ) ;
#16849=CARTESIAN_POINT ( 'NONE',  ( -339.1964088526558498, -156.6043281241909426, 48.84008046109164525 ) ) ;
#16851=EDGE_CURVE ( 'NONE', #19412, #30801, #6823, .T. ) ;
#16855=CARTESIAN_POINT ( 'NONE',  ( -336.3521761649654422, -97.97423230103774472, -54.29949524055093946 ) ) ;
#16863=LINE ( 'NONE', #17394, #50858 ) ;
#16867=CARTESIAN_POINT ( 'NONE',  ( -330.4913330509368166, -123.5000000000000284, 0.000000000000000000 ) ) ;
#16868=DIRECTION ( 'NONE',  ( -1.000000000000000000, 0.000000000000000000, -0.000000000000000000 ) ) ;
#16869=ORIENTED_EDGE ( 'NONE', *, *, #49046, .F. ) ;
#16871=CARTESIAN_POINT ( 'NONE',  ( -339.1964088526558498, -116.8846903019842927, 58.63009191191280678 ) ) ;
#16872=ORIENTED_EDGE ( 'NONE', *, *, #15046, .T. ) ;
#16875=VECTOR ( 'NONE', #46541, 1000.000000000000000 ) ;
#16879=CARTESIAN_POINT ( 'NONE',  ( -336.3521761649654422, -180.3949349376675855, 15.70448169564087770 ) ) ;
#16885=DIRECTION ( 'NONE',  ( -1.000000000000000000, 1.013386094502320512E-14, -2.497772389992655628E-15 ) ) ;
#16892=EDGE_LOOP ( 'NONE', ( #50807, #43140, #3143, #44430 ) ) ;
#16896=VERTEX_POINT ( 'NONE', #23373 ) ;
#16900=ORIENTED_EDGE ( 'NONE', *, *, #10816, .F. ) ;
#16901=ORIENTED_EDGE ( 'NONE', *, *, #51658, .T. ) ;
#16904=VERTEX_POINT ( 'NONE', #11261 ) ;
#16908=VECTOR ( 'NONE', #46413, 1000.000000000000000 ) ;
#16916=CARTESIAN_POINT ( 'NONE',  ( -339.1964088526558498, -89.57268800991437274, 48.27201571435973904 ) ) ;
#16917=CARTESIAN_POINT ( 'NONE',  ( -332.3517673607765914, -148.5878911270064009, 53.46519113769075204 ) ) ;
#16918=ORIENTED_EDGE ( 'NONE', *, *, #31283, .T. ) ;
#16922=FACE_BOUND ( 'NONE', #5121, .T. ) ;
#16927=ORIENTED_EDGE ( 'NONE', *, *, #43261, .T. ) ;
#16940=ORIENTED_EDGE ( 'NONE', *, *, #46503, .T. ) ;
#16942=ORIENTED_EDGE ( 'NONE', *, *, #25036, .F. ) ;
#16950=CARTESIAN_POINT ( 'NONE',  ( -336.3521761649654422, -67.75522407825191351, 19.39547174791671935 ) ) ;
#16964=DIRECTION ( 'NONE',  ( 1.043714542225393539E-14, -0.8854560256532079121, 0.4647231720437725033 ) ) ;
#16966=VERTEX_POINT ( 'NONE', #12569 ) ;
#16967=VECTOR ( 'NONE', #7177, 1000.000000000000000 ) ;
#16971=CARTESIAN_POINT ( 'NONE',  ( -339.1964088526558498, -157.4273119900853146, -48.27201571435997352 ) ) ;
#16972=AXIS2_PLACEMENT_3D ( 'NONE', #13111, #40685, #9183 ) ;
#16975=FACE_BOUND ( 'NONE', #22913, .T. ) ;
#16978=EDGE_CURVE ( 'NONE', #11613, #2690, #36217, .T. ) ;
#16981=VERTEX_POINT ( 'NONE', #16256 ) ;
#16987=DIRECTION ( 'NONE',  ( 0.000000000000000000, 0.000000000000000000, 1.000000000000000000 ) ) ;
#16995=CARTESIAN_POINT ( 'NONE',  ( -336.3521761649654422, -68.91285928486892942, -22.44790492310182017 ) ) ;
#16996=EDGE_CURVE ( 'NONE', #13092, #41341, #40164, .T. ) ;
#16999=ADVANCED_FACE ( 'NONE', ( #41196 ), #4689, .F. ) ;
#17002=EDGE_CURVE ( 'NONE', #34569, #5750, #48319, .T. ) ;
#17003=ORIENTED_EDGE ( 'NONE', *, *, #50643, .F. ) ;
#17004=CARTESIAN_POINT ( 'NONE',  ( -336.3521761649653854, -64.87442053112221174, 12.76876783163883111 ) ) ;
#17010=ORIENTED_EDGE ( 'NONE', *, *, #44359, .F. ) ;
#17013=EDGE_CURVE ( 'NONE', #18653, #39568, #32801, .T. ) ;
#17018=DIRECTION ( 'NONE',  ( -1.000000000000000000, 0.000000000000000000, 0.000000000000000000 ) ) ;
#17019=ADVANCED_FACE ( 'NONE', ( #31122 ), #6709, .F. ) ;
#17020=ORIENTED_EDGE ( 'NONE', *, *, #39545, .F. ) ;
#17026=VERTEX_POINT ( 'NONE', #38501 ) ;
#17032=EDGE_CURVE ( 'NONE', #6808, #48562, #30702, .T. ) ;
#17033=CIRCLE ( 'NONE', #48081, 60.00000000000000000 ) ;
#17035=CARTESIAN_POINT ( 'NONE',  ( -330.4913330509368166, -123.5000000000000284, 0.000000000000000000 ) ) ;
#17037=ORIENTED_EDGE ( 'NONE', *, *, #41308, .T. ) ;
#17038=LINE ( 'NONE', #36456, #46063 ) ;
#17039=FACE_OUTER_BOUND ( 'NONE', #34081, .T. ) ;
#17040=CARTESIAN_POINT ( 'NONE',  ( -339.1964088526558498, -78.92247586332028675, -40.16023333901007675 ) ) ;
#17043=ADVANCED_FACE ( 'NONE', ( #50853 ), #10639, .T. ) ;
#17048=DIRECTION ( 'NONE',  ( 0.000000000000000000, 0.1205366802553337752, 0.9927088740980526405 ) ) ;
#17049=ORIENTED_EDGE ( 'NONE', *, *, #33241, .T. ) ;
#17051=VECTOR ( 'NONE', #2196, 1000.000000000000114 ) ;
#17053=DIRECTION ( 'NONE',  ( 1.043714542225393223E-14, -0.3546048870425300148, 0.9350162426854169428 ) ) ;
#17054=ORIENTED_EDGE ( 'NONE', *, *, #42682, .F. ) ;
#17055=DIRECTION ( 'NONE',  ( 0.000000000000000000, 0.7485107481711089639, 0.6631226582407863113 ) ) ;
#17059=DIRECTION ( 'NONE',  ( 0.000000000000000000, 0.6631226582407911962, -0.7485107481711046340 ) ) ;
#17060=ORIENTED_EDGE ( 'NONE', *, *, #49362, .F. ) ;
#17064=DIRECTION ( 'NONE',  ( -0.000000000000000000, 1.000000000000000000, -0.000000000000000000 ) ) ;
#17071=ADVANCED_FACE ( 'NONE', ( #22728 ), #38736, .F. ) ;
#17072=EDGE_CURVE ( 'NONE', #36128, #29872, #34793, .T. ) ;
#17074=CARTESIAN_POINT ( 'NONE',  ( -336.3521761649654422, -169.4076645216271402, -37.15394033962039089 ) ) ;
#17076=DIRECTION ( 'NONE',  ( 0.000000000000000000, 0.9927088740980544168, 0.1205366802553199251 ) ) ;
#17077=DIRECTION ( 'NONE',  ( 0.000000000000000000, 0.000000000000000000, 1.000000000000000000 ) ) ;
#17079=FACE_OUTER_BOUND ( 'NONE', #722, .T. ) ;
#17082=DIRECTION ( 'NONE',  ( 0.000000000000000000, 0.6631226582408039638, 0.7485107481710934207 ) ) ;
#17085=VECTOR ( 'NONE', #10522, 1000.000000000000000 ) ;
#17086=ORIENTED_EDGE ( 'NONE', *, *, #49179, .T. ) ;
#17087=LINE ( 'NONE', #20232, #32638 ) ;
#17093=ORIENTED_EDGE ( 'NONE', *, *, #19711, .F. ) ;
#17094=DIRECTION ( 'NONE',  ( 1.000000000000000000, -0.000000000000000000, -0.000000000000000000 ) ) ;
#17097=ORIENTED_EDGE ( 'NONE', *, *, #8354, .T. ) ;
#17100=ORIENTED_EDGE ( 'NONE', *, *, #9979, .F. ) ;
#17107=CARTESIAN_POINT ( 'NONE',  ( -305.0000000000000568, -156.2279223070262049, 50.28800156563451651 ) ) ;
#17108=DIRECTION ( 'NONE',  ( -0.000000000000000000, -0.8854560256532126861, -0.4647231720437631775 ) ) ;
#17111=DIRECTION ( 'NONE',  ( -1.000000000000000000, -0.000000000000000000, -0.000000000000000000 ) ) ;
#17114=CARTESIAN_POINT ( 'NONE',  ( -339.1964088526558498, -95.63860483659040312, 52.00954392751717847 ) ) ;
#17115=ORIENTED_EDGE ( 'NONE', *, *, #23536, .T. ) ;
#17117=LINE ( 'NONE', #46018, #34989 ) ;
#17118=LINE ( 'NONE', #32086, #27326 ) ;
#17124=ORIENTED_EDGE ( 'NONE', *, *, #15267, .F. ) ;
#17127=DIRECTION ( 'NONE',  ( 0.000000000000000000, 0.000000000000000000, 1.000000000000000000 ) ) ;
#17128=ORIENTED_EDGE ( 'NONE', *, *, #35937, .F. ) ;
#17134=DIRECTION ( 'NONE',  ( 0.000000000000000000, 0.3546048870425331234, -0.9350162426854158326 ) ) ;
#17142=ADVANCED_FACE ( 'NONE', ( #7148 ), #47102, .F. ) ;
#17143=CARTESIAN_POINT ( 'NONE',  ( -332.3517673607765914, -98.41210887299327226, -53.46519113769058151 ) ) ;
#17145=ORIENTED_EDGE ( 'NONE', *, *, #45415, .T. ) ;
#17164=DIRECTION ( 'NONE',  ( -1.000000000000000000, 0.000000000000000000, 0.000000000000000000 ) ) ;
#17180=EDGE_LOOP ( 'NONE', ( #13403, #4495, #42494, #4739 ) ) ;
#17185=LINE ( 'NONE', #33200, #47429 ) ;
#17188=CARTESIAN_POINT ( 'NONE',  ( -336.3521761649654422, -94.63601285149479736, 51.48334306143172512 ) ) ;
#17190=ADVANCED_FACE ( 'NONE', ( #39698 ), #3712, .F. ) ;
#17191=CARTESIAN_POINT ( 'NONE',  ( 0.000000000000000000, -64.50000000000000000, 0.000000000000000000 ) ) ;
#17194=PLANE ( 'NONE',  #40785 ) ;
#17197=LINE ( 'NONE', #13254, #32455 ) ;
#17205=ORIENTED_EDGE ( 'NONE', *, *, #50057, .T. ) ;
#17209=FACE_OUTER_BOUND ( 'NONE', #11705, .T. ) ;
#17211=CARTESIAN_POINT ( 'NONE',  ( -336.3521761649654422, -132.2320517616439020, -58.37307289257706344 ) ) ;
#17213=ORIENTED_EDGE ( 'NONE', *, *, #47048, .T. ) ;
#17216=VERTEX_POINT ( 'NONE', #11080 ) ;
#17228=CARTESIAN_POINT ( 'NONE',  ( -339.1964088526558498, -123.5000000000000284, 0.000000000000000000 ) ) ;
#17233=EDGE_LOOP ( 'NONE', ( #44143, #15093, #50144, #20846 ) ) ;
#17236=ORIENTED_EDGE ( 'NONE', *, *, #13722, .F. ) ;
#17238=FACE_OUTER_BOUND ( 'NONE', #29398, .T. ) ;
#17243=CARTESIAN_POINT ( 'NONE',  ( -330.4913330509368166, -171.7720157143599238, 33.92731199008539278 ) ) ;
#17244=DIRECTION ( 'NONE',  ( 0.000000000000000000, 0.000000000000000000, -1.000000000000000000 ) ) ;
#17245=ORIENTED_EDGE ( 'NONE', *, *, #3047, .T. ) ;
#17246=EDGE_CURVE ( 'NONE', #18753, #43264, #38248, .T. ) ;
#17249=VECTOR ( 'NONE', #49063, 1000.000000000000000 ) ;
#17250=ADVANCED_FACE ( 'NONE', ( #23449 ), #47357, .T. ) ;
#17252=DIRECTION ( 'NONE',  ( 0.000000000000000000, -0.2393156642875448881, 0.9709418174260553425 ) ) ;
#17256=VERTEX_POINT ( 'NONE', #288 ) ;
#17258=EDGE_CURVE ( 'NONE', #12090, #5922, #31056, .T. ) ;
#17259=CARTESIAN_POINT ( 'NONE',  ( -330.4913330509368166, -123.5000000000000284, 0.000000000000000000 ) ) ;
#17265=LINE ( 'NONE', #33282, #32003 ) ;
#17269=CARTESIAN_POINT ( 'NONE',  ( -332.3517673607765914, -146.8829211657874794, -54.23253582808848705 ) ) ;
#17271=CARTESIAN_POINT ( 'NONE',  ( -336.3521761649654422, -163.8460225846223466, -43.07972642080364523 ) ) ;
#17278=DIRECTION ( 'NONE',  ( 0.000000000000000000, 0.000000000000000000, 1.000000000000000000 ) ) ;
#17279=EDGE_LOOP ( 'NONE', ( #16761, #46333, #25505, #45585 ) ) ;
#17291=LINE ( 'NONE', #44879, #18371 ) ;
#17295=EDGE_LOOP ( 'NONE', ( #25711, #14706, #45118, #11644 ) ) ;
#17306=CARTESIAN_POINT ( 'NONE',  ( -339.1964088526558498, -180.9052250602809977, -13.63415328425247885 ) ) ;
#17308=ORIENTED_EDGE ( 'NONE', *, *, #27009, .T. ) ;
#17311=CARTESIAN_POINT ( 'NONE',  ( -339.1964088526558498, -95.63860483659040312, 52.00954392751717847 ) ) ;
#17315=ORIENTED_EDGE ( 'NONE', *, *, #35601, .T. ) ;
#17318=EDGE_LOOP ( 'NONE', ( #18483, #4886, #39390, #1768 ) ) ;
#17322=AXIS2_PLACEMENT_3D ( 'NONE', #47259, #3607, #44347 ) ;
#17323=LINE ( 'NONE', #28859, #10468 ) ;
#17325=EDGE_CURVE ( 'NONE', #10943, #28183, #23990, .T. ) ;
#17326=DIRECTION ( 'NONE',  ( 0.000000000000000000, 0.6631226582408039638, 0.7485107481710934207 ) ) ;
#17329=AXIS2_PLACEMENT_3D ( 'NONE', #18667, #42301, #50224 ) ;
#17333=PRODUCT_CONTEXT ( 'NONE', #20613, 'mechanical' ) ;
#17334=DIRECTION ( 'NONE',  ( 0.000000000000000000, 0.6631226582407911962, -0.7485107481711046340 ) ) ;
#17335=LINE ( 'NONE', #27649, #27856 ) ;
#17338=EDGE_CURVE ( 'NONE', #35535, #46461, #21584, .T. ) ;
#17339=EDGE_CURVE ( 'NONE', #44669, #13273, #48394, .T. ) ;
#17341=VERTEX_POINT ( 'NONE', #25002 ) ;
#17342=CIRCLE ( 'NONE', #7266, 60.00000000000000000 ) ;
#17343=AXIS2_PLACEMENT_3D ( 'NONE', #45448, #38057, #38318 ) ;
#17347=ORIENTED_EDGE ( 'NONE', *, *, #7715, .T. ) ;
#17351=EDGE_CURVE ( 'NONE', #42367, #6696, #9487, .T. ) ;
#17354=LINE ( 'NONE', #32581, #9448 ) ;
#17355=DIRECTION ( 'NONE',  ( 0.000000000000000000, -0.6631226582407863113, 0.7485107481711089639 ) ) ;
#17356=DIRECTION ( 'NONE',  ( -8.718379230999705894E-17, -0.5680647467311457088, 0.8229838658936634577 ) ) ;
#17357=EDGE_LOOP ( 'NONE', ( #21075, #48007, #24141, #26059 ) ) ;
#17360=EDGE_LOOP ( 'NONE', ( #32323, #16151, #35881, #18473 ) ) ;
#17363=CARTESIAN_POINT ( 'NONE',  ( -339.1964088526558498, -89.57268800991514013, -48.27201571436026484 ) ) ;
#17364=CIRCLE ( 'NONE', #566, 60.00000000000000000 ) ;
#17369=EDGE_CURVE ( 'NONE', #33577, #7787, #32618, .T. ) ;
#17371=EDGE_CURVE ( 'NONE', #6229, #38472, #21050, .T. ) ;
#17374=DIRECTION ( 'NONE',  ( 1.000000000000000000, 0.000000000000000000, 0.000000000000000000 ) ) ;
#17381=PLANE ( 'NONE',  #12165 ) ;
#17385=ORIENTED_EDGE ( 'NONE', *, *, #40564, .F. ) ;
#17386=CARTESIAN_POINT ( 'NONE',  ( -339.1964088526558498, -180.9052250602807703, 13.63415328425337236 ) ) ;
#17394=CARTESIAN_POINT ( 'NONE',  ( -339.1964088526558498, -64.50000000000000000, -0.5000000000000457412 ) ) ;
#17395=EDGE_CURVE ( 'NONE', #18306, #43135, #16325, .T. ) ;
#17396=VERTEX_POINT ( 'NONE', #37851 ) ;
#17402=CARTESIAN_POINT ( 'NONE',  ( -339.1964088526558498, -131.1080185721133660, -58.50955523165751515 ) ) ;
#17403=CARTESIAN_POINT ( 'NONE',  ( -330.4913330509368166, -63.87926739338334414, -6.735595255826711814 ) ) ;
#17408=AXIS2_PLACEMENT_3D ( 'NONE', #27595, #40194, #36246 ) ;
#17416=AXIS2_PLACEMENT_3D ( 'NONE', #16849, #19995, #23928 ) ;
#17417=LINE ( 'NONE', #36578, #46332 ) ;
#17422=EDGE_LOOP ( 'NONE', ( #14569, #2791, #41635, #36618 ) ) ;
#17426=CARTESIAN_POINT ( 'NONE',  ( 0.000000000000000000, -79.33786585790457480, 39.12423683620640702 ) ) ;
#17431=CARTESIAN_POINT ( 'NONE',  ( -332.3517673607765914, -132.2320517616439020, -58.37307289257706344 ) ) ;
#17437=AXIS2_PLACEMENT_3D ( 'NONE', #25380, #1468, #25893 ) ;
#17438=DIRECTION ( 'NONE',  ( -1.000000000000000000, 0.000000000000000000, 0.000000000000000000 ) ) ;
#17443=PLANE ( 'NONE',  #1168 ) ;
#17451=ORIENTED_EDGE ( 'NONE', *, *, #41744, .F. ) ;
#17453=DIRECTION ( 'NONE',  ( 1.000000000000000000, -0.000000000000000000, -0.000000000000000000 ) ) ;
#17454=VECTOR ( 'NONE', #29178, 1000.000000000000000 ) ;
#17460=FACE_BOUND ( 'NONE', #50306, .T. ) ;
#17464=ORIENTED_EDGE ( 'NONE', *, *, #7048, .F. ) ;
#17468=CARTESIAN_POINT ( 'NONE',  ( -305.0000000000000568, -123.5000000000000284, 0.000000000000000000 ) ) ;
#17471=LINE ( 'NONE', #9827, #6255 ) ;
#17475=ORIENTED_EDGE ( 'NONE', *, *, #39886, .F. ) ;
#17476=CARTESIAN_POINT ( 'NONE',  ( -330.4913330509368166, -180.6659093959932250, 14.60509510167933556 ) ) ;
#17480=VECTOR ( 'NONE', #11474, 1000.000000000000000 ) ;
#17483=ORIENTED_EDGE ( 'NONE', *, *, #35617, .T. ) ;
#17488=CARTESIAN_POINT ( 'NONE',  ( -336.3521761649654422, -182.5000000000000568, 1.632288850093980725 ) ) ;
#17489=VECTOR ( 'NONE', #35172, 1000.000000000000000 ) ;
#17490=ORIENTED_EDGE ( 'NONE', *, *, #17614, .F. ) ;
#17493=DIRECTION ( 'NONE',  ( -0.000000000000000000, 0.000000000000000000, -1.000000000000000000 ) ) ;
#17494=FACE_OUTER_BOUND ( 'NONE', #23555, .T. ) ;
#17498=VERTEX_POINT ( 'NONE', #6317 ) ;
#17501=CIRCLE ( 'NONE', #46866, 60.00000000000000000 ) ;
#17503=CARTESIAN_POINT ( 'NONE',  ( -336.3521761649654422, -64.66963335249506883, 11.78931550685348029 ) ) ;
#17504=EDGE_CURVE ( 'NONE', #15290, #14977, #14720, .T. ) ;
#17507=ORIENTED_EDGE ( 'NONE', *, *, #45472, .F. ) ;
#17513=VECTOR ( 'NONE', #14084, 1000.000000000000114 ) ;
#17516=EDGE_CURVE ( 'NONE', #42461, #37884, #25774, .T. ) ;
#17517=LINE ( 'NONE', #20930, #43438 ) ;
#17519=FACE_OUTER_BOUND ( 'NONE', #38770, .T. ) ;
#17521=ORIENTED_EDGE ( 'NONE', *, *, #37833, .T. ) ;
#17523=EDGE_LOOP ( 'NONE', ( #24830, #27239, #2942, #2373 ) ) ;
#17528=ORIENTED_EDGE ( 'NONE', *, *, #18191, .F. ) ;
#17531=CARTESIAN_POINT ( 'NONE',  ( -332.3517673607765914, -72.67320051506121104, 31.88473700876054551 ) ) ;
#17534=DIRECTION ( 'NONE',  ( 0.000000000000000000, -0.9709418174260493473, 0.2393156642875685913 ) ) ;
#17540=ORIENTED_EDGE ( 'NONE', *, *, #42016, .T. ) ;
#17544=FACE_OUTER_BOUND ( 'NONE', #49870, .T. ) ;
#17547=FACE_OUTER_BOUND ( 'NONE', #28896, .T. ) ;
#17553=ORIENTED_EDGE ( 'NONE', *, *, #36834, .T. ) ;
#17556=LINE ( 'NONE', #33569, #35958 ) ;
#17559=ORIENTED_EDGE ( 'NONE', *, *, #22815, .T. ) ;
#17561=LINE ( 'NONE', #22535, #48864 ) ;
#17566=FACE_OUTER_BOUND ( 'NONE', #51633, .T. ) ;
#17569=ORIENTED_EDGE ( 'NONE', *, *, #40859, .F. ) ;
#17573=PLANE ( 'NONE',  #2932 ) ;
#17577=VERTEX_POINT ( 'NONE', #26026 ) ;
#17580=ORIENTED_EDGE ( 'NONE', *, *, #6170, .T. ) ;
#17582=DIRECTION ( 'NONE',  ( -1.000000000000000000, -0.000000000000000000, 0.000000000000000000 ) ) ;
#17584=LINE ( 'NONE', #764, #48191 ) ;
#17587=CARTESIAN_POINT ( 'NONE',  ( -332.3517673607765914, -85.59754891220836726, -45.24454186338619621 ) ) ;
#17592=ORIENTED_EDGE ( 'NONE', *, *, #17622, .F. ) ;
#17597=ADVANCED_FACE ( 'NONE', ( #11016 ), #7601, .F. ) ;
#17600=EDGE_CURVE ( 'NONE', #46515, #30632, #20659, .T. ) ;
#17601=ORIENTED_EDGE ( 'NONE', *, *, #35550, .T. ) ;
#17602=EDGE_CURVE ( 'NONE', #34082, #41945, #2881, .T. ) ;
#17610=CARTESIAN_POINT ( 'NONE',  ( -332.3517673607765914, -171.1288023355047585, 34.85916744524404720 ) ) ;
#17613=CARTESIAN_POINT ( 'NONE',  ( -339.1964088526558498, -95.17484985463089231, 52.89315522108975642 ) ) ;
#17614=EDGE_CURVE ( 'NONE', #30219, #38873, #51762, .T. ) ;
#17622=EDGE_CURVE ( 'NONE', #12850, #35564, #51498, .T. ) ;
#17628=CARTESIAN_POINT ( 'NONE',  ( -332.3517673607765914, -83.15397741537739762, 43.07972642080338233 ) ) ;
#17630=VERTEX_POINT ( 'NONE', #15776 ) ;
#17634=LINE ( 'NONE', #13672, #33186 ) ;
#17640=FACE_OUTER_BOUND ( 'NONE', #49910, .T. ) ;
#17643=ORIENTED_EDGE ( 'NONE', *, *, #966, .F. ) ;
#17645=AXIS2_PLACEMENT_3D ( 'NONE', #20100, #16430, #4085 ) ;
#17653=CARTESIAN_POINT ( 'NONE',  ( -336.3521761649654422, -123.5000000000000284, 0.000000000000000000 ) ) ;
#17654=VERTEX_POINT ( 'NONE', #27307 ) ;
#17660=AXIS2_PLACEMENT_3D ( 'NONE', #16301, #21284, #8414 ) ;
#17662=DIRECTION ( 'NONE',  ( 0.000000000000000000, 1.000000000000000000, -3.491481338843133355E-15 ) ) ;
#17669=DIRECTION ( 'NONE',  ( -1.000000000000000000, -9.758900497077134646E-15, 3.701062773504915833E-15 ) ) ;
#17671=CARTESIAN_POINT ( 'NONE',  ( 0.000000000000000000, -71.25809448646064936, -27.41866715058241866 ) ) ;
#17674=VERTEX_POINT ( 'NONE', #18051 ) ;
#17679=LINE ( 'NONE', #21873, #13715 ) ;
#17683=EDGE_CURVE ( 'NONE', #34468, #43598, #14122, .T. ) ;
#17690=EDGE_CURVE ( 'NONE', #17967, #9413, #2787, .T. ) ;
#17691=CARTESIAN_POINT ( 'NONE',  ( -332.3517673607765914, -123.5000000000000284, 0.000000000000000000 ) ) ;
#17694=AXIS2_PLACEMENT_3D ( 'NONE', #38540, #50631, #23299 ) ;
#17702=EDGE_CURVE ( 'NONE', #9413, #15564, #3049, .T. ) ;
#17707=ORIENTED_EDGE ( 'NONE', *, *, #44895, .F. ) ;
#17708=CARTESIAN_POINT ( 'NONE',  ( -336.3521761649654422, -119.0014323656137947, -58.88711093124865670 ) ) ;
#17720=ORIENTED_EDGE ( 'NONE', *, *, #10672, .T. ) ;
#17724=EDGE_CURVE ( 'NONE', #30970, #46519, #33814, .T. ) ;
#17725=CARTESIAN_POINT ( 'NONE',  ( -330.4913330509368166, -84.00150778970767362, -43.83057281297470098 ) ) ;
#17726=VERTEX_POINT ( 'NONE', #50129 ) ;
#17729=VECTOR ( 'NONE', #46689, 1000.000000000000114 ) ;
#17734=DIRECTION ( 'NONE',  ( -0.000000000000000000, -0.2393156642875582940, -0.9709418174260519008 ) ) ;
#17736=ORIENTED_EDGE ( 'NONE', *, *, #41383, .T. ) ;
#17738=EDGE_CURVE ( 'NONE', #31384, #9916, #6749, .T. ) ;
#17740=FACE_OUTER_BOUND ( 'NONE', #50184, .T. ) ;
#17741=CARTESIAN_POINT ( 'NONE',  ( -339.1964088526558498, -102.1108035431470427, 54.98865587491797413 ) ) ;
#17744=DIRECTION ( 'NONE',  ( -1.000000000000000000, 0.000000000000000000, -0.000000000000000000 ) ) ;
#17745=ORIENTED_EDGE ( 'NONE', *, *, #23709, .T. ) ;
#17751=CARTESIAN_POINT ( 'NONE',  ( -332.3517673607765914, -81.08339623743702873, -41.09453333279329712 ) ) ;
#17752=AXIS2_PLACEMENT_3D ( 'NONE', #26939, #43231, #7241 ) ;
#17753=LINE ( 'NONE', #41642, #23660 ) ;
#17754=CARTESIAN_POINT ( 'NONE',  ( 0.000000000000000000, -157.0158200571378018, 48.55604808772604741 ) ) ;
#17759=ORIENTED_EDGE ( 'NONE', *, *, #38752, .F. ) ;
#17761=DIRECTION ( 'NONE',  ( 0.000000000000000000, 0.8229838658936495799, -0.5680647467311656929 ) ) ;
#17763=FACE_OUTER_BOUND ( 'NONE', #30545, .T. ) ;
#17768=ORIENTED_EDGE ( 'NONE', *, *, #22405, .T. ) ;
#17769=LINE ( 'NONE', #42718, #44737 ) ;
#17770=CARTESIAN_POINT ( 'NONE',  ( -336.3521761649654422, -126.1322888500942270, -59.00000000000001421 ) ) ;
#17771=ORIENTED_EDGE ( 'NONE', *, *, #45564, .F. ) ;
#17778=CARTESIAN_POINT ( 'NONE',  ( -339.1964088526558498, -182.5000000000000568, -0.4999999999999543698 ) ) ;
#17781=CARTESIAN_POINT ( 'NONE',  ( -330.4913330509368166, -71.49045607248250178, -27.86139516340898581 ) ) ;
#17793=ORIENTED_EDGE ( 'NONE', *, *, #11114, .T. ) ;
#17798=ORIENTED_EDGE ( 'NONE', *, *, #8147, .T. ) ;
#17804=VECTOR ( 'NONE', #38102, 999.9999999999998863 ) ;
#17807=AXIS2_PLACEMENT_3D ( 'NONE', #7119, #19215, #27338 ) ;
#17814=ORIENTED_EDGE ( 'NONE', *, *, #17369, .T. ) ;
#17815=DIRECTION ( 'NONE',  ( -8.718379230999705894E-17, 0.3546048870425363986, 0.9350162426854146114 ) ) ;
#17817=ORIENTED_EDGE ( 'NONE', *, *, #36627, .F. ) ;
#17819=CARTESIAN_POINT ( 'NONE',  ( -336.3521761649654422, -128.9912765084839066, 58.76657425099337928 ) ) ;
#17820=DIRECTION ( 'NONE',  ( -1.000000000000000000, 0.000000000000000000, 0.000000000000000000 ) ) ;
#17821=ORIENTED_EDGE ( 'NONE', *, *, #33392, .T. ) ;
#17825=VECTOR ( 'NONE', #6772, 1000.000000000000000 ) ;
#17827=ORIENTED_EDGE ( 'NONE', *, *, #21604, .F. ) ;
#17828=PLANE ( 'NONE',  #1023 ) ;
#17829=CIRCLE ( 'NONE', #1010, 60.00000000000000000 ) ;
#17830=LINE ( 'NONE', #37788, #20557 ) ;
#17840=LINE ( 'NONE', #6009, #23162 ) ;
#17841=ADVANCED_FACE ( 'NONE', ( #26178 ), #6228, .T. ) ;
#17842=CARTESIAN_POINT ( 'NONE',  ( -365.0000000000001137, -168.5000000000000284, 0.000000000000000000 ) ) ;
#17846=CIRCLE ( 'NONE', #37975, 60.00000000000000000 ) ;
#17848=CARTESIAN_POINT ( 'NONE',  ( -336.3521761649654422, -82.40546666720629787, 42.41660376256258047 ) ) ;
#17857=DIRECTION ( 'NONE',  ( 0.000000000000000000, -0.7485107481711089639, -0.6631226582407863113 ) ) ;
#17860=EDGE_LOOP ( 'NONE', ( #29554, #44815, #48290, #8793 ) ) ;
#17862=CARTESIAN_POINT ( 'NONE',  ( -336.3521761649654422, -177.7325358280884586, 23.38292116578760726 ) ) ;
#17865=AXIS2_PLACEMENT_3D ( 'NONE', #51982, #27767, #3350 ) ;
#17868=DIRECTION ( 'NONE',  ( 0.000000000000000000, 0.000000000000000000, -1.000000000000000000 ) ) ;
#17869=ORIENTED_EDGE ( 'NONE', *, *, #5523, .F. ) ;
#17876=VERTEX_POINT ( 'NONE', #20114 ) ;
#17884=DIRECTION ( 'NONE',  ( 0.000000000000000000, 0.000000000000000000, -1.000000000000000000 ) ) ;
#17885=DIRECTION ( 'NONE',  ( 0.000000000000000000, 1.119474883163699554E-13, 1.000000000000000000 ) ) ;
#17886=CARTESIAN_POINT ( 'NONE',  ( -330.4913330509368166, -123.5000000000000284, 0.000000000000000000 ) ) ;
#17891=ORIENTED_EDGE ( 'NONE', *, *, #1695, .T. ) ;
#17895=DIRECTION ( 'NONE',  ( -0.000000000000000000, -0.8854560256532126861, -0.4647231720437631775 ) ) ;
#17897=DIRECTION ( 'NONE',  ( -0.000000000000000000, 0.6631226582407965253, 0.7485107481711000821 ) ) ;
#17898=CARTESIAN_POINT ( 'NONE',  ( -305.0000000000000568, -181.8741440471346493, 13.87297036558422647 ) ) ;
#17899=ORIENTED_EDGE ( 'NONE', *, *, #28332, .F. ) ;
#17911=LINE ( 'NONE', #37348, #20603 ) ;
#17917=FACE_OUTER_BOUND ( 'NONE', #7263, .T. ) ;
#17921=ORIENTED_EDGE ( 'NONE', *, *, #33334, .F. ) ;
#17929=EDGE_LOOP ( 'NONE', ( #5446, #51532, #24702, #32100 ) ) ;
#17934=ORIENTED_EDGE ( 'NONE', *, *, #31389, .T. ) ;
#17935=EDGE_CURVE ( 'NONE', #49256, #38482, #19095, .T. ) ;
#17939=ORIENTED_EDGE ( 'NONE', *, *, #3903, .F. ) ;
#17943=CARTESIAN_POINT ( 'NONE',  ( -336.3521761649654422, -120.8677111499054320, 59.00000000000000000 ) ) ;
#17944=EDGE_LOOP ( 'NONE', ( #22261, #21063, #35775, #9477 ) ) ;
#17947=ADVANCED_FACE ( 'NONE', ( #7771 ), #16184, .F. ) ;
#17949=LINE ( 'NONE', #14265, #8130 ) ;
#17953=ORIENTED_EDGE ( 'NONE', *, *, #617, .F. ) ;
#17954=ORIENTED_EDGE ( 'NONE', *, *, #43568, .F. ) ;
#17959=DIRECTION ( 'NONE',  ( 0.000000000000000000, 0.9927088740980544168, 0.1205366802553199251 ) ) ;
#17960=AXIS2_PLACEMENT_3D ( 'NONE', #11228, #26221, #10202 ) ;
#17965=VECTOR ( 'NONE', #51202, 1000.000000000000114 ) ;
#17967=VERTEX_POINT ( 'NONE', #24836 ) ;
#17968=LINE ( 'NONE', #41873, #5639 ) ;
#17973=ORIENTED_EDGE ( 'NONE', *, *, #36585, .T. ) ;
#17974=EDGE_CURVE ( 'NONE', #38255, #15864, #42530, .T. ) ;
#17975=PLANE ( 'NONE',  #46231 ) ;
#17976=CARTESIAN_POINT ( 'NONE',  ( -336.3521761649654422, -65.58448481710581746, 11.56382487286456140 ) ) ;
#17977=PLANE ( 'NONE',  #35788 ) ;
#17979=DIRECTION ( 'NONE',  ( 0.000000000000000000, 5.851800525628429686E-14, -1.000000000000000000 ) ) ;
#17980=EDGE_CURVE ( 'NONE', #1552, #31094, #20370, .T. ) ;
#17981=ORIENTED_EDGE ( 'NONE', *, *, #2760, .T. ) ;
#17983=EDGE_LOOP ( 'NONE', ( #24934, #31619, #31767, #33984 ) ) ;
#17986=ORIENTED_EDGE ( 'NONE', *, *, #41504, .F. ) ;
#17989=EDGE_CURVE ( 'NONE', #10439, #6696, #21414, .T. ) ;
#17990=CARTESIAN_POINT ( 'NONE',  ( -336.3521761649654422, -177.7325358280884586, 23.38292116578760726 ) ) ;
#17993=ORIENTED_EDGE ( 'NONE', *, *, #48739, .T. ) ;
#17994=LINE ( 'NONE', #42677, #20812 ) ;
#17995=CARTESIAN_POINT ( 'NONE',  ( -339.1964088526558498, -150.4759391377560576, -52.47426709956116042 ) ) ;
#17997=VECTOR ( 'NONE', #29384, 1000.000000000000000 ) ;
#18000=ORIENTED_EDGE ( 'NONE', *, *, #39806, .F. ) ;
#18003=EDGE_LOOP ( 'NONE', ( #5032, #44271, #43419, #19110 ) ) ;
#18005=DIRECTION ( 'NONE',  ( 1.043714542225393381E-14, 0.8229838658936613482, 0.5680647467311485954 ) ) ;
#18012=EDGE_CURVE ( 'NONE', #34105, #19012, #3939, .T. ) ;
#18015=PLANE ( 'NONE',  #16463 ) ;
#18018=CARTESIAN_POINT ( 'NONE',  ( -305.0000000000000568, -65.92952926200918284, -16.90091414705545247 ) ) ;
#18019=CARTESIAN_POINT ( 'NONE',  ( -332.3517673607765914, -99.78295912235451226, 55.11353710303931308 ) ) ;
#18021=CARTESIAN_POINT ( 'NONE',  ( -305.0000000000000568, -142.2945752170892035, 56.98038208374156000 ) ) ;
#18022=EDGE_LOOP ( 'NONE', ( #16940, #9396, #19459, #4816 ) ) ;
#18023=CARTESIAN_POINT ( 'NONE',  ( -332.3517673607765914, -173.5513585866778214, -31.34948880313881503 ) ) ;
#18025=ORIENTED_EDGE ( 'NONE', *, *, #44439, .T. ) ;
#18027=DIRECTION ( 'NONE',  ( -0.000000000000000000, 0.4647231720437664526, -0.8854560256532110207 ) ) ;
#18034=DIRECTION ( 'NONE',  ( 0.000000000000000000, 0.1205366802553268363, 0.9927088740980534176 ) ) ;
#18037=FACE_OUTER_BOUND ( 'NONE', #51618, .T. ) ;
#18040=FACE_OUTER_BOUND ( 'NONE', #49187, .T. ) ;
#18042=ORIENTED_EDGE ( 'NONE', *, *, #18783, .F. ) ;
#18047=DIRECTION ( 'NONE',  ( 1.000000000000000000, -0.000000000000000000, -0.000000000000000000 ) ) ;
#18049=DIRECTION ( 'NONE',  ( 0.000000000000000000, 0.000000000000000000, 1.000000000000000000 ) ) ;
#18051=CARTESIAN_POINT ( 'NONE',  ( -339.1964088526558498, -68.15673923803898049, 20.45418021416614351 ) ) ;
#18057=AXIS2_PLACEMENT_3D ( 'NONE', #42119, #45818, #1134 ) ;
#18058=LINE ( 'NONE', #30643, #40211 ) ;
#18059=AXIS2_PLACEMENT_3D ( 'NONE', #11398, #51619, #43205 ) ;
#18061=DIRECTION ( 'NONE',  ( 0.000000000000000000, -0.2393156642875615969, -0.9709418174260511236 ) ) ;
#18065=VECTOR ( 'NONE', #35094, 1000.000000000000000 ) ;
#18068=PLANE ( 'NONE',  #20574 ) ;
#18080=DIRECTION ( 'NONE',  ( 1.000000000000000000, -0.000000000000000000, -0.000000000000000000 ) ) ;
#18081=AXIS2_PLACEMENT_3D ( 'NONE', #25243, #17111, #531 ) ;
#18082=EDGE_LOOP ( 'NONE', ( #42337, #11323, #33106, #1401 ) ) ;
#18084=VERTEX_POINT ( 'NONE', #41380 ) ;
#18096=PLANE ( 'NONE',  #31368 ) ;
#18099=ORIENTED_EDGE ( 'NONE', *, *, #1467, .F. ) ;
#18100=ORIENTED_EDGE ( 'NONE', *, *, #42671, .T. ) ;
#18102=DIRECTION ( 'NONE',  ( 0.000000000000000000, 0.000000000000000000, 1.000000000000000000 ) ) ;
#18104=VECTOR ( 'NONE', #2899, 1000.000000000000000 ) ;
#18106=ORIENTED_EDGE ( 'NONE', *, *, #18496, .F. ) ;
#18112=VECTOR ( 'NONE', #33126, 1000.000000000000000 ) ;
#18115=DIRECTION ( 'NONE',  ( 0.000000000000000000, 0.9350162426854158326, 0.3546048870425331234 ) ) ;
#18117=CARTESIAN_POINT ( 'NONE',  ( -336.3521761649654422, -64.61288906875131488, 4.498567634385603142 ) ) ;
#18119=DIRECTION ( 'NONE',  ( 0.000000000000000000, 0.3546048870425426158, 0.9350162426854121689 ) ) ;
#18120=EDGE_CURVE ( 'NONE', #4224, #1505, #9852, .T. ) ;
#18127=EDGE_CURVE ( 'NONE', #37502, #16440, #44220, .T. ) ;
#18129=DIRECTION ( 'NONE',  ( -0.000000000000000000, 0.000000000000000000, 1.000000000000000000 ) ) ;
#18132=CARTESIAN_POINT ( 'NONE',  ( -339.1964088526558498, -171.7720157143604069, -33.92731199008472487 ) ) ;
#18134=EDGE_CURVE ( 'NONE', #23565, #32390, #50836, .T. ) ;
#18136=CARTESIAN_POINT ( 'NONE',  ( -336.3521761649653854, -65.65568511206123503, -15.93848283698870105 ) ) ;
#18146=ORIENTED_EDGE ( 'NONE', *, *, #17351, .T. ) ;
#18148=ORIENTED_EDGE ( 'NONE', *, *, #34041, .F. ) ;
#18150=FACE_OUTER_BOUND ( 'NONE', #40949, .T. ) ;
#18153=EDGE_CURVE ( 'NONE', #42349, #42007, #42150, .T. ) ;
#18156=DIRECTION ( 'NONE',  ( -1.000000000000000000, 0.000000000000000000, -0.000000000000000000 ) ) ;
#18157=PLANE ( 'NONE',  #20127 ) ;
#18160=VERTEX_POINT ( 'NONE', #18511 ) ;
#18161=VECTOR ( 'NONE', #8969, 1000.000000000000000 ) ;
#18162=DIRECTION ( 'NONE',  ( -1.000000000000000000, -1.036104688092335575E-14, 1.258058860540570666E-15 ) ) ;
#18163=ADVANCED_FACE ( 'NONE', ( #34282 ), #25875, .F. ) ;
#18165=VECTOR ( 'NONE', #20584, 1000.000000000000000 ) ;
#18166=LINE ( 'NONE', #42587, #8660 ) ;
#18171=CARTESIAN_POINT ( 'NONE',  ( -336.3521761649654422, -119.0014323656137947, -58.88711093124865670 ) ) ;
#18176=CARTESIAN_POINT ( 'NONE',  ( -339.1964088526558498, -138.1050951016783301, 57.16590939599346655 ) ) ;
#18178=VERTEX_POINT ( 'NONE', #50063 ) ;
#18183=DIRECTION ( 'NONE',  ( 1.000000000000000000, 0.000000000000000000, 0.000000000000000000 ) ) ;
#18185=VECTOR ( 'NONE', #51378, 1000.000000000000000 ) ;
#18186=VERTEX_POINT ( 'NONE', #10881 ) ;
#18187=ORIENTED_EDGE ( 'NONE', *, *, #20419, .F. ) ;
#18191=EDGE_CURVE ( 'NONE', #42079, #34284, #42418, .T. ) ;
#18195=ORIENTED_EDGE ( 'NONE', *, *, #38838, .F. ) ;
#18200=CARTESIAN_POINT ( 'NONE',  ( -332.3517673607765914, -159.1821513111375452, -47.06073758877369073 ) ) ;
#18204=CARTESIAN_POINT ( 'NONE',  ( -330.4913330509368166, -180.6659093959932250, 14.60509510167933556 ) ) ;
#18211=DIRECTION ( 'NONE',  ( 0.000000000000000000, 0.8854560256532044704, -0.4647231720437789981 ) ) ;
#18214=CARTESIAN_POINT ( 'NONE',  ( -305.0000000000000568, -176.3931552210903249, -28.32515014536811648 ) ) ;
#18216=DIRECTION ( 'NONE',  ( -1.000000000000000000, 0.000000000000000000, -0.000000000000000000 ) ) ;
#18217=ORIENTED_EDGE ( 'NONE', *, *, #37892, .T. ) ;
#18220=ORIENTED_EDGE ( 'NONE', *, *, #10944, .F. ) ;
#18221=FACE_BOUND ( 'NONE', #27162, .T. ) ;
#18222=DIRECTION ( 'NONE',  ( 1.000000000000000000, -0.000000000000000000, -0.000000000000000000 ) ) ;
#18223=ORIENTED_EDGE ( 'NONE', *, *, #31698, .T. ) ;
#18225=ORIENTED_EDGE ( 'NONE', *, *, #3459, .F. ) ;
#18228=CIRCLE ( 'NONE', #24939, 60.00000000000000000 ) ;
#18229=CARTESIAN_POINT ( 'NONE',  ( -339.1964088526558498, -162.9984922102920848, 43.83057281297495678 ) ) ;
#18233=DIRECTION ( 'NONE',  ( -0.000000000000000000, 0.8854560256532043594, -0.4647231720437789981 ) ) ;
#18238=CIRCLE ( 'NONE', #47610, 60.00000000000000000 ) ;
#18239=VERTEX_POINT ( 'NONE', #34523 ) ;
#18240=EDGE_CURVE ( 'NONE', #20222, #37538, #50572, .T. ) ;
#18250=EDGE_CURVE ( 'NONE', #10838, #17726, #23487, .T. ) ;
#18257=LINE ( 'NONE', #34278, #4003 ) ;
#18261=CARTESIAN_POINT ( 'NONE',  ( -339.1964088526558498, -64.99044476834248485, -7.608018572113150135 ) ) ;
#18263=ORIENTED_EDGE ( 'NONE', *, *, #38521, .F. ) ;
#18265=ADVANCED_FACE ( 'NONE', ( #43186 ), #31102, .F. ) ;
#18267=CARTESIAN_POINT ( 'NONE',  ( -305.0000000000000568, -179.7763290203208726, -20.80804632820190392 ) ) ;
#18269=VECTOR ( 'NONE', #34782, 1000.000000000000000 ) ;
#18270=EDGE_CURVE ( 'NONE', #16896, #18800, #35301, .T. ) ;
#18274=CARTESIAN_POINT ( 'NONE',  ( -336.3521761649654422, -85.59754891220836726, -45.24454186338619621 ) ) ;
#18279=EDGE_CURVE ( 'NONE', #4817, #28748, #42929, .T. ) ;
#18282=DIRECTION ( 'NONE',  ( 1.000000000000000000, -0.000000000000000000, -0.000000000000000000 ) ) ;
#18284=CARTESIAN_POINT ( 'NONE',  ( -330.4913330509368166, -96.52406086224436876, -52.47426709956133806 ) ) ;
#18285=LINE ( 'NONE', #1471, #24264 ) ;
#18286=VERTEX_POINT ( 'NONE', #39498 ) ;
#18287=CARTESIAN_POINT ( 'NONE',  ( -336.3521761649653854, -152.8183901354257159, -52.34913561719022113 ) ) ;
#18289=EDGE_CURVE ( 'NONE', #1436, #15388, #11380, .T. ) ;
#18291=CARTESIAN_POINT ( 'NONE',  ( -339.1964088526558498, -108.8949048983213004, -57.16590939599337418 ) ) ;
#18295=ORIENTED_EDGE ( 'NONE', *, *, #6677, .F. ) ;
#18304=AXIS2_PLACEMENT_3D ( 'NONE', #667, #45346, #44808 ) ;
#18305=FACE_OUTER_BOUND ( 'NONE', #3550, .T. ) ;
#18306=VERTEX_POINT ( 'NONE', #51874 ) ;
#18308=ORIENTED_EDGE ( 'NONE', *, *, #37175, .T. ) ;
#18312=ORIENTED_EDGE ( 'NONE', *, *, #16647, .T. ) ;
#18316=FACE_OUTER_BOUND ( 'NONE', #19426, .T. ) ;
#18325=DIRECTION ( 'NONE',  ( 0.000000000000000000, -0.5680647467311485954, 0.8229838658936613482 ) ) ;
#18329=EDGE_CURVE ( 'NONE', #903, #29300, #2989, .T. ) ;
#18336=ADVANCED_FACE ( 'NONE', ( #19029 ), #7464, .F. ) ;
#18338=PLANE ( 'NONE',  #41645 ) ;
#18340=CARTESIAN_POINT ( 'NONE',  ( -365.0000000000001137, -78.50000000000002842, -5.000000000000001776 ) ) ;
#18347=ORIENTED_EDGE ( 'NONE', *, *, #45690, .T. ) ;
#18351=DIRECTION ( 'NONE',  ( -1.000000000000000000, -0.000000000000000000, -0.000000000000000000 ) ) ;
#18356=CARTESIAN_POINT ( 'NONE',  ( -339.1964088526558498, -123.5000000000000284, 0.000000000000000000 ) ) ;
#18360=DIRECTION ( 'NONE',  ( 0.000000000000000000, 0.9709418174260553425, 0.2393156642875449158 ) ) ;
#18362=ORIENTED_EDGE ( 'NONE', *, *, #8409, .F. ) ;
#18363=CARTESIAN_POINT ( 'NONE',  ( -332.3517673607765914, -87.81784868886214213, 47.06073758877343494 ) ) ;
#18365=CARTESIAN_POINT ( 'NONE',  ( -336.3521761649654422, -105.0395444947681369, -56.09938080879045685 ) ) ;
#18367=ORIENTED_EDGE ( 'NONE', *, *, #44895, .T. ) ;
#18368=VECTOR ( 'NONE', #2503, 1000.000000000000000 ) ;
#18371=VECTOR ( 'NONE', #28576, 1000.000000000000000 ) ;
#18375=EDGE_CURVE ( 'NONE', #7178, #49884, #5678, .T. ) ;
#18376=CARTESIAN_POINT ( 'NONE',  ( 0.000000000000000000, -150.9186671505818822, 52.24190551353965617 ) ) ;
#18379=FACE_OUTER_BOUND ( 'NONE', #7065, .T. ) ;
#18380=CARTESIAN_POINT ( 'NONE',  ( -336.3521761649654422, -121.8677111499054320, 59.00000000000001421 ) ) ;
#18382=LINE ( 'NONE', #34401, #20763 ) ;
#18387=EDGE_LOOP ( 'NONE', ( #51488, #47883 ) ) ;
#18394=FACE_OUTER_BOUND ( 'NONE', #6387, .T. ) ;
#18410=VECTOR ( 'NONE', #6221, 1000.000000000000000 ) ;
#18415=EDGE_LOOP ( 'NONE', ( #16225, #32279, #32621, #8112 ) ) ;
#18416=DIRECTION ( 'NONE',  ( 0.000000000000000000, 0.5680647467311596976, 0.8229838658936536877 ) ) ;
#18417=LINE ( 'NONE', #50228, #6539 ) ;
#18418=LINE ( 'NONE', #46283, #14863 ) ;
#18420=LINE ( 'NONE', #46532, #46730 ) ;
#18422=DIRECTION ( 'NONE',  ( -1.000000000000000000, 0.000000000000000000, 0.000000000000000000 ) ) ;
#18423=DIRECTION ( 'NONE',  ( -1.000000000000000000, -0.000000000000000000, 0.000000000000000000 ) ) ;
#18425=EDGE_CURVE ( 'NONE', #50508, #21465, #51809, .T. ) ;
#18429=DIRECTION ( 'NONE',  ( 0.000000000000000000, 0.000000000000000000, 1.000000000000000000 ) ) ;
#18435=ADVANCED_FACE ( 'NONE', ( #24260 ), #44748, .F. ) ;
#18437=LINE ( 'NONE', #34452, #3502 ) ;
#18439=CARTESIAN_POINT ( 'NONE',  ( -305.0000000000000568, -173.7880015656344312, -32.72792230702632565 ) ) ;
#18441=ORIENTED_EDGE ( 'NONE', *, *, #26005, .F. ) ;
#18453=DIRECTION ( 'NONE',  ( 0.000000000000000000, -0.3546048870425463906, -0.9350162426854107256 ) ) ;
#18459=ORIENTED_EDGE ( 'NONE', *, *, #30878, .F. ) ;
#18460=DIRECTION ( 'NONE',  ( 1.000000000000000000, -0.000000000000000000, -0.000000000000000000 ) ) ;
#18461=VERTEX_POINT ( 'NONE', #41310 ) ;
#18465=ORIENTED_EDGE ( 'NONE', *, *, #52003, .T. ) ;
#18466=CARTESIAN_POINT ( 'NONE',  ( -336.3521761649653854, -177.3662605214052519, -26.42775013958059560 ) ) ;
#18467=CARTESIAN_POINT ( 'NONE',  ( -330.4913330509368166, -66.33409060400670398, -14.60509510167892522 ) ) ;
#18473=ORIENTED_EDGE ( 'NONE', *, *, #17935, .F. ) ;
#18475=FACE_OUTER_BOUND ( 'NONE', #49675, .T. ) ;
#18478=ORIENTED_EDGE ( 'NONE', *, *, #497, .F. ) ;
#18481=CARTESIAN_POINT ( 'NONE',  ( -340.0000000000000568, -123.5000000000000284, -60.00000000000000000 ) ) ;
#18482=CYLINDRICAL_SURFACE ( 'NONE', #37832, 20.00000000000001066 ) ;
#18483=ORIENTED_EDGE ( 'NONE', *, *, #25665, .T. ) ;
#18484=DIRECTION ( 'NONE',  ( 1.000000000000000000, 7.175085443855111658E-17, 4.952603889764001357E-17 ) ) ;
#18491=ORIENTED_EDGE ( 'NONE', *, *, #37103, .F. ) ;
#18493=DIRECTION ( 'NONE',  ( -1.000000000000000000, -0.000000000000000000, 0.000000000000000000 ) ) ;
#18494=VERTEX_POINT ( 'NONE', #28442 ) ;
#18495=EDGE_CURVE ( 'NONE', #19422, #48723, #8473, .T. ) ;
#18496=EDGE_CURVE ( 'NONE', #46003, #22824, #36598, .T. ) ;
#18498=PLANE ( 'NONE',  #29354 ) ;
#18499=DIRECTION ( 'NONE',  ( -1.000000000000000000, 0.000000000000000000, 0.000000000000000000 ) ) ;
#18501=ORIENTED_EDGE ( 'NONE', *, *, #36103, .T. ) ;
#18502=PLANE ( 'NONE',  #8985 ) ;
#18504=ORIENTED_EDGE ( 'NONE', *, *, #45593, .F. ) ;
#18511=CARTESIAN_POINT ( 'NONE',  ( -339.1964088526558498, -131.2283041299240836, 59.50019592636143528 ) ) ;
#18517=CARTESIAN_POINT ( 'NONE',  ( -365.0000000000001137, -78.50000000000002842, 0.000000000000000000 ) ) ;
#18519=VERTEX_POINT ( 'NONE', #12381 ) ;
#18522=AXIS2_PLACEMENT_3D ( 'NONE', #44691, #4748, #49161 ) ;
#18529=FACE_OUTER_BOUND ( 'NONE', #3567, .T. ) ;
#18534=LINE ( 'NONE', #35328, #11689 ) ;
#18538=LINE ( 'NONE', #14341, #45575 ) ;
#18540=DIRECTION ( 'NONE',  ( 1.000000000000000000, -0.000000000000000000, 0.000000000000000000 ) ) ;
#18546=EDGE_CURVE ( 'NONE', #39327, #21742, #28141, .T. ) ;
#18547=DIRECTION ( 'NONE',  ( -0.000000000000000000, -0.3546048870425396182, -0.9350162426854132791 ) ) ;
#18549=DIRECTION ( 'NONE',  ( -0.000000000000000000, -0.9709418174260534551, -0.2393156642875516327 ) ) ;
#18551=ADVANCED_FACE ( 'NONE', ( #48400 ), #42563, .T. ) ;
#18553=EDGE_LOOP ( 'NONE', ( #16801, #27351, #15555, #20968 ) ) ;
#18563=DIRECTION ( 'NONE',  ( 0.000000000000000000, 0.4647231720437789981, 0.8854560256532044704 ) ) ;
#18565=CARTESIAN_POINT ( 'NONE',  ( -330.4913330509368166, -182.5000000000000568, 0.4999999999999549249 ) ) ;
#18566=DIRECTION ( 'NONE',  ( -1.000000000000000000, 0.000000000000000000, 0.000000000000000000 ) ) ;
#18567=DIRECTION ( 'NONE',  ( -0.000000000000000000, 0.8229838658936556861, -0.5680647467311569221 ) ) ;
#18569=EDGE_LOOP ( 'NONE', ( #45298, #31057, #23613, #38344 ) ) ;
#18570=ORIENTED_EDGE ( 'NONE', *, *, #843, .F. ) ;
#18571=VERTEX_POINT ( 'NONE', #8704 ) ;
#18573=DIRECTION ( 'NONE',  ( -0.000000000000000000, 0.4647231720437573488, -0.8854560256532157947 ) ) ;
#18574=VECTOR ( 'NONE', #42093, 1000.000000000000000 ) ;
#18575=LINE ( 'NONE', #21747, #15894 ) ;
#18576=DIRECTION ( 'NONE',  ( 0.000000000000000000, 0.000000000000000000, -1.000000000000000000 ) ) ;
#18582=DIRECTION ( 'NONE',  ( -0.000000000000000000, 0.1205366802553337752, 0.9927088740980526405 ) ) ;
#18584=ORIENTED_EDGE ( 'NONE', *, *, #17690, .T. ) ;
#18587=DIRECTION ( 'NONE',  ( 1.000000000000000000, 0.000000000000000000, 0.000000000000000000 ) ) ;
#18591=LINE ( 'NONE', #10705, #38068 ) ;
#18593=EDGE_CURVE ( 'NONE', #29662, #49548, #18417, .T. ) ;
#18594=CARTESIAN_POINT ( 'NONE',  ( -339.1964088526558498, -131.2283041299249930, -59.50019592636133581 ) ) ;
#18600=EDGE_LOOP ( 'NONE', ( #51774, #14617, #47697, #51067 ) ) ;
#18606=LINE ( 'NONE', #39843, #34917 ) ;
#18607=DIRECTION ( 'NONE',  ( -1.000000000000000000, 0.000000000000000000, 0.000000000000000000 ) ) ;
#18608=DIRECTION ( 'NONE',  ( 0.000000000000000000, 0.7485107481711024136, 0.6631226582407937498 ) ) ;
#18614=VECTOR ( 'NONE', #16166, 1000.000000000000000 ) ;
#18615=ADVANCED_FACE ( 'NONE', ( #2387 ), #10263, .F. ) ;
#18617=ORIENTED_EDGE ( 'NONE', *, *, #50811, .T. ) ;
#18618=VECTOR ( 'NONE', #37252, 1000.000000000000114 ) ;
#18619=EDGE_CURVE ( 'NONE', #5479, #48164, #9237, .T. ) ;
#18621=CARTESIAN_POINT ( 'NONE',  ( -339.1964088526558498, -176.8578783931336602, 27.43969411971573891 ) ) ;
#18622=ADVANCED_FACE ( 'NONE', ( #42305 ), #29977, .F. ) ;
#18624=CARTESIAN_POINT ( 'NONE',  ( -330.4913330509368166, -167.9936954712150339, 38.74998146212178796 ) ) ;
#18625=EDGE_LOOP ( 'NONE', ( #45454, #50978, #19219, #11618 ) ) ;
#18628=DIRECTION ( 'NONE',  ( 1.000000000000000000, 0.000000000000000000, 0.000000000000000000 ) ) ;
#18630=CARTESIAN_POINT ( 'NONE',  ( -336.3521761649654422, -174.9833430614318388, 28.86398714850502856 ) ) ;
#18634=DIRECTION ( 'NONE',  ( 0.000000000000000000, 0.000000000000000000, 1.000000000000000000 ) ) ;
#18643=VECTOR ( 'NONE', #1361, 1000.000000000000000 ) ;
#18648=CARTESIAN_POINT ( 'NONE',  ( -330.4913330509368166, -167.3305728129743102, 39.49849221029282376 ) ) ;
#18651=CONICAL_SURFACE ( 'NONE', #48022, 10.00000000000000711, 0.03490658503988659789 ) ;
#18652=CARTESIAN_POINT ( 'NONE',  ( -305.0000000000000568, -110.7312321683605916, -58.62557946887767457 ) ) ;
#18653=VERTEX_POINT ( 'NONE', #46030 ) ;
#18660=CARTESIAN_POINT ( 'NONE',  ( -339.1964088526558498, -122.9999999999993747, 59.00000000000002132 ) ) ;
#18667=CARTESIAN_POINT ( 'NONE',  ( -339.1964088526558498, -123.9999999999993747, 59.00000000000002132 ) ) ;
#18672=CARTESIAN_POINT ( 'NONE',  ( -339.1964088526558498, -180.9052250602807703, 13.63415328425337236 ) ) ;
#18673=VECTOR ( 'NONE', #30942, 1000.000000000000000 ) ;
#18677=FACE_OUTER_BOUND ( 'NONE', #35837, .T. ) ;
#18683=EDGE_CURVE ( 'NONE', #10791, #26860, #51854, .T. ) ;
#18685=CARTESIAN_POINT ( 'NONE',  ( -339.1964088526558498, -68.51134412508183402, -21.38919645685240312 ) ) ;
#18692=VECTOR ( 'NONE', #14753, 1000.000000000000114 ) ;
#18694=CARTESIAN_POINT ( 'NONE',  ( -336.3521761649653854, -132.3499116637027271, -59.34373651485605450 ) ) ;
#18695=ORIENTED_EDGE ( 'NONE', *, *, #10752, .F. ) ;
#18696=AXIS2_PLACEMENT_3D ( 'NONE', #10735, #11501, #35160 ) ;
#18697=LINE ( 'NONE', #36919, #46166 ) ;
#18701=VERTEX_POINT ( 'NONE', #41530 ) ;
#18702=CARTESIAN_POINT ( 'NONE',  ( -330.4913330509368166, -123.5000000000000284, 0.000000000000000000 ) ) ;
#18703=CIRCLE ( 'NONE', #24582, 60.00000000000000000 ) ;
#18709=FACE_OUTER_BOUND ( 'NONE', #47936, .T. ) ;
#18712=ORIENTED_EDGE ( 'NONE', *, *, #36631, .F. ) ;
#18717=EDGE_CURVE ( 'NONE', #3693, #10327, #4847, .T. ) ;
#18718=DIRECTION ( 'NONE',  ( -1.000000000000000000, -0.000000000000000000, 0.000000000000000000 ) ) ;
#18723=VERTEX_POINT ( 'NONE', #19432 ) ;
#18728=ORIENTED_EDGE ( 'NONE', *, *, #37238, .T. ) ;
#18731=ORIENTED_EDGE ( 'NONE', *, *, #17600, .F. ) ;
#18732=DIRECTION ( 'NONE',  ( 0.000000000000000000, 0.000000000000000000, -1.000000000000000000 ) ) ;
#18742=AXIS2_PLACEMENT_3D ( 'NONE', #45259, #13183, #40298 ) ;
#18744=DIRECTION ( 'NONE',  ( -1.000000000000000000, 0.000000000000000000, -0.000000000000000000 ) ) ;
#18746=AXIS2_PLACEMENT_3D ( 'NONE', #17488, #41627, #45341 ) ;
#18748=LINE ( 'NONE', #46612, #47250 ) ;
#18749=CARTESIAN_POINT ( 'NONE',  ( -330.4913330509368166, -143.9541802141672235, -55.34326076196065003 ) ) ;
#18750=DIRECTION ( 'NONE',  ( 1.000000000000000000, 0.000000000000000000, 0.000000000000000000 ) ) ;
#18752=ORIENTED_EDGE ( 'NONE', *, *, #39632, .F. ) ;
#18753=VERTEX_POINT ( 'NONE', #51256 ) ;
#18757=PLANE ( 'NONE',  #51465 ) ;
#18758=VECTOR ( 'NONE', #38294, 999.9999999999998863 ) ;
#18762=LINE ( 'NONE', #26649, #45174 ) ;
#18765=CARTESIAN_POINT ( 'NONE',  ( -332.3517673607765914, -135.0638248728647852, 57.91551518289418254 ) ) ;
#18766=ORIENTED_EDGE ( 'NONE', *, *, #13578, .T. ) ;
#18775=EDGE_LOOP ( 'NONE', ( #43521, #42817, #18954, #13774 ) ) ;
#18776=ADVANCED_FACE ( 'NONE', ( #34936 ), #2888, .F. ) ;
#18779=VECTOR ( 'NONE', #45782, 1000.000000000000000 ) ;
#18782=DIRECTION ( 'NONE',  ( 0.000000000000000000, -0.9709418174260553425, -0.2393156642875449158 ) ) ;
#18783=EDGE_CURVE ( 'NONE', #21100, #14977, #49218, .T. ) ;
#18786=DIRECTION ( 'NONE',  ( -1.000000000000000000, -0.000000000000000000, -0.000000000000000000 ) ) ;
#18800=VERTEX_POINT ( 'NONE', #39645 ) ;
#18805=VECTOR ( 'NONE', #7605, 1000.000000000000000 ) ;
#18806=ORIENTED_EDGE ( 'NONE', *, *, #42016, .F. ) ;
#18814=LINE ( 'NONE', #18565, #3131 ) ;
#18816=ADVANCED_FACE ( 'NONE', ( #30738 ), #18920, .F. ) ;
#18819=CARTESIAN_POINT ( 'NONE',  ( -339.1964088526558498, -74.65991953890826949, 33.10432812419072945 ) ) ;
#18823=CARTESIAN_POINT ( 'NONE',  ( 0.000000000000000000, -130.6116641350635064, 58.56982357178529242 ) ) ;
#18825=DIRECTION ( 'NONE',  ( -1.000000000000000000, 0.000000000000000000, -0.000000000000000000 ) ) ;
#18828=VERTEX_POINT ( 'NONE', #31005 ) ;
#18829=ADVANCED_FACE ( 'NONE', ( #6839 ), #22865, .T. ) ;
#18831=CARTESIAN_POINT ( 'NONE',  ( -332.3517673607765914, -72.48138011061176655, -29.74944317415788930 ) ) ;
#18836=EDGE_CURVE ( 'NONE', #49548, #4472, #10508, .T. ) ;
#18843=CARTESIAN_POINT ( 'NONE',  ( -340.0000000000000568, -168.5000000000000284, 5.000000000000001776 ) ) ;
#18847=AXIS2_PLACEMENT_3D ( 'NONE', #26362, #46105, #14814 ) ;
#18848=ORIENTED_EDGE ( 'NONE', *, *, #46097, .F. ) ;
#18851=DIRECTION ( 'NONE',  ( 0.000000000000000000, 5.851800525628429686E-14, 1.000000000000000000 ) ) ;
#18857=EDGE_LOOP ( 'NONE', ( #10736, #6967, #7409, #25692 ) ) ;
#18868=EDGE_CURVE ( 'NONE', #47538, #10327, #11553, .T. ) ;
#18874=VECTOR ( 'NONE', #48058, 1000.000000000000000 ) ;
#18882=ADVANCED_FACE ( 'NONE', ( #48866 ), #23887, .F. ) ;
#18885=ORIENTED_EDGE ( 'NONE', *, *, #38165, .F. ) ;
#18887=AXIS2_PLACEMENT_3D ( 'NONE', #4424, #36464, #19935 ) ;
#18889=AXIS2_PLACEMENT_3D ( 'NONE', #44022, #36132, #4094 ) ;
#18890=ADVANCED_FACE ( 'NONE', ( #28079 ), #35990, .F. ) ;
#18892=ADVANCED_FACE ( 'NONE', ( #44652 ), #43859, .T. ) ;
#18894=DIRECTION ( 'NONE',  ( -1.000000000000000000, 0.000000000000000000, 0.000000000000000000 ) ) ;
#18895=PLANE ( 'NONE',  #45891 ) ;
#18898=SURFACE_STYLE_FILL_AREA ( #2867 ) ;
#18899=VERTEX_POINT ( 'NONE', #3932 ) ;
#18902=ORIENTED_EDGE ( 'NONE', *, *, #22279, .T. ) ;
#18910=ORIENTED_EDGE ( 'NONE', *, *, #10754, .T. ) ;
#18913=CARTESIAN_POINT ( 'NONE',  ( -305.0000000000000568, -117.8908635894569272, -59.73723787327232060 ) ) ;
#18914=EDGE_LOOP ( 'NONE', ( #48804, #6433, #11692, #12511 ) ) ;
#18915=PLANE ( 'NONE',  #32870 ) ;
#18916=VECTOR ( 'NONE', #27057, 1000.000000000000000 ) ;
#18918=ORIENTED_EDGE ( 'NONE', *, *, #6729, .T. ) ;
#18920=PLANE ( 'NONE',  #632 ) ;
#18921=DIRECTION ( 'NONE',  ( -0.000000000000000000, 0.9350162426854146114, -0.3546048870425363986 ) ) ;
#18928=ADVANCED_FACE ( 'NONE', ( #16024 ), #40681, .F. ) ;
#18930=VECTOR ( 'NONE', #44857, 1000.000000000000000 ) ;
#18931=CARTESIAN_POINT ( 'NONE',  ( -330.4913330509368166, -172.3400804610910200, 33.10432812419180948 ) ) ;
#18933=CARTESIAN_POINT ( 'NONE',  ( -332.3517673607765914, -123.5000000000000284, 0.000000000000000000 ) ) ;
#18938=DIRECTION ( 'NONE',  ( 1.000000000000000000, 0.000000000000000000, 0.000000000000000000 ) ) ;
#18940=VECTOR ( 'NONE', #10898, 1000.000000000000114 ) ;
#18941=AXIS2_PLACEMENT_3D ( 'NONE', #33829, #47164, #37257 ) ;
#18948=ADVANCED_FACE ( 'NONE', ( #44401 ), #40957, .F. ) ;
#18951=EDGE_CURVE ( 'NONE', #39885, #22194, #483, .T. ) ;
#18952=EDGE_CURVE ( 'NONE', #13133, #22275, #31791, .T. ) ;
#18954=ORIENTED_EDGE ( 'NONE', *, *, #47034, .F. ) ;
#18959=DIRECTION ( 'NONE',  ( -0.000000000000000000, -0.1205366802553130001, 0.9927088740980551940 ) ) ;
#18960=AXIS2_PLACEMENT_3D ( 'NONE', #761, #29125, #21513 ) ;
#18961=AXIS2_PLACEMENT_3D ( 'NONE', #27592, #31525, #23640 ) ;
#18962=LINE ( 'NONE', #43399, #37891 ) ;
#18965=CARTESIAN_POINT ( 'NONE',  ( -332.3517673607765914, -111.9361751271348879, -57.91551518289410438 ) ) ;
#18968=ORIENTED_EDGE ( 'NONE', *, *, #9575, .F. ) ;
#18970=VECTOR ( 'NONE', #44828, 1000.000000000000114 ) ;
#18971=CIRCLE ( 'NONE', #26502, 60.00000000000000000 ) ;
#18974=CARTESIAN_POINT ( 'NONE',  ( -336.3521761649653854, -162.0508476703726330, 45.97643030831914501 ) ) ;
#18983=VECTOR ( 'NONE', #16789, 1000.000000000000000 ) ;
#18985=CARTESIAN_POINT ( 'NONE',  ( -339.1964088526558498, -84.75001853787875916, -44.49369547121548862 ) ) ;
#18988=LINE ( 'NONE', #26858, #33295 ) ;
#18991=FACE_BOUND ( 'NONE', #37638, .T. ) ;
#18994=CARTESIAN_POINT ( 'NONE',  ( -339.1964088526558498, -84.75001853787875916, -44.49369547121548862 ) ) ;
#18996=AXIS2_PLACEMENT_3D ( 'NONE', #40125, #3875, #35150 ) ;
#19002=CARTESIAN_POINT ( 'NONE',  ( -339.1964088526558498, -89.57268800991514013, -48.27201571436026484 ) ) ;
#19003=CARTESIAN_POINT ( 'NONE',  ( -332.3517673607765914, -80.37812621821328207, -41.71934804796994456 ) ) ;
#19004=DIRECTION ( 'NONE',  ( -1.000000000000000000, 0.000000000000000000, 0.000000000000000000 ) ) ;
#19011=FACE_OUTER_BOUND ( 'NONE', #17944, .T. ) ;
#19012=VERTEX_POINT ( 'NONE', #29128 ) ;
#19013=AXIS2_PLACEMENT_3D ( 'NONE', #22803, #30420, #46465 ) ;
#19015=EDGE_CURVE ( 'NONE', #47856, #16704, #13625, .T. ) ;
#19018=VECTOR ( 'NONE', #31939, 1000.000000000000000 ) ;
#19020=DIRECTION ( 'NONE',  ( 0.000000000000000000, 0.4647231720437695057, 0.8854560256532093554 ) ) ;
#19029=FACE_OUTER_BOUND ( 'NONE', #199, .T. ) ;
#19041=ORIENTED_EDGE ( 'NONE', *, *, #34971, .T. ) ;
#19043=LINE ( 'NONE', #46914, #35693 ) ;
#19045=ORIENTED_EDGE ( 'NONE', *, *, #26943, .F. ) ;
#19048=CARTESIAN_POINT ( 'NONE',  ( -332.3517673607765914, -65.24746378767824240, -9.724760635741734660 ) ) ;
#19052=CARTESIAN_POINT ( 'NONE',  ( -305.0000000000000568, -71.15086438280971493, -29.31839013542551342 ) ) ;
#19057=ORIENTED_EDGE ( 'NONE', *, *, #23168, .T. ) ;
#19058=LINE ( 'NONE', #6716, #14175 ) ;
#19060=VECTOR ( 'NONE', #1962, 999.9999999999998863 ) ;
#19062=VERTEX_POINT ( 'NONE', #6001 ) ;
#19072=VERTEX_POINT ( 'NONE', #21516 ) ;
#19075=CARTESIAN_POINT ( 'NONE',  ( 0.000000000000000000, -167.6621341420946578, 39.12423683620730230 ) ) ;
#19076=CARTESIAN_POINT ( 'NONE',  ( -332.3517673607765914, -123.5000000000000284, 0.000000000000000000 ) ) ;
#19078=AXIS2_PLACEMENT_3D ( 'NONE', #20765, #16835, #24440 ) ;
#19080=DIRECTION ( 'NONE',  ( 1.000000000000000000, -0.000000000000000000, -0.000000000000000000 ) ) ;
#19081=ADVANCED_FACE ( 'NONE', ( #38045 ), #5764, .T. ) ;
#19087=ORIENTED_EDGE ( 'NONE', *, *, #51025, .T. ) ;
#19088=PLANE ( 'NONE',  #23097 ) ;
#19089=VECTOR ( 'NONE', #24451, 1000.000000000000000 ) ;
#19090=DIRECTION ( 'NONE',  ( -0.000000000000000000, 0.1205366802553337752, 0.9927088740980526405 ) ) ;
#19093=AXIS2_PLACEMENT_3D ( 'NONE', #9100, #21430, #9356 ) ;
#19094=LINE ( 'NONE', #31686, #17729 ) ;
#19095=LINE ( 'NONE', #19598, #19018 ) ;
#19098=ORIENTED_EDGE ( 'NONE', *, *, #37534, .F. ) ;
#19105=CARTESIAN_POINT ( 'NONE',  ( -332.3517673607765914, -103.7577981350106313, -56.65902810251876787 ) ) ;
#19108=ORIENTED_EDGE ( 'NONE', *, *, #41035, .T. ) ;
#19110=ORIENTED_EDGE ( 'NONE', *, *, #49356, .T. ) ;
#19111=VECTOR ( 'NONE', #41590, 1000.000000000000000 ) ;
#19114=CARTESIAN_POINT ( 'NONE',  ( -330.4913330509368166, -130.1153096980153236, -58.63009191191284941 ) ) ;
#19117=DIRECTION ( 'NONE',  ( 0.000000000000000000, 0.7485107481711024136, 0.6631226582407937498 ) ) ;
#19121=VERTEX_POINT ( 'NONE', #16150 ) ;
#19123=DIRECTION ( 'NONE',  ( 0.000000000000000000, -0.8229838658936556861, 0.5680647467311569221 ) ) ;
#19126=ORIENTED_EDGE ( 'NONE', *, *, #6452, .F. ) ;
#19130=EDGE_CURVE ( 'NONE', #33399, #21096, #45880, .T. ) ;
#19131=CARTESIAN_POINT ( 'NONE',  ( -490.0000000000001137, -168.5000000000000284, 0.000000000000000000 ) ) ;
#19136=VECTOR ( 'NONE', #48388, 1000.000000000000000 ) ;
#19137=CARTESIAN_POINT ( 'NONE',  ( -330.4913330509368166, -89.57268800991514013, -48.27201571436026484 ) ) ;
#19138=ORIENTED_EDGE ( 'NONE', *, *, #28258, .F. ) ;
#19142=DIRECTION ( 'NONE',  ( 0.000000000000000000, 0.000000000000000000, -1.000000000000000000 ) ) ;
#19145=EDGE_CURVE ( 'NONE', #43547, #16663, #7270, .T. ) ;
#19147=CARTESIAN_POINT ( 'NONE',  ( -336.3521761649654422, -149.4733471526596134, 53.00046796564699036 ) ) ;
#19154=DIRECTION ( 'NONE',  ( 1.000000000000000000, -0.000000000000000000, -0.000000000000000000 ) ) ;
#19157=DIRECTION ( 'NONE',  ( 0.000000000000000000, 0.000000000000000000, 1.000000000000000000 ) ) ;
#19158=AXIS2_PLACEMENT_3D ( 'NONE', #21028, #43957, #40005 ) ;
#19161=AXIS2_PLACEMENT_3D ( 'NONE', #9674, #46458, #10438 ) ;
#19162=CARTESIAN_POINT ( 'NONE',  ( -339.1964088526558498, -167.9936954712150339, 38.74998146212178796 ) ) ;
#19164=EDGE_LOOP ( 'NONE', ( #22854, #18570, #48255, #7957 ) ) ;
#19172=CARTESIAN_POINT ( 'NONE',  ( -332.3517673607765914, -123.5000000000000284, 0.000000000000000000 ) ) ;
#19174=DIRECTION ( 'NONE',  ( -1.000000000000000000, 0.000000000000000000, 0.000000000000000000 ) ) ;
#19175=DIRECTION ( 'NONE',  ( 0.000000000000000000, 0.000000000000000000, 1.000000000000000000 ) ) ;
#19177=CARTESIAN_POINT ( 'NONE',  ( -330.4913330509368166, -96.52406086224436876, -52.47426709956133806 ) ) ;
#19180=CARTESIAN_POINT ( 'NONE',  ( -330.4913330509368166, -68.51134412508180560, -21.38919645685231075 ) ) ;
#19184=VECTOR ( 'NONE', #43587, 1000.000000000000000 ) ;
#19197=ADVANCED_FACE ( 'NONE', ( #24026 ), #42777, .T. ) ;
#19201=EDGE_CURVE ( 'NONE', #2635, #16080, #30944, .T. ) ;
#19205=CARTESIAN_POINT ( 'NONE',  ( -336.3521761649654422, -64.50000000000000000, -2.632288850093980503 ) ) ;
#19210=CIRCLE ( 'NONE', #32628, 60.00000000000000000 ) ;
#19215=DIRECTION ( 'NONE',  ( 1.000000000000000000, 0.000000000000000000, 0.000000000000000000 ) ) ;
#19219=ORIENTED_EDGE ( 'NONE', *, *, #48206, .T. ) ;
#19222=ORIENTED_EDGE ( 'NONE', *, *, #32416, .F. ) ;
#19223=AXIS2_PLACEMENT_3D ( 'NONE', #12068, #20758, #16569 ) ;
#19232=AXIS2_PLACEMENT_3D ( 'NONE', #30130, #14362, #21472 ) ;
#19233=DIRECTION ( 'NONE',  ( -0.000000000000000000, 0.1205366802553095168, -0.9927088740980556381 ) ) ;
#19234=PLANE ( 'NONE',  #26622 ) ;
#19241=CARTESIAN_POINT ( 'NONE',  ( -305.0000000000000568, -176.8578783931336602, 27.43969411971573891 ) ) ;
#19245=VECTOR ( 'NONE', #49571, 1000.000000000000000 ) ;
#19247=CARTESIAN_POINT ( 'NONE',  ( -330.4913330509368166, -95.63860483659048839, 52.00954392751722111 ) ) ;
#19248=ORIENTED_EDGE ( 'NONE', *, *, #24000, .F. ) ;
#19249=LINE ( 'NONE', #11082, #13903 ) ;
#19255=EDGE_CURVE ( 'NONE', #50353, #26805, #5597, .T. ) ;
#19259=FACE_BOUND ( 'NONE', #37471, .T. ) ;
#19260=CARTESIAN_POINT ( 'NONE',  ( -330.4913330509368166, -138.1050951016783301, 57.16590939599346655 ) ) ;
#19264=VERTEX_POINT ( 'NONE', #20597 ) ;
#19267=EDGE_CURVE ( 'NONE', #15270, #20782, #4574, .T. ) ;
#19270=AXIS2_PLACEMENT_3D ( 'NONE', #19356, #47223, #35368 ) ;
#19273=LINE ( 'NONE', #42905, #11481 ) ;
#19276=LINE ( 'NONE', #4528, #33833 ) ;
#19283=VERTEX_POINT ( 'NONE', #1408 ) ;
#19284=CARTESIAN_POINT ( 'NONE',  ( -330.4913330509368166, -123.5000000000000284, 0.000000000000000000 ) ) ;
#19287=CARTESIAN_POINT ( 'NONE',  ( -339.1964088526558498, -162.9984922102920848, 43.83057281297495678 ) ) ;
#19291=ORIENTED_EDGE ( 'NONE', *, *, #9515, .F. ) ;
#19293=LINE ( 'NONE', #26382, #23324 ) ;
#19299=EDGE_CURVE ( 'NONE', #20926, #7384, #12281, .T. ) ;
#19301=PLANE ( 'NONE',  #15125 ) ;
#19302=FACE_OUTER_BOUND ( 'NONE', #10745, .T. ) ;
#19304=FACE_OUTER_BOUND ( 'NONE', #10189, .T. ) ;
#19306=ORIENTED_EDGE ( 'NONE', *, *, #48094, .T. ) ;
#19308=ORIENTED_EDGE ( 'NONE', *, *, #17683, .T. ) ;
#19313=DIRECTION ( 'NONE',  ( -0.000000000000000000, 0.1205366802553337752, 0.9927088740980526405 ) ) ;
#19314=CARTESIAN_POINT ( 'NONE',  ( -336.3521761649654422, -179.2447759217480154, -19.39547174791710660 ) ) ;
#19317=ADVANCED_FACE ( 'NONE', ( #41092 ), #884, .F. ) ;
#19318=EDGE_LOOP ( 'NONE', ( #22875, #25760, #22426, #1462 ) ) ;
#19323=CARTESIAN_POINT ( 'NONE',  ( -490.0000000000001137, -168.5000000000000284, 0.000000000000000000 ) ) ;
#19328=DIRECTION ( 'NONE',  ( -1.000000000000000000, 6.921107616850842615E-15, 7.812315528781815670E-15 ) ) ;
#19331=ORIENTED_EDGE ( 'NONE', *, *, #39737, .T. ) ;
#19334=EDGE_CURVE ( 'NONE', #42991, #37560, #51772, .T. ) ;
#19335=DIRECTION ( 'NONE',  ( -0.000000000000000000, 0.5680647467311656929, 0.8229838658936495799 ) ) ;
#19341=CARTESIAN_POINT ( 'NONE',  ( -339.1964088526558498, -96.52406086224443982, -52.47426709956138069 ) ) ;
#19351=VECTOR ( 'NONE', #43652, 1000.000000000000227 ) ;
#19354=PLANE ( 'NONE',  #11645 ) ;
#19355=DIRECTION ( 'NONE',  ( 0.000000000000000000, 0.8854560256532078011, -0.4647231720437724478 ) ) ;
#19356=CARTESIAN_POINT ( 'NONE',  ( 0.000000000000000000, -71.25809448646064936, -27.41866715058241866 ) ) ;
#19358=CARTESIAN_POINT ( 'NONE',  ( -332.3517673607765914, -63.76276212672765809, 5.609136410542459039 ) ) ;
#19359=EDGE_LOOP ( 'NONE', ( #46236, #5220, #39551, #39953 ) ) ;
#19360=DIRECTION ( 'NONE',  ( 0.000000000000000000, -0.3546048870425235200, 0.9350162426854194964 ) ) ;
#19362=CARTESIAN_POINT ( 'NONE',  ( -332.3517673607765914, -65.82380048139334860, 12.53476669029061519 ) ) ;
#19363=VERTEX_POINT ( 'NONE', #6400 ) ;
#19371=ORIENTED_EDGE ( 'NONE', *, *, #39545, .T. ) ;
#19378=DIRECTION ( 'NONE',  ( -8.718379230999707126E-17, -0.4647231720437755564, -0.8854560256532062468 ) ) ;
#19379=VECTOR ( 'NONE', #43621, 1000.000000000000000 ) ;
#19383=FACE_OUTER_BOUND ( 'NONE', #43841, .T. ) ;
#19388=EDGE_CURVE ( 'NONE', #3747, #34815, #17968, .T. ) ;
#19392=FACE_OUTER_BOUND ( 'NONE', #20321, .T. ) ;
#19401=CARTESIAN_POINT ( 'NONE',  ( -305.0000000000000568, -99.78295912235451226, 55.11353710303931308 ) ) ;
#19403=CARTESIAN_POINT ( 'NONE',  ( -339.1964088526558498, -124.0000000000002700, -59.00000000000002132 ) ) ;
#19404=AXIS2_PLACEMENT_3D ( 'NONE', #371, #9319, #36910 ) ;
#19407=EDGE_CURVE ( 'NONE', #3041, #42991, #10586, .T. ) ;
#19408=DIRECTION ( 'NONE',  ( 0.000000000000000000, 0.000000000000000000, 1.000000000000000000 ) ) ;
#19409=ORIENTED_EDGE ( 'NONE', *, *, #48138, .F. ) ;
#19410=CARTESIAN_POINT ( 'NONE',  ( -336.3521761649654422, -166.6218737817864621, 41.71934804797023588 ) ) ;
#19411=SURFACE_SIDE_STYLE ('',( #18898 ) ) ;
#19412=VERTEX_POINT ( 'NONE', #37673 ) ;
#19418=FACE_OUTER_BOUND ( 'NONE', #28586, .T. ) ;
#19422=VERTEX_POINT ( 'NONE', #22425 ) ;
#19426=EDGE_LOOP ( 'NONE', ( #2304, #13533, #37084, #11584 ) ) ;
#19432=CARTESIAN_POINT ( 'NONE',  ( -339.1964088526558498, -163.6602333390102331, -44.57752413667962088 ) ) ;
#19434=PLANE ( 'NONE',  #49916 ) ;
#19439=ORIENTED_EDGE ( 'NONE', *, *, #30601, .F. ) ;
#19442=ADVANCED_FACE ( 'NONE', ( #30550 ), #25572, .F. ) ;
#19446=ORIENTED_EDGE ( 'NONE', *, *, #30379, .T. ) ;
#19447=VERTEX_POINT ( 'NONE', #14544 ) ;
#19448=AXIS2_PLACEMENT_3D ( 'NONE', #37984, #30605, #2761 ) ;
#19449=ORIENTED_EDGE ( 'NONE', *, *, #15598, .F. ) ;
#19451=CARTESIAN_POINT ( 'NONE',  ( -330.4913330509368166, -138.1050951016783301, 57.16590939599346655 ) ) ;
#19455=ORIENTED_EDGE ( 'NONE', *, *, #8061, .F. ) ;
#19459=ORIENTED_EDGE ( 'NONE', *, *, #28824, .F. ) ;
#19468=DIRECTION ( 'NONE',  ( -0.000000000000000000, 0.7485107481711024136, 0.6631226582407937498 ) ) ;
#19471=EDGE_LOOP ( 'NONE', ( #10042, #48706, #12027, #40518 ) ) ;
#19475=VECTOR ( 'NONE', #3399, 999.9999999999998863 ) ;
#19477=DIRECTION ( 'NONE',  ( -0.000000000000000000, 0.000000000000000000, -1.000000000000000000 ) ) ;
#19478=EDGE_CURVE ( 'NONE', #50728, #5823, #13760, .T. ) ;
#19482=ORIENTED_EDGE ( 'NONE', *, *, #42625, .F. ) ;
#19483=EDGE_CURVE ( 'NONE', #24129, #12564, #30298, .T. ) ;
#19485=CARTESIAN_POINT ( 'NONE',  ( 0.000000000000000000, -96.08133284941780516, -52.24190551353947143 ) ) ;
#19488=DIRECTION ( 'NONE',  ( 0.000000000000000000, 0.8854560256532078011, -0.4647231720437724478 ) ) ;
#19492=EDGE_CURVE ( 'NONE', #33439, #20384, #9817, .T. ) ;
#19494=DIRECTION ( 'NONE',  ( -0.000000000000000000, 0.7485107481711089639, 0.6631226582407863113 ) ) ;
#19496=DIRECTION ( 'NONE',  ( 1.043714542225393539E-14, 0.1205366802553095307, -0.9927088740980556381 ) ) ;
#19502=AXIS2_PLACEMENT_3D ( 'NONE', #27423, #43471, #27685 ) ;
#19503=FACE_OUTER_BOUND ( 'NONE', #5118, .T. ) ;
#19508=DIRECTION ( 'NONE',  ( 1.000000000000000000, -0.000000000000000000, -0.000000000000000000 ) ) ;
#19510=DIRECTION ( 'NONE',  ( -0.000000000000000000, -0.5680647467311485954, 0.8229838658936613482 ) ) ;
#19512=ORIENTED_EDGE ( 'NONE', *, *, #24102, .F. ) ;
#19513=VECTOR ( 'NONE', #20994, 1000.000000000000000 ) ;
#19516=EDGE_CURVE ( 'NONE', #19986, #32415, #31643, .T. ) ;
#19523=LINE ( 'NONE', #43707, #51055 ) ;
#19525=EDGE_CURVE ( 'NONE', #42477, #11058, #51842, .T. ) ;
#19526=ADVANCED_FACE ( 'NONE', ( #35520 ), #31326, .F. ) ;
#19528=DIRECTION ( 'NONE',  ( -1.000000000000000000, 0.000000000000000000, 0.000000000000000000 ) ) ;
#19530=AXIS2_PLACEMENT_3D ( 'NONE', #33298, #29347, #21988 ) ;
#19531=ORIENTED_EDGE ( 'NONE', *, *, #1061, .T. ) ;
#19533=ORIENTED_EDGE ( 'NONE', *, *, #20373, .F. ) ;
#19537=DIRECTION ( 'NONE',  ( 0.000000000000000000, -0.9709418174260519008, 0.2393156642875582940 ) ) ;
#19541=FACE_OUTER_BOUND ( 'NONE', #13907, .T. ) ;
#19543=FACE_OUTER_BOUND ( 'NONE', #22857, .T. ) ;
#19548=DIRECTION ( 'NONE',  ( -1.000000000000000000, 0.000000000000000000, 0.000000000000000000 ) ) ;
#19551=ORIENTED_EDGE ( 'NONE', *, *, #38525, .F. ) ;
#19553=CARTESIAN_POINT ( 'NONE',  ( -332.3517673607765914, -118.8878589706978914, -59.82247199109903590 ) ) ;
#19555=CARTESIAN_POINT ( 'NONE',  ( -336.3521761649654422, -71.64707600775140861, -30.18731974611341684 ) ) ;
#19556=ORIENTED_EDGE ( 'NONE', *, *, #8632, .F. ) ;
#19560=DIRECTION ( 'NONE',  ( 0.000000000000000000, -0.9350162426854107256, 0.3546048870425463906 ) ) ;
#19562=ORIENTED_EDGE ( 'NONE', *, *, #33469, .T. ) ;
#19563=CARTESIAN_POINT ( 'NONE',  ( -339.1964088526558498, -123.0000000000002700, -59.00000000000002132 ) ) ;
#19564=EDGE_CURVE ( 'NONE', #48223, #39946, #2958, .T. ) ;
#19565=VECTOR ( 'NONE', #37698, 1000.000000000000227 ) ;
#19567=CARTESIAN_POINT ( 'NONE',  ( -332.3517673607765914, -123.5000000000000284, 0.000000000000000000 ) ) ;
#19569=ORIENTED_EDGE ( 'NONE', *, *, #11768, .F. ) ;
#19571=DIRECTION ( 'NONE',  ( 0.000000000000000000, 0.000000000000000000, -1.000000000000000000 ) ) ;
#19574=DIRECTION ( 'NONE',  ( -1.000000000000000000, 1.043714542225393381E-14, -1.093232954177749459E-28 ) ) ;
#19577=DIRECTION ( 'NONE',  ( -1.000000000000000000, 0.000000000000000000, 0.000000000000000000 ) ) ;
#19581=LINE ( 'NONE', #48498, #4305 ) ;
#19583=ORIENTED_EDGE ( 'NONE', *, *, #4295, .F. ) ;
#19584=EDGE_LOOP ( 'NONE', ( #26270, #26843, #25435, #1197 ) ) ;
#19586=AXIS2_PLACEMENT_3D ( 'NONE', #9636, #29859, #29343 ) ;
#19587=CARTESIAN_POINT ( 'NONE',  ( -336.3521761649654422, -181.7525362123217292, 9.724760635742144999 ) ) ;
#19588=ORIENTED_EDGE ( 'NONE', *, *, #41392, .F. ) ;
#19591=EDGE_LOOP ( 'NONE', ( #6425, #6465, #15334, #50362 ) ) ;
#19592=CARTESIAN_POINT ( 'NONE',  ( -330.4913330509368166, -130.2355952558269507, -59.62073260661665586 ) ) ;
#19593=FACE_OUTER_BOUND ( 'NONE', #50576, .T. ) ;
#19597=LINE ( 'NONE', #30634, #20223 ) ;
#19598=CARTESIAN_POINT ( 'NONE',  ( -330.4913330509368166, -137.1341532842523918, 57.40522506028099770 ) ) ;
#19602=ADVANCED_FACE ( 'NONE', ( #27651 ), #43157, .F. ) ;
#19603=ORIENTED_EDGE ( 'NONE', *, *, #49912, .F. ) ;
#19610=ORIENTED_EDGE ( 'NONE', *, *, #16722, .T. ) ;
#19615=VECTOR ( 'NONE', #37781, 1000.000000000000000 ) ;
#19616=VERTEX_POINT ( 'NONE', #4001 ) ;
#19619=PRODUCT_DEFINITION ( 'UNKNOWN', '', #29265, #3774 ) ;
#19622=CARTESIAN_POINT ( 'NONE',  ( -339.1964088526558498, -144.8891964568526305, -54.98865587491811624 ) ) ;
#19628=LINE ( 'NONE', #23331, #38836 ) ;
#19629=FACE_OUTER_BOUND ( 'NONE', #8063, .T. ) ;
#19631=CARTESIAN_POINT ( 'NONE',  ( -330.4913330509368166, -75.22798428563987727, -33.92731199008506593 ) ) ;
#19633=CARTESIAN_POINT ( 'NONE',  ( -339.1964088526558498, -175.9742670995610752, 26.97593913775620678 ) ) ;
#19640=PLANE ( 'NONE',  #14826 ) ;
#19643=DIRECTION ( 'NONE',  ( 0.000000000000000000, -0.7485107481710953081, 0.6631226582408016323 ) ) ;
#19644=ORIENTED_EDGE ( 'NONE', *, *, #38414, .T. ) ;
#19645=CARTESIAN_POINT ( 'NONE',  ( -330.4913330509368166, -123.5000000000000284, 0.000000000000000000 ) ) ;
#19657=CARTESIAN_POINT ( 'NONE',  ( -336.3521761649654422, -139.2044816956407089, -56.89493493766761389 ) ) ;
#19661=AXIS2_PLACEMENT_3D ( 'NONE', #11686, #36117, #19571 ) ;
#19662=DIRECTION ( 'NONE',  ( 0.000000000000000000, -0.8229838658936516893, 0.5680647467311625842 ) ) ;
#19666=CARTESIAN_POINT ( 'NONE',  ( -330.4913330509368166, -84.75001853787810546, 44.49369547121489887 ) ) ;
#19667=ORIENTED_EDGE ( 'NONE', *, *, #36862, .T. ) ;
#19676=DIRECTION ( 'NONE',  ( 0.000000000000000000, 7.470875769873448799E-14, -1.000000000000000000 ) ) ;
#19677=CARTESIAN_POINT ( 'NONE',  ( -330.4913330509368166, -96.52406086224436876, -52.47426709956133806 ) ) ;
#19680=DIRECTION ( 'NONE',  ( 1.000000000000000000, 0.000000000000000000, -0.000000000000000000 ) ) ;
#19693=EDGE_LOOP ( 'NONE', ( #25919, #22842, #13098, #31148 ) ) ;
#19694=LINE ( 'NONE', #11566, #3010 ) ;
#19696=VECTOR ( 'NONE', #40250, 1000.000000000000114 ) ;
#19699=VERTEX_POINT ( 'NONE', #44197 ) ;
#19701=VERTEX_POINT ( 'NONE', #16871 ) ;
#19711=EDGE_CURVE ( 'NONE', #47019, #38839, #5308, .T. ) ;
#19716=EDGE_CURVE ( 'NONE', #10327, #18753, #49193, .T. ) ;
#19723=DIRECTION ( 'NONE',  ( 0.000000000000000000, -2.558138885907131360E-13, 1.000000000000000000 ) ) ;
#19724=VERTEX_POINT ( 'NONE', #16621 ) ;
#19725=VECTOR ( 'NONE', #25016, 1000.000000000000114 ) ;
#19730=LINE ( 'NONE', #43905, #1203 ) ;
#19733=CARTESIAN_POINT ( 'NONE',  ( -330.4913330509368166, -176.3931552210899554, 28.32515014536886611 ) ) ;
#19735=LINE ( 'NONE', #8433, #14872 ) ;
#19736=CARTESIAN_POINT ( 'NONE',  ( -332.3517673607765914, -94.18160986457395722, 52.34913561719000796 ) ) ;
#19745=CARTESIAN_POINT ( 'NONE',  ( -339.1964088526558498, -124.0000000000002700, -59.00000000000002132 ) ) ;
#19751=DIRECTION ( 'NONE',  ( -0.000000000000000000, 0.6631226582408039638, 0.7485107481710934207 ) ) ;
#19752=AXIS2_PLACEMENT_3D ( 'NONE', #25434, #25691, #1520 ) ;
#19761=LINE ( 'NONE', #39983, #21556 ) ;
#19762=ADVANCED_FACE ( 'NONE', ( #12907 ), #37083, .T. ) ;
#19763=FACE_OUTER_BOUND ( 'NONE', #17233, .T. ) ;
#19768=VERTEX_POINT ( 'NONE', #8449 ) ;
#19772=CARTESIAN_POINT ( 'NONE',  ( -339.1964088526558498, -108.8949048983213004, -57.16590939599337418 ) ) ;
#19781=LINE ( 'NONE', #11890, #37622 ) ;
#19782=CARTESIAN_POINT ( 'NONE',  ( -332.3517673607765914, -74.01670616005314685, 32.17247266903214609 ) ) ;
#19790=VERTEX_POINT ( 'NONE', #1348 ) ;
#19791=VECTOR ( 'NONE', #40661, 1000.000000000000000 ) ;
#19792=DIRECTION ( 'NONE',  ( 0.000000000000000000, -0.2393156642875482465, 0.9709418174260544543 ) ) ;
#19793=CARTESIAN_POINT ( 'NONE',  ( -336.3521761649654422, -74.01670616005314685, 32.17247266903214609 ) ) ;
#19794=DIRECTION ( 'NONE',  ( 0.000000000000000000, 9.251858538542971828E-16, 1.000000000000000000 ) ) ;
#19795=FACE_OUTER_BOUND ( 'NONE', #10554, .T. ) ;
#19797=ORIENTED_EDGE ( 'NONE', *, *, #17989, .T. ) ;
#19798=DIRECTION ( 'NONE',  ( 1.000000000000000000, -0.000000000000000000, 0.000000000000000000 ) ) ;
#19803=EDGE_LOOP ( 'NONE', ( #21652, #386, #15892, #26197 ) ) ;
#19813=VERTEX_POINT ( 'NONE', #9500 ) ;
#19814=DIRECTION ( 'NONE',  ( 0.000000000000000000, 0.000000000000000000, 1.000000000000000000 ) ) ;
#19823=EDGE_CURVE ( 'NONE', #47279, #11613, #18166, .T. ) ;
#19834=VECTOR ( 'NONE', #12098, 1000.000000000000114 ) ;
#19838=CARTESIAN_POINT ( 'NONE',  ( -339.1964088526558498, -95.63860483659040312, 52.00954392751717847 ) ) ;
#19840=ORIENTED_EDGE ( 'NONE', *, *, #42439, .F. ) ;
#19848=VERTEX_POINT ( 'NONE', #13442 ) ;
#19849=ADVANCED_FACE ( 'NONE', ( #5570 ), #13699, .F. ) ;
#19851=DIRECTION ( 'NONE',  ( -1.000000000000000000, -0.000000000000000000, 0.000000000000000000 ) ) ;
#19853=CARTESIAN_POINT ( 'NONE',  ( -332.3517673607765914, -183.4422309845877805, 2.632288850093980503 ) ) ;
#19856=EDGE_CURVE ( 'NONE', #23381, #41706, #34442, .T. ) ;
#19862=CARTESIAN_POINT ( 'NONE',  ( -305.0000000000000568, -123.5000000000000284, 20.00000000000000355 ) ) ;
#19865=AXIS2_PLACEMENT_3D ( 'NONE', #44985, #25008, #22866 ) ;
#19868=DIRECTION ( 'NONE',  ( 1.000000000000000000, -0.000000000000000000, -0.000000000000000000 ) ) ;
#19870=ORIENTED_EDGE ( 'NONE', *, *, #28707, .T. ) ;
#19881=LINE ( 'NONE', #24097, #31230 ) ;
#19892=VECTOR ( 'NONE', #37634, 1000.000000000000000 ) ;
#19897=EDGE_CURVE ( 'NONE', #10996, #22773, #30494, .T. ) ;
#19899=DIRECTION ( 'NONE',  ( -0.000000000000000000, -0.7485107481711046340, -0.6631226582407911962 ) ) ;
#19900=FACE_OUTER_BOUND ( 'NONE', #10083, .T. ) ;
#19904=VECTOR ( 'NONE', #42992, 1000.000000000000000 ) ;
#19906=LINE ( 'NONE', #40372, #18930 ) ;
#19911=AXIS2_PLACEMENT_3D ( 'NONE', #48954, #595, #4815 ) ;
#19913=VECTOR ( 'NONE', #8964, 1000.000000000000000 ) ;
#19920=CARTESIAN_POINT ( 'NONE',  ( -339.1964088526558498, -71.49045607248213230, 27.86139516340826106 ) ) ;
#19925=VECTOR ( 'NONE', #47754, 1000.000000000000000 ) ;
#19931=DIRECTION ( 'NONE',  ( 0.000000000000000000, -0.8854560256532141294, -0.4647231720437604574 ) ) ;
#19935=DIRECTION ( 'NONE',  ( 0.000000000000000000, 0.000000000000000000, -1.000000000000000000 ) ) ;
#19939=AXIS2_PLACEMENT_3D ( 'NONE', #24204, #32322, #1053 ) ;
#19941=CARTESIAN_POINT ( 'NONE',  ( -339.1964088526558498, -63.87926739338334414, -6.735595255826711814 ) ) ;
#19942=ORIENTED_EDGE ( 'NONE', *, *, #40718, .T. ) ;
#19948=DIRECTION ( 'NONE',  ( -1.000000000000000000, -0.000000000000000000, -0.000000000000000000 ) ) ;
#19949=DIRECTION ( 'NONE',  ( -0.000000000000000000, 0.8854560256532157947, 0.4647231720437573488 ) ) ;
#19953=CARTESIAN_POINT ( 'NONE',  ( -330.4913330509368166, -156.6043281241909995, 48.84008046109159551 ) ) ;
#19955=CARTESIAN_POINT ( 'NONE',  ( -339.1964088526558498, -79.00630452878414189, 38.74998146212082162 ) ) ;
#19957=CARTESIAN_POINT ( 'NONE',  ( -332.3517673607765914, -182.3871109312487420, -4.498567634386014369 ) ) ;
#19967=VECTOR ( 'NONE', #3782, 1000.000000000000000 ) ;
#19968=AXIS2_PLACEMENT_3D ( 'NONE', #25632, #29052, #41663 ) ;
#19973=VERTEX_POINT ( 'NONE', #15250 ) ;
#19974=ORIENTED_EDGE ( 'NONE', *, *, #51010, .F. ) ;
#19980=CARTESIAN_POINT ( 'NONE',  ( -339.1964088526558498, -66.09477493971917283, -13.63415328425296202 ) ) ;
#19986=VERTEX_POINT ( 'NONE', #2639 ) ;
#19995=DIRECTION ( 'NONE',  ( -1.000000000000000000, 0.000000000000000000, -0.000000000000000000 ) ) ;
#19999=DIRECTION ( 'NONE',  ( -1.000000000000000000, -0.000000000000000000, 0.000000000000000000 ) ) ;
#20000=ORIENTED_EDGE ( 'NONE', *, *, #50577, .T. ) ;
#20004=LINE ( 'NONE', #36033, #24943 ) ;
#20005=CARTESIAN_POINT ( 'NONE',  ( 0.000000000000000000, -123.4999999999994174, 59.00000000000002132 ) ) ;
#20009=EDGE_CURVE ( 'NONE', #43701, #7946, #31523, .T. ) ;
#20010=VECTOR ( 'NONE', #46185, 1000.000000000000000 ) ;
#20012=CARTESIAN_POINT ( 'NONE',  ( -336.3521761649654422, -177.7325358280884586, 23.38292116578760726 ) ) ;
#20013=FACE_OUTER_BOUND ( 'NONE', #47919, .T. ) ;
#20014=ORIENTED_EDGE ( 'NONE', *, *, #50938, .T. ) ;
#20020=CARTESIAN_POINT ( 'NONE',  ( -305.0000000000000568, -171.3361784870343740, 36.21739951675979086 ) ) ;
#20021=DIRECTION ( 'NONE',  ( 0.000000000000000000, 0.9927088740980556381, 0.1205366802553095307 ) ) ;
#20027=CARTESIAN_POINT ( 'NONE',  ( -332.3517673607765914, -161.2787550547969033, 46.61293454085098631 ) ) ;
#20029=LINE ( 'NONE', #16096, #10120 ) ;
#20032=DIRECTION ( 'NONE',  ( -0.000000000000000000, -0.5680647467311596976, -0.8229838658936536877 ) ) ;
#20044=ORIENTED_EDGE ( 'NONE', *, *, #5806, .T. ) ;
#20052=ORIENTED_EDGE ( 'NONE', *, *, #8005, .F. ) ;
#20058=CARTESIAN_POINT ( 'NONE',  ( -336.3521761649654422, -66.60506506233235768, -15.70448169564047092 ) ) ;
#20062=CARTESIAN_POINT ( 'NONE',  ( -332.3517673607765914, -80.42027357919624819, -40.34602258462219027 ) ) ;
#20063=ADVANCED_FACE ( 'NONE', ( #39405 ), #10790, .F. ) ;
#20065=CARTESIAN_POINT ( 'NONE',  ( -330.4913330509368166, -68.51134412508180560, -21.38919645685231075 ) ) ;
#20069=ORIENTED_EDGE ( 'NONE', *, *, #16665, .F. ) ;
#20073=VECTOR ( 'NONE', #36445, 1000.000000000000000 ) ;
#20074=ORIENTED_EDGE ( 'NONE', *, *, #43846, .F. ) ;
#20075=CARTESIAN_POINT ( 'NONE',  ( -336.3521761649654422, -166.5797264208035244, 40.34602258462248159 ) ) ;
#20079=ORIENTED_EDGE ( 'NONE', *, *, #27888, .T. ) ;
#20080=EDGE_CURVE ( 'NONE', #46003, #46969, #47579, .T. ) ;
#20081=CARTESIAN_POINT ( 'NONE',  ( -339.1964088526558498, -151.8251501453679850, 52.89315522109039591 ) ) ;
#20083=EDGE_CURVE ( 'NONE', #29431, #40004, #35724, .T. ) ;
#20086=ORIENTED_EDGE ( 'NONE', *, *, #39419, .F. ) ;
#20087=DIRECTION ( 'NONE',  ( 0.000000000000000000, 0.000000000000000000, -1.000000000000000000 ) ) ;
#20088=EDGE_CURVE ( 'NONE', #15690, #22268, #7868, .T. ) ;
#20090=ORIENTED_EDGE ( 'NONE', *, *, #15703, .T. ) ;
#20093=CARTESIAN_POINT ( 'NONE',  ( -336.3521761649654422, -182.3871109312487420, -4.498567634386014369 ) ) ;
#20095=AXIS2_PLACEMENT_3D ( 'NONE', #37858, #33912, #49957 ) ;
#20096=ORIENTED_EDGE ( 'NONE', *, *, #15348, .T. ) ;
#20100=CARTESIAN_POINT ( 'NONE',  ( -336.3521761649654422, -123.5000000000000284, 0.000000000000000000 ) ) ;
#20106=ORIENTED_EDGE ( 'NONE', *, *, #45593, .T. ) ;
#20108=LINE ( 'NONE', #16177, #39023 ) ;
#20110=ORIENTED_EDGE ( 'NONE', *, *, #25910, .T. ) ;
#20114=CARTESIAN_POINT ( 'NONE',  ( -336.3521761649654422, -175.3529239922484351, 30.18731974611377566 ) ) ;
#20115=ORIENTED_EDGE ( 'NONE', *, *, #35337, .T. ) ;
#20118=CARTESIAN_POINT ( 'NONE',  ( -330.4913330509368166, -67.22367097967925531, -20.80804632820203537 ) ) ;
#20121=FACE_BOUND ( 'NONE', #48102, .T. ) ;
#20122=LINE ( 'NONE', #7532, #33931 ) ;
#20127=AXIS2_PLACEMENT_3D ( 'NONE', #26282, #25780, #34436 ) ;
#20128=AXIS2_PLACEMENT_3D ( 'NONE', #21921, #37943, #49788 ) ;
#20132=VERTEX_POINT ( 'NONE', #32036 ) ;
#20133=DIRECTION ( 'NONE',  ( 0.000000000000000000, 1.047444401652940007E-14, 1.000000000000000000 ) ) ;
#20134=ORIENTED_EDGE ( 'NONE', *, *, #41035, .F. ) ;
#20138=DIRECTION ( 'NONE',  ( 0.000000000000000000, 2.361536891963093559E-13, -1.000000000000000000 ) ) ;
#20139=DIRECTION ( 'NONE',  ( 1.000000000000000000, -0.000000000000000000, -0.000000000000000000 ) ) ;
#20151=ADVANCED_FACE ( 'NONE', ( #17079 ), #36241, .F. ) ;
#20152=DIRECTION ( 'NONE',  ( 0.000000000000000000, 2.498001805406602216E-14, -1.000000000000000000 ) ) ;
#20154=ORIENTED_EDGE ( 'NONE', *, *, #1158, .T. ) ;
#20156=FACE_OUTER_BOUND ( 'NONE', #15145, .T. ) ;
#20158=ORIENTED_EDGE ( 'NONE', *, *, #19201, .F. ) ;
#20162=LINE ( 'NONE', #16494, #41377 ) ;
#20170=ORIENTED_EDGE ( 'NONE', *, *, #20205, .F. ) ;
#20178=DIRECTION ( 'NONE',  ( 0.000000000000000000, 0.9709418174260511236, -0.2393156642875615969 ) ) ;
#20181=ADVANCED_FACE ( 'NONE', ( #32567 ), #44920, .F. ) ;
#20183=EDGE_CURVE ( 'NONE', #12564, #16597, #48618, .T. ) ;
#20184=EDGE_CURVE ( 'NONE', #19790, #30079, #12848, .T. ) ;
#20185=CARTESIAN_POINT ( 'NONE',  ( -336.3521761649654422, -125.1322888500942270, -59.00000000000002132 ) ) ;
#20188=DIRECTION ( 'NONE',  ( -1.000000000000000000, 0.000000000000000000, 0.000000000000000000 ) ) ;
#20189=FACE_OUTER_BOUND ( 'NONE', #49598, .T. ) ;
#20194=VERTEX_POINT ( 'NONE', #9189 ) ;
#20196=VECTOR ( 'NONE', #37932, 1000.000000000000000 ) ;
#20199=ORIENTED_EDGE ( 'NONE', *, *, #5861, .F. ) ;
#20203=VERTEX_POINT ( 'NONE', #45982 ) ;
#20204=VECTOR ( 'NONE', #51813, 1000.000000000000114 ) ;
#20205=EDGE_CURVE ( 'NONE', #12928, #35455, #15681, .T. ) ;
#20208=CARTESIAN_POINT ( 'NONE',  ( -332.3517673607765914, -181.7525362123217292, 9.724760635742144999 ) ) ;
#20211=CARTESIAN_POINT ( 'NONE',  ( -305.0000000000000568, -159.7173995167596274, -47.83617848703448772 ) ) ;
#20216=ORIENTED_EDGE ( 'NONE', *, *, #41954, .F. ) ;
#20222=VERTEX_POINT ( 'NONE', #30189 ) ;
#20223=VECTOR ( 'NONE', #47214, 1000.000000000000000 ) ;
#20226=CARTESIAN_POINT ( 'NONE',  ( -336.3521761649654422, -123.5000000000000284, 0.000000000000000000 ) ) ;
#20232=CARTESIAN_POINT ( 'NONE',  ( -330.4913330509368166, -130.1153096980153236, -58.63009191191284941 ) ) ;
#20236=AXIS2_PLACEMENT_3D ( 'NONE', #39978, #44467, #36054 ) ;
#20238=LINE ( 'NONE', #49420, #24351 ) ;
#20240=AXIS2_PLACEMENT_3D ( 'NONE', #44859, #12787, #40908 ) ;
#20241=VERTEX_POINT ( 'NONE', #37289 ) ;
#20247=ADVANCED_FACE ( 'NONE', ( #29918 ), #33861, .F. ) ;
#20249=DIRECTION ( 'NONE',  ( 0.000000000000000000, 0.000000000000000000, -1.000000000000000000 ) ) ;
#20254=CARTESIAN_POINT ( 'NONE',  ( -330.4913330509368166, -122.9999999999994600, 59.00000000000002132 ) ) ;
#20255=ORIENTED_EDGE ( 'NONE', *, *, #37180, .F. ) ;
#20257=ORIENTED_EDGE ( 'NONE', *, *, #27458, .F. ) ;
#20259=DIRECTION ( 'NONE',  ( 0.000000000000000000, 0.9350162426854132791, -0.3546048870425396182 ) ) ;
#20262=ORIENTED_EDGE ( 'NONE', *, *, #15398, .T. ) ;
#20265=ORIENTED_EDGE ( 'NONE', *, *, #24896, .F. ) ;
#20266=EDGE_CURVE ( 'NONE', #29097, #47521, #29397, .T. ) ;
#20269=AXIS2_PLACEMENT_3D ( 'NONE', #51151, #23523, #7237 ) ;
#20270=DIRECTION ( 'NONE',  ( 0.000000000000000000, 0.6631226582407911962, -0.7485107481711046340 ) ) ;
#20271=EDGE_LOOP ( 'NONE', ( #2434, #9735, #14189, #29535 ) ) ;
#20273=VECTOR ( 'NONE', #7296, 1000.000000000000000 ) ;
#20274=CARTESIAN_POINT ( 'NONE',  ( -332.3517673607765914, -141.9604555052315220, 56.09938080879057765 ) ) ;
#20276=ORIENTED_EDGE ( 'NONE', *, *, #41565, .T. ) ;
#20277=DIRECTION ( 'NONE',  ( 0.000000000000000000, -0.5680647467311625842, -0.8229838658936516893 ) ) ;
#20279=CARTESIAN_POINT ( 'NONE',  ( -332.3517673607765914, -123.5000000000000284, 0.000000000000000000 ) ) ;
#20283=CARTESIAN_POINT ( 'NONE',  ( -305.0000000000000568, -123.5000000000000284, 0.000000000000000000 ) ) ;
#20284=VECTOR ( 'NONE', #10093, 1000.000000000000000 ) ;
#20288=CARTESIAN_POINT ( 'NONE',  ( -330.4913330509368166, -156.6043281241909995, 48.84008046109159551 ) ) ;
#20291=ORIENTED_EDGE ( 'NONE', *, *, #34453, .T. ) ;
#20296=ORIENTED_EDGE ( 'NONE', *, *, #30880, .T. ) ;
#20300=DIRECTION ( 'NONE',  ( 0.000000000000000000, 0.9709418174260493473, -0.2393156642875685913 ) ) ;
#20303=VERTEX_POINT ( 'NONE', #42256 ) ;
#20307=DIRECTION ( 'NONE',  ( 1.000000000000000000, -0.000000000000000000, -0.000000000000000000 ) ) ;
#20309=ORIENTED_EDGE ( 'NONE', *, *, #46629, .T. ) ;
#20310=DIRECTION ( 'NONE',  ( 0.000000000000000000, 0.5680647467311510379, -0.8229838658936596829 ) ) ;
#20314=FACE_OUTER_BOUND ( 'NONE', #51064, .T. ) ;
#20318=ORIENTED_EDGE ( 'NONE', *, *, #34681, .T. ) ;
#20321=EDGE_LOOP ( 'NONE', ( #26987, #6254, #44380, #36730 ) ) ;
#20327=DIRECTION ( 'NONE',  ( 0.000000000000000000, 0.000000000000000000, 1.000000000000000000 ) ) ;
#20336=CARTESIAN_POINT ( 'NONE',  ( -332.3517673607765914, -146.8829211657874794, -54.23253582808848705 ) ) ;
#20337=EDGE_CURVE ( 'NONE', #30471, #23668, #45706, .T. ) ;
#20341=DIRECTION ( 'NONE',  ( 0.000000000000000000, 0.000000000000000000, 1.000000000000000000 ) ) ;
#20351=CARTESIAN_POINT ( 'NONE',  ( -305.0000000000000568, -88.08538291676191534, 48.43351006119235080 ) ) ;
#20355=DIRECTION ( 'NONE',  ( -0.000000000000000000, 0.9927088740980538617, -0.1205366802553232974 ) ) ;
#20359=LINE ( 'NONE', #44020, #32679 ) ;
#20362=EDGE_LOOP ( 'NONE', ( #21992, #479, #32768, #40921 ) ) ;
#20363=DIRECTION ( 'NONE',  ( -0.000000000000000000, 0.4647231720437664526, -0.8854560256532110207 ) ) ;
#20370=LINE ( 'NONE', #36395, #38329 ) ;
#20371=ORIENTED_EDGE ( 'NONE', *, *, #17325, .F. ) ;
#20372=ORIENTED_EDGE ( 'NONE', *, *, #19856, .F. ) ;
#20373=EDGE_CURVE ( 'NONE', #4643, #7784, #42786, .T. ) ;
#20375=LINE ( 'NONE', #40593, #10638 ) ;
#20377=ADVANCED_FACE ( 'NONE', ( #2586 ), #3094, .T. ) ;
#20379=FACE_BOUND ( 'NONE', #21645, .T. ) ;
#20380=FACE_OUTER_BOUND ( 'NONE', #24912, .T. ) ;
#20381=VECTOR ( 'NONE', #51195, 1000.000000000000227 ) ;
#20383=VECTOR ( 'NONE', #38200, 1000.000000000000000 ) ;
#20384=VERTEX_POINT ( 'NONE', #27003 ) ;
#20386=ORIENTED_EDGE ( 'NONE', *, *, #25036, .T. ) ;
#20387=DIRECTION ( 'NONE',  ( 0.000000000000000000, -1.000000000000000000, 1.047444401652940007E-14 ) ) ;
#20391=CARTESIAN_POINT ( 'NONE',  ( -339.1964088526558498, -74.65991953890876687, -33.10432812419148263 ) ) ;
#20395=LINE ( 'NONE', #32748, #14958 ) ;
#20398=VECTOR ( 'NONE', #36727, 1000.000000000000000 ) ;
#20399=EDGE_LOOP ( 'NONE', ( #5801, #16696, #29404, #40173 ) ) ;
#20405=CARTESIAN_POINT ( 'NONE',  ( -330.4913330509368166, -150.9396941197155968, -53.35787839313373837 ) ) ;
#20407=AXIS2_PLACEMENT_3D ( 'NONE', #19645, #32773, #40636 ) ;
#20414=LINE ( 'NONE', #39854, #4632 ) ;
#20419=EDGE_CURVE ( 'NONE', #6309, #42116, #27525, .T. ) ;
#20421=ORIENTED_EDGE ( 'NONE', *, *, #34319, .F. ) ;
#20426=ORIENTED_EDGE ( 'NONE', *, *, #38834, .T. ) ;
#20436=EDGE_LOOP ( 'NONE', ( #17559, #16411, #25534, #38462 ) ) ;
#20438=PLANE ( 'NONE',  #23626 ) ;
#20440=ADVANCED_FACE ( 'NONE', ( #22568 ), #19640, .F. ) ;
#20447=ORIENTED_EDGE ( 'NONE', *, *, #49090, .F. ) ;
#20450=FACE_OUTER_BOUND ( 'NONE', #34550, .T. ) ;
#20460=VERTEX_POINT ( 'NONE', #38582 ) ;
#20462=FACE_OUTER_BOUND ( 'NONE', #17983, .T. ) ;
#20464=DIRECTION ( 'NONE',  ( 0.000000000000000000, -0.7485107481711089639, -0.6631226582407863113 ) ) ;
#20466=CARTESIAN_POINT ( 'NONE',  ( -332.3517673607765914, -170.5607375887735770, 35.68215131113770155 ) ) ;
#20470=CARTESIAN_POINT ( 'NONE',  ( -336.3521761649654422, -97.52665284734005979, -53.00046796564681983 ) ) ;
#20473=VERTEX_POINT ( 'NONE', #19137 ) ;
#20479=ORIENTED_EDGE ( 'NONE', *, *, #23099, .T. ) ;
#20480=EDGE_CURVE ( 'NONE', #15659, #24073, #5442, .T. ) ;
#20485=PLANE ( 'NONE',  #164 ) ;
#20490=CARTESIAN_POINT ( 'NONE',  ( -305.0000000000000568, -180.1590281025188460, -19.74220186498920881 ) ) ;
#20495=EDGE_CURVE ( 'NONE', #43377, #38337, #29335, .T. ) ;
#20497=ORIENTED_EDGE ( 'NONE', *, *, #10394, .F. ) ;
#20498=EDGE_CURVE ( 'NONE', #16257, #1746, #5954, .T. ) ;
#20500=CARTESIAN_POINT ( 'NONE',  ( -330.0000000000000568, -123.5000000000000284, 0.000000000000000000 ) ) ;
#20502=VECTOR ( 'NONE', #42940, 1000.000000000000114 ) ;
#20514=CARTESIAN_POINT ( 'NONE',  ( -332.3517673607765914, -65.92952926200918284, -16.90091414705545247 ) ) ;
#20516=DIRECTION ( 'NONE',  ( 0.000000000000000000, -4.093947403305264743E-14, 1.000000000000000000 ) ) ;
#20517=DIRECTION ( 'NONE',  ( -1.000000000000000000, 0.000000000000000000, 0.000000000000000000 ) ) ;
#20519=ORIENTED_EDGE ( 'NONE', *, *, #28564, .F. ) ;
#20523=EDGE_LOOP ( 'NONE', ( #6587, #38406, #7001, #11367 ) ) ;
#20525=VECTOR ( 'NONE', #50212, 1000.000000000000000 ) ;
#20532=ADVANCED_FACE ( 'NONE', ( #40022 ), #868, .F. ) ;
#20533=ORIENTED_EDGE ( 'NONE', *, *, #46852, .T. ) ;
#20540=DIRECTION ( 'NONE',  ( -1.000000000000000000, 0.000000000000000000, 0.000000000000000000 ) ) ;
#20542=DIRECTION ( 'NONE',  ( 0.000000000000000000, 0.8854560256532157947, 0.4647231720437573488 ) ) ;
#20549=LINE ( 'NONE', #47654, #19696 ) ;
#20550=CARTESIAN_POINT ( 'NONE',  ( -339.1964088526558498, -108.8949048983204051, 57.16590939599314680 ) ) ;
#20553=DIRECTION ( 'NONE',  ( 0.000000000000000000, 0.8229838658936556861, -0.5680647467311569221 ) ) ;
#20555=VERTEX_POINT ( 'NONE', #48713 ) ;
#20557=VECTOR ( 'NONE', #50414, 1000.000000000000000 ) ;
#20562=VECTOR ( 'NONE', #9820, 1000.000000000000000 ) ;
#20563=EDGE_CURVE ( 'NONE', #28063, #21855, #87, .T. ) ;
#20565=DIRECTION ( 'NONE',  ( -1.000000000000000000, 0.000000000000000000, 0.000000000000000000 ) ) ;
#20569=EDGE_CURVE ( 'NONE', #41226, #4457, #48969, .T. ) ;
#20570=PLANE ( 'NONE',  #9032 ) ;
#20572=DIRECTION ( 'NONE',  ( -1.000000000000000000, 0.000000000000000000, 0.000000000000000000 ) ) ;
#20574=AXIS2_PLACEMENT_3D ( 'NONE', #33324, #13355, #17048 ) ;
#20576=AXIS2_PLACEMENT_3D ( 'NONE', #51108, #15095, #15336 ) ;
#20577=CARTESIAN_POINT ( 'NONE',  ( -330.4913330509368166, -182.5000000000000568, -0.4999999999999551470 ) ) ;
#20578=EDGE_LOOP ( 'NONE', ( #30293, #12222, #48590, #23589 ) ) ;
#20584=DIRECTION ( 'NONE',  ( 1.000000000000000000, -0.000000000000000000, -0.000000000000000000 ) ) ;
#20589=FACE_OUTER_BOUND ( 'NONE', #34322, .T. ) ;
#20592=DIRECTION ( 'NONE',  ( -0.000000000000000000, -3.491481338843133355E-15, -1.000000000000000000 ) ) ;
#20594=DIRECTION ( 'NONE',  ( 0.000000000000000000, 0.8229838658936613482, 0.5680647467311485954 ) ) ;
#20595=LINE ( 'NONE', #32686, #34804 ) ;
#20597=CARTESIAN_POINT ( 'NONE',  ( -336.3521761649654422, -69.26746417191145611, -23.38292116578723068 ) ) ;
#20598=EDGE_LOOP ( 'NONE', ( #28259, #40226, #40660, #6371 ) ) ;
#20599=AXIS2_PLACEMENT_3D ( 'NONE', #298, #16619, #12641 ) ;
#20601=ORIENTED_EDGE ( 'NONE', *, *, #10110, .F. ) ;
#20603=VECTOR ( 'NONE', #33668, 1000.000000000000114 ) ;
#20605=CARTESIAN_POINT ( 'NONE',  ( -336.3521761649654422, -101.0520950768976149, 54.58714071513087873 ) ) ;
#20606=CARTESIAN_POINT ( 'NONE',  ( -336.3521761649654422, -123.5000000000000284, 0.000000000000000000 ) ) ;
#20607=ADVANCED_FACE ( 'NONE', ( #20314 ), #12164, .F. ) ;
#20609=PLANE ( 'NONE',  #36659 ) ;
#20613=APPLICATION_CONTEXT ( 'automotive_design' ) ;
#20622=AXIS2_PLACEMENT_3D ( 'NONE', #19485, #31313, #40228 ) ;
#20626=CARTESIAN_POINT ( 'NONE',  ( -332.3517673607765914, -113.6616659693417546, 59.18789727217204444 ) ) ;
#20628=ORIENTED_EDGE ( 'NONE', *, *, #36626, .T. ) ;
#20629=FACE_OUTER_BOUND ( 'NONE', #40839, .T. ) ;
#20635=EDGE_CURVE ( 'NONE', #32740, #16500, #44502, .T. ) ;
#20641=VECTOR ( 'NONE', #32026, 1000.000000000000000 ) ;
#20642=CYLINDRICAL_SURFACE ( 'NONE', #11096, 60.00000000000000000 ) ;
#20650=ORIENTED_EDGE ( 'NONE', *, *, #21491, .F. ) ;
#20651=LINE ( 'NONE', #32743, #19925 ) ;
#20652=AXIS2_PLACEMENT_3D ( 'NONE', #6190, #27635, #31053 ) ;
#20654=AXIS2_PLACEMENT_3D ( 'NONE', #41608, #29524, #21661 ) ;
#20655=CARTESIAN_POINT ( 'NONE',  ( -336.3521761649654422, -93.75055682584159911, 51.01861988938794923 ) ) ;
#20659=CIRCLE ( 'NONE', #8924, 60.00000000000000000 ) ;
#20665=DIRECTION ( 'NONE',  ( -8.718379230999703429E-17, 0.4647231720437695057, 0.8854560256532093554 ) ) ;
#20666=LINE ( 'NONE', #45824, #20562 ) ;
#20670=EDGE_CURVE ( 'NONE', #4146, #153, #21637, .T. ) ;
#20671=ADVANCED_FACE ( 'NONE', ( #45301 ), #5873, .F. ) ;
#20673=LINE ( 'NONE', #37220, #34741 ) ;
#20680=AXIS2_PLACEMENT_3D ( 'NONE', #15709, #31725, #23830 ) ;
#20684=CARTESIAN_POINT ( 'NONE',  ( -330.4913330509368166, -157.9941932480469973, -49.09328500076553325 ) ) ;
#20685=ORIENTED_EDGE ( 'NONE', *, *, #1920, .T. ) ;
#20691=VECTOR ( 'NONE', #9493, 1000.000000000000114 ) ;
#20697=AXIS2_PLACEMENT_3D ( 'NONE', #11441, #7260, #8030 ) ;
#20700=EDGE_LOOP ( 'NONE', ( #17347, #40717, #26088, #15082 ) ) ;
#20704=ORIENTED_EDGE ( 'NONE', *, *, #15359, .T. ) ;
#20706=DIRECTION ( 'NONE',  ( 0.000000000000000000, 0.000000000000000000, 1.000000000000000000 ) ) ;
#20712=DIRECTION ( 'NONE',  ( 1.043714542225393223E-14, 0.9350162426854181641, 0.3546048870425267951 ) ) ;
#20714=VECTOR ( 'NONE', #892, 1000.000000000000114 ) ;
#20716=VECTOR ( 'NONE', #19004, 1000.000000000000000 ) ;
#20718=ORIENTED_EDGE ( 'NONE', *, *, #23285, .F. ) ;
#20719=CARTESIAN_POINT ( 'NONE',  ( -336.3521761649654422, -86.34605966037949543, -45.90766452162698386 ) ) ;
#20727=DIRECTION ( 'NONE',  ( 0.000000000000000000, 0.000000000000000000, 1.000000000000000000 ) ) ;
#20732=PLANE ( 'NONE',  #18960 ) ;
#20735=CARTESIAN_POINT ( 'NONE',  ( -330.4913330509368166, -68.15673923803930734, -20.45418021416698551 ) ) ;
#20744=DIRECTION ( 'NONE',  ( -1.000000000000000000, 0.000000000000000000, 0.000000000000000000 ) ) ;
#20745=EDGE_CURVE ( 'NONE', #27746, #28072, #30029, .T. ) ;
#20746=AXIS2_PLACEMENT_3D ( 'NONE', #23379, #19948, #19676 ) ;
#20748=ORIENTED_EDGE ( 'NONE', *, *, #30958, .F. ) ;
#20753=DIRECTION ( 'NONE',  ( -1.000000000000000000, -0.000000000000000000, -0.000000000000000000 ) ) ;
#20755=ORIENTED_EDGE ( 'NONE', *, *, #18783, .T. ) ;
#20756=ORIENTED_EDGE ( 'NONE', *, *, #38752, .T. ) ;
#20758=DIRECTION ( 'NONE',  ( -8.718379230999704661E-17, 0.1205366802553164696, -0.9927088740980548609 ) ) ;
#20760=DIRECTION ( 'NONE',  ( 0.000000000000000000, -0.9350162426854121689, 0.3546048870425426713 ) ) ;
#20761=DIRECTION ( 'NONE',  ( 0.000000000000000000, 0.000000000000000000, -1.000000000000000000 ) ) ;
#20763=VECTOR ( 'NONE', #38595, 1000.000000000000000 ) ;
#20765=CARTESIAN_POINT ( 'NONE',  ( -332.3517673607765914, -82.40546666720629787, 42.41660376256258047 ) ) ;
#20766=CARTESIAN_POINT ( 'NONE',  ( -336.3521761649654422, -76.43926241122620979, -35.68215131113738181 ) ) ;
#20770=AXIS2_PLACEMENT_3D ( 'NONE', #2009, #6746, #18049 ) ;
#20775=VECTOR ( 'NONE', #26329, 999.9999999999998863 ) ;
#20777=CARTESIAN_POINT ( 'NONE',  ( -336.3521761649654422, -132.2320517616439020, -58.37307289257706344 ) ) ;
#20779=CARTESIAN_POINT ( 'NONE',  ( -332.3517673607765914, -64.50000000000000000, -2.632288850093980503 ) ) ;
#20782=VERTEX_POINT ( 'NONE', #5348 ) ;
#20787=EDGE_CURVE ( 'NONE', #26369, #7333, #17949, .T. ) ;
#20797=VECTOR ( 'NONE', #39131, 1000.000000000000000 ) ;
#20803=EDGE_CURVE ( 'NONE', #41684, #37940, #26077, .T. ) ;
#20804=AXIS2_PLACEMENT_3D ( 'NONE', #23485, #47915, #40261 ) ;
#20809=EDGE_CURVE ( 'NONE', #36354, #42318, #11604, .T. ) ;
#20812=VECTOR ( 'NONE', #10102, 1000.000000000000000 ) ;
#20814=DIRECTION ( 'NONE',  ( 0.000000000000000000, 1.137978600240785454E-13, -1.000000000000000000 ) ) ;
#20822=DIRECTION ( 'NONE',  ( -1.000000000000000000, -0.000000000000000000, 0.000000000000000000 ) ) ;
#20826=ORIENTED_EDGE ( 'NONE', *, *, #17395, .T. ) ;
#20828=EDGE_CURVE ( 'NONE', #2008, #32067, #3209, .T. ) ;
#20833=ORIENTED_EDGE ( 'NONE', *, *, #14398, .T. ) ;
#20840=VERTEX_POINT ( 'NONE', #34731 ) ;
#20843=DIRECTION ( 'NONE',  ( -0.000000000000000000, 0.2393156642875685636, 0.9709418174260492362 ) ) ;
#20844=AXIS2_PLACEMENT_3D ( 'NONE', #15599, #7461, #39249 ) ;
#20846=ORIENTED_EDGE ( 'NONE', *, *, #12497, .F. ) ;
#20848=ORIENTED_EDGE ( 'NONE', *, *, #38818, .T. ) ;
#20854=ADVANCED_FACE ( 'NONE', ( #51057 ), #11327, .F. ) ;
#20857=CARTESIAN_POINT ( 'NONE',  ( -305.0000000000000568, -94.18160986457394301, 52.34913561719000086 ) ) ;
#20858=EDGE_CURVE ( 'NONE', #32415, #32067, #27364, .T. ) ;
#20859=VECTOR ( 'NONE', #37845, 1000.000000000000000 ) ;
#20863=LINE ( 'NONE', #16917, #19111 ) ;
#20867=PLANE ( 'NONE',  #34127 ) ;
#20868=LINE ( 'NONE', #32928, #39619 ) ;
#20869=ORIENTED_EDGE ( 'NONE', *, *, #8092, .T. ) ;
#20885=ADVANCED_FACE ( 'NONE', ( #50527 ), #30533, .F. ) ;
#20891=ORIENTED_EDGE ( 'NONE', *, *, #48741, .T. ) ;
#20892=LINE ( 'NONE', #16425, #42961 ) ;
#20893=EDGE_LOOP ( 'NONE', ( #43238, #21173, #29441, #40801 ) ) ;
#20894=VERTEX_POINT ( 'NONE', #19733 ) ;
#20895=VECTOR ( 'NONE', #1506, 1000.000000000000114 ) ;
#20902=ADVANCED_FACE ( 'NONE', ( #39690 ), #48658, .F. ) ;
#20907=CARTESIAN_POINT ( 'NONE',  ( -336.3521761649654422, -64.50000000000000000, -2.632288850093980503 ) ) ;
#20911=ORIENTED_EDGE ( 'NONE', *, *, #26485, .T. ) ;
#20919=DIRECTION ( 'NONE',  ( -8.718379230999707126E-17, -0.3546048870425426158, -0.9350162426854121689 ) ) ;
#20925=DIRECTION ( 'NONE',  ( 0.000000000000000000, 0.2393156642875582940, 0.9709418174260519008 ) ) ;
#20926=VERTEX_POINT ( 'NONE', #33583 ) ;
#20930=CARTESIAN_POINT ( 'NONE',  ( -305.0000000000000568, -157.1712093821534211, -49.66134974749665076 ) ) ;
#20938=DIRECTION ( 'NONE',  ( 0.000000000000000000, 0.000000000000000000, -1.000000000000000000 ) ) ;
#20940=LINE ( 'NONE', #5427, #22797 ) ;
#20947=EDGE_CURVE ( 'NONE', #18306, #38201, #44702, .T. ) ;
#20948=DIRECTION ( 'NONE',  ( -1.000000000000000000, 0.000000000000000000, -0.000000000000000000 ) ) ;
#20953=EDGE_LOOP ( 'NONE', ( #51803, #7350, #50953, #6039 ) ) ;
#20954=VECTOR ( 'NONE', #49432, 1000.000000000000000 ) ;
#20961=DIRECTION ( 'NONE',  ( 1.000000000000000000, 0.000000000000000000, -0.000000000000000000 ) ) ;
#20962=CARTESIAN_POINT ( 'NONE',  ( -330.4913330509368166, -66.33409060400670398, -14.60509510167892522 ) ) ;
#20964=DIRECTION ( 'NONE',  ( -0.000000000000000000, 0.6631226582407937498, -0.7485107481711024136 ) ) ;
#20965=ORIENTED_EDGE ( 'NONE', *, *, #13147, .T. ) ;
#20968=ORIENTED_EDGE ( 'NONE', *, *, #40786, .T. ) ;
#20969=CARTESIAN_POINT ( 'NONE',  ( -339.1964088526558498, -63.99980407363865709, -7.728304129924767452 ) ) ;
#20978=ORIENTED_EDGE ( 'NONE', *, *, #10032, .T. ) ;
#20983=VECTOR ( 'NONE', #6102, 1000.000000000000000 ) ;
#20985=VERTEX_POINT ( 'NONE', #20514 ) ;
#20986=CARTESIAN_POINT ( 'NONE',  ( -305.0000000000000568, -123.5000000000000284, -15.24495751795539000 ) ) ;
#20994=DIRECTION ( 'NONE',  ( -0.000000000000000000, -1.000000000000000000, -0.000000000000000000 ) ) ;
#20997=LINE ( 'NONE', #4703, #21330 ) ;
#21002=FACE_OUTER_BOUND ( 'NONE', #45959, .T. ) ;
#21003=CARTESIAN_POINT ( 'NONE',  ( -336.3521761649654422, -123.5000000000000284, 0.000000000000000000 ) ) ;
#21004=PLANE ( 'NONE',  #16452 ) ;
#21007=DIRECTION ( 'NONE',  ( -1.000000000000000000, -0.000000000000000000, 0.000000000000000000 ) ) ;
#21013=ORIENTED_EDGE ( 'NONE', *, *, #18329, .T. ) ;
#21014=ORIENTED_EDGE ( 'NONE', *, *, #7609, .F. ) ;
#21015=LINE ( 'NONE', #8928, #3279 ) ;
#21018=DIRECTION ( 'NONE',  ( 0.000000000000000000, 0.7485107481711089639, 0.6631226582407863113 ) ) ;
#21019=PLANE ( 'NONE',  #41326 ) ;
#21020=ORIENTED_EDGE ( 'NONE', *, *, #26594, .F. ) ;
#21021=EDGE_CURVE ( 'NONE', #45109, #25441, #20004, .T. ) ;
#21022=PLANE ( 'NONE',  #9850 ) ;
#21024=ORIENTED_EDGE ( 'NONE', *, *, #16276, .F. ) ;
#21025=DIRECTION ( 'NONE',  ( 1.000000000000000000, 0.000000000000000000, -0.000000000000000000 ) ) ;
#21028=CARTESIAN_POINT ( 'NONE',  ( -339.1964088526558498, -180.6659093959934523, -14.60509510167853264 ) ) ;
#21031=EDGE_CURVE ( 'NONE', #18239, #19986, #21498, .T. ) ;
#21033=VECTOR ( 'NONE', #50266, 1000.000000000000114 ) ;
#21035=CARTESIAN_POINT ( 'NONE',  ( -305.0000000000000568, -89.00580675195338642, -49.09328500076576773 ) ) ;
#21036=CARTESIAN_POINT ( 'NONE',  ( -332.3517673607765914, -170.5607375887735770, 35.68215131113770155 ) ) ;
#21038=PLANE ( 'NONE',  #19939 ) ;
#21039=EDGE_LOOP ( 'NONE', ( #28969, #21769, #34678, #51684 ) ) ;
#21040=EDGE_CURVE ( 'NONE', #30980, #18160, #29630, .T. ) ;
#21046=LINE ( 'NONE', #45488, #49379 ) ;
#21048=FACE_OUTER_BOUND ( 'NONE', #23405, .T. ) ;
#21050=LINE ( 'NONE', #8436, #28229 ) ;
#21054=ORIENTED_EDGE ( 'NONE', *, *, #29542, .T. ) ;
#21057=LINE ( 'NONE', #37074, #20691 ) ;
#21059=DIRECTION ( 'NONE',  ( 0.000000000000000000, 0.000000000000000000, -1.000000000000000000 ) ) ;
#21061=LINE ( 'NONE', #37618, #31509 ) ;
#21063=ORIENTED_EDGE ( 'NONE', *, *, #47132, .F. ) ;
#21064=CARTESIAN_POINT ( 'NONE',  ( -330.4913330509368166, -116.8846903019842927, 58.63009191191280678 ) ) ;
#21068=DIRECTION ( 'NONE',  ( 0.000000000000000000, 0.000000000000000000, -1.000000000000000000 ) ) ;
#21069=VECTOR ( 'NONE', #51516, 1000.000000000000000 ) ;
#21075=ORIENTED_EDGE ( 'NONE', *, *, #42366, .T. ) ;
#21076=EDGE_CURVE ( 'NONE', #25441, #45944, #29893, .T. ) ;
#21080=EDGE_LOOP ( 'NONE', ( #11624, #557, #13994, #20318 ) ) ;
#21093=EDGE_LOOP ( 'NONE', ( #27486, #26593, #35867, #4856 ) ) ;
#21095=CARTESIAN_POINT ( 'NONE',  ( -330.4913330509368166, -123.5000000000000284, 0.000000000000000000 ) ) ;
#21096=VERTEX_POINT ( 'NONE', #30404 ) ;
#21098=VECTOR ( 'NONE', #13568, 1000.000000000000000 ) ;
#21099=EDGE_CURVE ( 'NONE', #51399, #6061, #33389, .T. ) ;
#21100=VERTEX_POINT ( 'NONE', #25697 ) ;
#21108=DIRECTION ( 'NONE',  ( 0.000000000000000000, 0.3546048870425331789, -0.9350162426854158326 ) ) ;
#21113=EDGE_LOOP ( 'NONE', ( #1883, #41213, #15041, #2978 ) ) ;
#21114=LINE ( 'NONE', #49518, #37639 ) ;
#21116=CARTESIAN_POINT ( 'NONE',  ( -332.3517673607765914, -111.9361751271348879, -57.91551518289410438 ) ) ;
#21118=CARTESIAN_POINT ( 'NONE',  ( -336.3521761649654422, -123.5000000000000284, 0.000000000000000000 ) ) ;
#21119=ORIENTED_EDGE ( 'NONE', *, *, #9979, .T. ) ;
#21128=CARTESIAN_POINT ( 'NONE',  ( -490.0000000000001137, -78.50000000000002842, 14.36509618646847386 ) ) ;
#21129=EDGE_LOOP ( 'NONE', ( #36242, #22610, #4389, #31920 ) ) ;
#21133=FACE_OUTER_BOUND ( 'NONE', #38186, .T. ) ;
#21134=ORIENTED_EDGE ( 'NONE', *, *, #20670, .T. ) ;
#21135=VECTOR ( 'NONE', #15557, 1000.000000000000114 ) ;
#21136=EDGE_CURVE ( 'NONE', #30781, #23810, #6245, .T. ) ;
#21142=ADVANCED_FACE ( 'NONE', ( #50152 ), #46205, .F. ) ;
#21143=VECTOR ( 'NONE', #51793, 1000.000000000000000 ) ;
#21144=LINE ( 'NONE', #17990, #20383 ) ;
#21148=EDGE_CURVE ( 'NONE', #33963, #37409, #2562, .T. ) ;
#21150=CARTESIAN_POINT ( 'NONE',  ( -336.3521761649654422, -182.3871109312487420, -4.498567634386014369 ) ) ;
#21152=ADVANCED_FACE ( 'NONE', ( #41726 ), #10433, .F. ) ;
#21153=CARTESIAN_POINT ( 'NONE',  ( -336.3521761649654422, -174.3267994849386184, -31.88473700876087591 ) ) ;
#21158=EDGE_CURVE ( 'NONE', #33644, #6394, #40907, .T. ) ;
#21160=CARTESIAN_POINT ( 'NONE',  ( -339.1964088526558498, -162.2499814621209850, 44.49369547121574442 ) ) ;
#21165=FACE_BOUND ( 'NONE', #14338, .T. ) ;
#21167=EDGE_LOOP ( 'NONE', ( #45745, #7157, #11770, #44814 ) ) ;
#21173=ORIENTED_EDGE ( 'NONE', *, *, #49768, .F. ) ;
#21176=CARTESIAN_POINT ( 'NONE',  ( -330.4913330509368166, -68.51134412508150717, 21.38919645685156112 ) ) ;
#21178=CARTESIAN_POINT ( 'NONE',  ( -330.4913330509368166, -90.39567187580871632, -48.84008046109136814 ) ) ;
#21182=DIRECTION ( 'NONE',  ( 0.000000000000000000, -2.611337072503753781E-13, -1.000000000000000000 ) ) ;
#21187=PLANE ( 'NONE',  #31292 ) ;
#21191=CARTESIAN_POINT ( 'NONE',  ( -336.3521761649654422, -159.1821513111375452, -47.06073758877369073 ) ) ;
#21195=FACE_OUTER_BOUND ( 'NONE', #20362, .T. ) ;
#21196=VECTOR ( 'NONE', #23653, 1000.000000000000000 ) ;
#21197=AXIS2_PLACEMENT_3D ( 'NONE', #41085, #28466, #12177 ) ;
#21198=CARTESIAN_POINT ( 'NONE',  ( -336.3521761649654422, -178.0871407151310279, 22.44790492310219676 ) ) ;
#21201=VECTOR ( 'NONE', #4642, 1000.000000000000114 ) ;
#21202=VECTOR ( 'NONE', #35222, 1000.000000000000000 ) ;
#21203=DIRECTION ( 'NONE',  ( -0.000000000000000000, 0.8229838658936634577, 0.5680647467311457088 ) ) ;
#21206=ADVANCED_FACE ( 'NONE', ( #24096 ), #47484, .F. ) ;
#21208=EDGE_CURVE ( 'NONE', #16640, #49884, #43272, .T. ) ;
#21226=ADVANCED_FACE ( 'NONE', ( #27505 ), #39829, .T. ) ;
#21229=CARTESIAN_POINT ( 'NONE',  ( -305.0000000000000568, -84.08827740916061089, 45.24064679492014562 ) ) ;
#21238=CARTESIAN_POINT ( 'NONE',  ( -330.4913330509368166, -173.1613497474970416, -33.67120938215288817 ) ) ;
#21241=VECTOR ( 'NONE', #7173, 1000.000000000000000 ) ;
#21253=VERTEX_POINT ( 'NONE', #3857 ) ;
#21254=FACE_OUTER_BOUND ( 'NONE', #11121, .T. ) ;
#21255=CARTESIAN_POINT ( 'NONE',  ( -336.3521761649654422, -111.9361751271348879, -57.91551518289410438 ) ) ;
#21256=CARTESIAN_POINT ( 'NONE',  ( -332.3517673607765914, -70.49953203435293858, 25.97334715265942151 ) ) ;
#21258=ORIENTED_EDGE ( 'NONE', *, *, #47450, .F. ) ;
#21263=LINE ( 'NONE', #31582, #13620 ) ;
#21264=CARTESIAN_POINT ( 'NONE',  ( -339.1964088526558498, -172.3400804610915600, -33.10432812419107051 ) ) ;
#21266=VECTOR ( 'NONE', #8727, 1000.000000000000000 ) ;
#21269=CARTESIAN_POINT ( 'NONE',  ( -170.0000000000000284, -123.5000000000000284, -15.24495751795539000 ) ) ;
#21272=ADVANCED_FACE ( 'NONE', ( #31711 ), #47755, .F. ) ;
#21276=DIRECTION ( 'NONE',  ( -1.000000000000000000, 3.701062773504747805E-15, -9.758900497077197755E-15 ) ) ;
#21278=FACE_OUTER_BOUND ( 'NONE', #13026, .T. ) ;
#21284=DIRECTION ( 'NONE',  ( 0.000000000000000000, -0.1205366802553095307, 0.9927088740980556381 ) ) ;
#21285=PLANE ( 'NONE',  #29843 ) ;
#21286=VERTEX_POINT ( 'NONE', #43787 ) ;
#21295=LINE ( 'NONE', #20777, #9795 ) ;
#21297=CARTESIAN_POINT ( 'NONE',  ( -339.1964088526558498, -138.1050951016783301, 57.16590939599346655 ) ) ;
#21300=PLANE ( 'NONE',  #23955 ) ;
#21303=PLANE ( 'NONE',  #23279 ) ;
#21305=EDGE_CURVE ( 'NONE', #7980, #10791, #17517, .T. ) ;
#21313=DIRECTION ( 'NONE',  ( 1.000000000000000000, -0.000000000000000000, -0.000000000000000000 ) ) ;
#21319=PLANE ( 'NONE',  #52001 ) ;
#21321=VERTEX_POINT ( 'NONE', #28779 ) ;
#21325=CARTESIAN_POINT ( 'NONE',  ( -332.3517673607765914, -140.1754235130667610, -56.65561927338005432 ) ) ;
#21330=VECTOR ( 'NONE', #49383, 1000.000000000000000 ) ;
#21334=VECTOR ( 'NONE', #37216, 1000.000000000000114 ) ;
#21342=CARTESIAN_POINT ( 'NONE',  ( -339.1964088526558498, -71.49045607248213230, 27.86139516340826106 ) ) ;
#21347=ORIENTED_EDGE ( 'NONE', *, *, #24352, .T. ) ;
#21360=CARTESIAN_POINT ( 'NONE',  ( -332.3517673607765914, -70.49953203435293858, 25.97334715265942151 ) ) ;
#21361=VERTEX_POINT ( 'NONE', #21176 ) ;
#21365=DIRECTION ( 'NONE',  ( -8.718379230999705894E-17, 0.9350162426854158326, 0.3546048870425331789 ) ) ;
#21376=FACE_BOUND ( 'NONE', #40266, .T. ) ;
#21377=VECTOR ( 'NONE', #40018, 1000.000000000000000 ) ;
#21378=CARTESIAN_POINT ( 'NONE',  ( -330.4913330509368166, -64.86990808808705822, 6.615309698014281814 ) ) ;
#21379=VERTEX_POINT ( 'NONE', #40346 ) ;
#21388=EDGE_CURVE ( 'NONE', #13133, #45030, #4366, .T. ) ;
#21403=CARTESIAN_POINT ( 'NONE',  ( -365.0000000000001137, -78.50000000000002842, 0.000000000000000000 ) ) ;
#21407=AXIS2_PLACEMENT_3D ( 'NONE', #18132, #42037, #5540 ) ;
#21412=DIRECTION ( 'NONE',  ( -0.000000000000000000, -0.2393156642875615969, -0.9709418174260511236 ) ) ;
#21414=LINE ( 'NONE', #49286, #48387 ) ;
#21428=AXIS2_PLACEMENT_3D ( 'NONE', #37402, #49519, #26614 ) ;
#21430=DIRECTION ( 'NONE',  ( 1.000000000000000000, -0.000000000000000000, -0.000000000000000000 ) ) ;
#21432=VECTOR ( 'NONE', #4521, 1000.000000000000000 ) ;
#21434=CARTESIAN_POINT ( 'NONE',  ( -332.3517673607765914, -172.9832938399466684, -32.17247266903247294 ) ) ;
#21438=VERTEX_POINT ( 'NONE', #45111 ) ;
#21440=ORIENTED_EDGE ( 'NONE', *, *, #966, .T. ) ;
#21442=EDGE_CURVE ( 'NONE', #8221, #36738, #31684, .T. ) ;
#21443=EDGE_CURVE ( 'NONE', #3275, #18160, #48472, .T. ) ;
#21444=ORIENTED_EDGE ( 'NONE', *, *, #21021, .F. ) ;
#21445=CARTESIAN_POINT ( 'NONE',  ( -336.3521761649654422, -132.2320517616439020, -58.37307289257706344 ) ) ;
#21446=ADVANCED_FACE ( 'NONE', ( #37459 ), #13813, .F. ) ;
#21448=DIRECTION ( 'NONE',  ( -0.000000000000000000, -0.3546048870425300148, 0.9350162426854169428 ) ) ;
#21456=AXIS2_PLACEMENT_3D ( 'NONE', #37842, #10492, #1837 ) ;
#21457=DIRECTION ( 'NONE',  ( 0.000000000000000000, 0.9709418174260519008, -0.2393156642875582940 ) ) ;
#21458=ADVANCED_FACE ( 'NONE', ( #50085 ), #1977, .T. ) ;
#21459=CARTESIAN_POINT ( 'NONE',  ( -339.1964088526558498, -64.86990808808717190, -6.615309698015097162 ) ) ;
#21461=CARTESIAN_POINT ( 'NONE',  ( -330.4913330509368166, -124.0000000000001990, -59.00000000000002132 ) ) ;
#21462=ORIENTED_EDGE ( 'NONE', *, *, #35816, .T. ) ;
#21464=DIRECTION ( 'NONE',  ( 1.043714542225393381E-14, 0.2393156642875449158, -0.9709418174260553425 ) ) ;
#21465=VERTEX_POINT ( 'NONE', #18019 ) ;
#21470=DIRECTION ( 'NONE',  ( 0.000000000000000000, 0.8229838658936516893, -0.5680647467311626952 ) ) ;
#21471=VECTOR ( 'NONE', #45705, 1000.000000000000000 ) ;
#21472=DIRECTION ( 'NONE',  ( 0.000000000000000000, 1.029269262412905585E-13, 1.000000000000000000 ) ) ;
#21474=VERTEX_POINT ( 'NONE', #45878 ) ;
#21477=EDGE_CURVE ( 'NONE', #41880, #26860, #45625, .T. ) ;
#21481=FACE_BOUND ( 'NONE', #44839, .T. ) ;
#21483=VERTEX_POINT ( 'NONE', #30596 ) ;
#21490=CARTESIAN_POINT ( 'NONE',  ( -339.1964088526558498, -71.49045607248255862, -27.86139516340906397 ) ) ;
#21491=EDGE_CURVE ( 'NONE', #9298, #13843, #34543, .T. ) ;
#21492=CARTESIAN_POINT ( 'NONE',  ( -336.3521761649654422, -93.75055682584159911, 51.01861988938794923 ) ) ;
#21493=ORIENTED_EDGE ( 'NONE', *, *, #50436, .T. ) ;
#21496=VERTEX_POINT ( 'NONE', #26142 ) ;
#21498=LINE ( 'NONE', #16598, #35845 ) ;
#21504=EDGE_CURVE ( 'NONE', #46459, #10671, #29829, .T. ) ;
#21505=CARTESIAN_POINT ( 'NONE',  ( -330.4913330509368166, -84.08827740916061089, 45.24064679492014562 ) ) ;
#21511=DIRECTION ( 'NONE',  ( 0.000000000000000000, -0.5680647467311457088, 0.8229838658936633466 ) ) ;
#21513=DIRECTION ( 'NONE',  ( -0.000000000000000000, 0.000000000000000000, 1.000000000000000000 ) ) ;
#21516=CARTESIAN_POINT ( 'NONE',  ( -332.3517673607765914, -148.5878911270064009, 53.46519113769075204 ) ) ;
#21519=DIRECTION ( 'NONE',  ( -0.000000000000000000, 0.000000000000000000, -1.000000000000000000 ) ) ;
#21523=CARTESIAN_POINT ( 'NONE',  ( -330.4913330509368166, -122.9999999999994600, 59.99791663049642665 ) ) ;
#21527=PLANE ( 'NONE',  #3004 ) ;
#21530=CIRCLE ( 'NONE', #51033, 60.00000000000000000 ) ;
#21534=VECTOR ( 'NONE', #25202, 1000.000000000000000 ) ;
#21538=ORIENTED_EDGE ( 'NONE', *, *, #41068, .T. ) ;
#21539=ORIENTED_EDGE ( 'NONE', *, *, #16737, .T. ) ;
#21542=ADVANCED_FACE ( 'NONE', ( #18529 ), #38740, .F. ) ;
#21546=DIRECTION ( 'NONE',  ( 0.000000000000000000, -0.1205366802553095168, 0.9927088740980556381 ) ) ;
#21556=VECTOR ( 'NONE', #11872, 1000.000000000000114 ) ;
#21565=DIRECTION ( 'NONE',  ( 0.000000000000000000, 0.5680647467311626952, 0.8229838658936516893 ) ) ;
#21572=ORIENTED_EDGE ( 'NONE', *, *, #31926, .F. ) ;
#21574=VERTEX_POINT ( 'NONE', #15120 ) ;
#21575=ADVANCED_FACE ( 'NONE', ( #47172 ), #26921, .F. ) ;
#21576=EDGE_CURVE ( 'NONE', #24073, #22978, #3784, .T. ) ;
#21583=AXIS2_PLACEMENT_3D ( 'NONE', #13942, #37846, #6059 ) ;
#21584=LINE ( 'NONE', #41525, #24864 ) ;
#21587=ORIENTED_EDGE ( 'NONE', *, *, #42140, .T. ) ;
#21588=CARTESIAN_POINT ( 'NONE',  ( -339.1964088526558498, -123.5000000000000284, 0.000000000000000000 ) ) ;
#21590=DIRECTION ( 'NONE',  ( -1.000000000000000000, 0.000000000000000000, 0.000000000000000000 ) ) ;
#21592=LINE ( 'NONE', #1345, #50628 ) ;
#21596=VECTOR ( 'NONE', #13164, 1000.000000000000114 ) ;
#21598=DIRECTION ( 'NONE',  ( 1.000000000000000000, -0.000000000000000000, -0.000000000000000000 ) ) ;
#21603=DIRECTION ( 'NONE',  ( 0.000000000000000000, 0.000000000000000000, 1.000000000000000000 ) ) ;
#21604=EDGE_CURVE ( 'NONE', #45638, #38775, #22989, .T. ) ;
#21605=CARTESIAN_POINT ( 'NONE',  ( -339.1964088526558498, -162.2499814621216672, -44.49369547121515467 ) ) ;
#21608=CARTESIAN_POINT ( 'NONE',  ( -339.1964088526558498, -64.86990808808717190, -6.615309698015097162 ) ) ;
#21610=DIRECTION ( 'NONE',  ( -1.000000000000000000, 9.241633304753506654E-15, -4.850383327712056395E-15 ) ) ;
#21613=EDGE_LOOP ( 'NONE', ( #44530, #10354 ) ) ;
#21615=VECTOR ( 'NONE', #32346, 1000.000000000000000 ) ;
#21618=VERTEX_POINT ( 'NONE', #15893 ) ;
#21619=EDGE_LOOP ( 'NONE', ( #3307, #41768, #37014, #7341 ) ) ;
#21627=AXIS2_PLACEMENT_3D ( 'NONE', #10640, #31376, #11399 ) ;
#21628=FACE_OUTER_BOUND ( 'NONE', #45314, .T. ) ;
#21632=ORIENTED_EDGE ( 'NONE', *, *, #28169, .T. ) ;
#21633=CARTESIAN_POINT ( 'NONE',  ( -305.0000000000000568, -123.5000000000000284, 0.000000000000000000 ) ) ;
#21635=EDGE_LOOP ( 'NONE', ( #12802, #13358, #10052, #34232 ) ) ;
#21636=EDGE_CURVE ( 'NONE', #2495, #29872, #21530, .T. ) ;
#21637=LINE ( 'NONE', #2163, #10643 ) ;
#21639=DIRECTION ( 'NONE',  ( -0.000000000000000000, -0.1205366802553268363, -0.9927088740980534176 ) ) ;
#21644=CARTESIAN_POINT ( 'NONE',  ( -305.0000000000000568, -100.7053649598255163, 55.50139289590170222 ) ) ;
#21645=EDGE_LOOP ( 'NONE', ( #40581, #24722, #3828, #47625 ) ) ;
#21650=FACE_OUTER_BOUND ( 'NONE', #45905, .T. ) ;
#21652=ORIENTED_EDGE ( 'NONE', *, *, #51528, .T. ) ;
#21654=VERTEX_POINT ( 'NONE', #11920 ) ;
#21657=DIRECTION ( 'NONE',  ( 0.000000000000000000, 1.535808517398133130E-13, 1.000000000000000000 ) ) ;
#21660=EDGE_CURVE ( 'NONE', #42791, #20194, #15626, .T. ) ;
#21661=DIRECTION ( 'NONE',  ( 0.000000000000000000, 0.000000000000000000, 1.000000000000000000 ) ) ;
#21663=DIRECTION ( 'NONE',  ( -1.000000000000000000, 0.000000000000000000, 0.000000000000000000 ) ) ;
#21664=DIRECTION ( 'NONE',  ( 0.000000000000000000, -1.082467449009527627E-13, 1.000000000000000000 ) ) ;
#21669=CARTESIAN_POINT ( 'NONE',  ( -339.1964088526558498, -157.4273119900853146, -48.27201571435997352 ) ) ;
#21670=LINE ( 'NONE', #2468, #48017 ) ;
#21671=ORIENTED_EDGE ( 'NONE', *, *, #26631, .T. ) ;
#21672=AXIS2_PLACEMENT_3D ( 'NONE', #28175, #35548, #325 ) ;
#21673=ORIENTED_EDGE ( 'NONE', *, *, #46092, .T. ) ;
#21675=CARTESIAN_POINT ( 'NONE',  ( -330.4913330509368166, -130.1153096980145563, 58.63009191191294178 ) ) ;
#21677=ORIENTED_EDGE ( 'NONE', *, *, #29077, .T. ) ;
#21682=ADVANCED_FACE ( 'NONE', ( #47941 ), #35326, .F. ) ;
#21683=DIRECTION ( 'NONE',  ( -1.000000000000000000, 0.000000000000000000, -0.000000000000000000 ) ) ;
#21688=AXIS2_PLACEMENT_3D ( 'NONE', #37008, #1003, #17059 ) ;
#21689=EDGE_CURVE ( 'NONE', #36746, #41934, #48377, .T. ) ;
#21690=CARTESIAN_POINT ( 'NONE',  ( -305.0000000000000568, -139.4384828369889249, -57.84431488793872944 ) ) ;
#21691=CARTESIAN_POINT ( 'NONE',  ( -339.1964088526558498, -84.75001853787809125, 44.49369547121489887 ) ) ;
#21692=CARTESIAN_POINT ( 'NONE',  ( -365.0000000000001137, -168.5000000000000284, -10.00000000000000711 ) ) ;
#21694=EDGE_LOOP ( 'NONE', ( #46447, #3738, #36168, #22025 ) ) ;
#21695=UNCERTAINTY_MEASURE_WITH_UNIT (LENGTH_MEASURE( 1.000000000000000082E-05 ), #7587, 'distance_accuracy_value', 'NONE');
#21697=EDGE_CURVE ( 'NONE', #45030, #11192, #43731, .T. ) ;
#21701=ORIENTED_EDGE ( 'NONE', *, *, #31999, .T. ) ;
#21705=AXIS2_PLACEMENT_3D ( 'NONE', #47540, #19662, #24389 ) ;
#21711=CARTESIAN_POINT ( 'NONE',  ( -339.1964088526558498, -66.33409060400650503, 14.60509510167813474 ) ) ;
#21712=EDGE_LOOP ( 'NONE', ( #48221, #25139, #18968, #48989 ) ) ;
#21717=VERTEX_POINT ( 'NONE', #7487 ) ;
#21736=ORIENTED_EDGE ( 'NONE', *, *, #10218, .F. ) ;
#21738=EDGE_CURVE ( 'NONE', #8223, #38711, #38999, .T. ) ;
#21739=EDGE_CURVE ( 'NONE', #6345, #43598, #47694, .T. ) ;
#21742=VERTEX_POINT ( 'NONE', #11674 ) ;
#21747=CARTESIAN_POINT ( 'NONE',  ( -339.1964088526558498, -116.8846903019842927, 58.63009191191280678 ) ) ;
#21748=ADVANCED_FACE ( 'NONE', ( #35075 ), #7734, .F. ) ;
#21751=ORIENTED_EDGE ( 'NONE', *, *, #24518, .T. ) ;
#21755=CARTESIAN_POINT ( 'NONE',  ( -332.3517673607765914, -111.9361751271348879, -57.91551518289410438 ) ) ;
#21762=ORIENTED_EDGE ( 'NONE', *, *, #16978, .T. ) ;
#21769=ORIENTED_EDGE ( 'NONE', *, *, #37150, .T. ) ;
#21772=ORIENTED_EDGE ( 'NONE', *, *, #46229, .T. ) ;
#21777=DIRECTION ( 'NONE',  ( 0.000000000000000000, -0.3546048870425267951, 0.9350162426854181641 ) ) ;
#21783=CARTESIAN_POINT ( 'NONE',  ( -305.0000000000000568, -73.83865025250295844, 33.67120938215276738 ) ) ;
#21785=FACE_OUTER_BOUND ( 'NONE', #38620, .T. ) ;
#21789=EDGE_CURVE ( 'NONE', #1606, #1505, #17342, .T. ) ;
#21796=ORIENTED_EDGE ( 'NONE', *, *, #27189, .F. ) ;
#21798=ADVANCED_FACE ( 'NONE', ( #13238 ), #48978, .F. ) ;
#21806=ADVANCED_FACE ( 'NONE', ( #36623 ), #20867, .F. ) ;
#21820=CARTESIAN_POINT ( 'NONE',  ( -330.4913330509368166, -109.8658467157464571, 57.40522506028071348 ) ) ;
#21825=FACE_OUTER_BOUND ( 'NONE', #15209, .T. ) ;
#21828=FACE_OUTER_BOUND ( 'NONE', #41723, .T. ) ;
#21830=CARTESIAN_POINT ( 'NONE',  ( -336.3521761649654422, -64.61288906875131488, 4.498567634385603142 ) ) ;
#21833=CARTESIAN_POINT ( 'NONE',  ( -336.3521761649654422, -65.82380048139334860, 12.53476669029061519 ) ) ;
#21834=DIRECTION ( 'NONE',  ( -0.000000000000000000, -0.8854560256532110207, -0.4647231720437664526 ) ) ;
#21837=ORIENTED_EDGE ( 'NONE', *, *, #47808, .T. ) ;
#21850=LINE ( 'NONE', #37861, #35524 ) ;
#21855=VERTEX_POINT ( 'NONE', #41592 ) ;
#21857=CARTESIAN_POINT ( 'NONE',  ( -305.0000000000000568, -63.87926739338334414, -6.735595255826709149 ) ) ;
#21861=LINE ( 'NONE', #13452, #6982 ) ;
#21863=CARTESIAN_POINT ( 'NONE',  ( -305.0000000000000568, -175.3529239922484351, 30.18731974611377211 ) ) ;
#21865=ORIENTED_EDGE ( 'NONE', *, *, #29796, .F. ) ;
#21866=ORIENTED_EDGE ( 'NONE', *, *, #35795, .T. ) ;
#21867=EDGE_CURVE ( 'NONE', #36669, #39834, #45815, .T. ) ;
#21868=ADVANCED_FACE ( 'NONE', ( #50284 ), #46088, .F. ) ;
#21873=CARTESIAN_POINT ( 'NONE',  ( -339.1964088526558498, -130.1153096980153236, -58.63009191191284941 ) ) ;
#21874=CARTESIAN_POINT ( 'NONE',  ( -332.3517673607765914, -182.5000000000000568, 2.632288850093980503 ) ) ;
#21877=ORIENTED_EDGE ( 'NONE', *, *, #3949, .F. ) ;
#21881=EDGE_LOOP ( 'NONE', ( #5092, #16942, #24345, #49814 ) ) ;
#21882=DIRECTION ( 'NONE',  ( 1.000000000000000000, 0.000000000000000000, 0.000000000000000000 ) ) ;
#21883=CARTESIAN_POINT ( 'NONE',  ( -339.1964088526558498, -137.1341532842531876, -57.40522506028080585 ) ) ;
#21884=CARTESIAN_POINT ( 'NONE',  ( -339.1964088526558498, -167.3305728129748786, -39.49849221029221269 ) ) ;
#21886=AXIS2_PLACEMENT_3D ( 'NONE', #2289, #13337, #29350 ) ;
#21889=DIRECTION ( 'NONE',  ( 1.000000000000000000, -4.952603889763928634E-17, 7.175085443855162194E-17 ) ) ;
#21895=ORIENTED_EDGE ( 'NONE', *, *, #34549, .T. ) ;
#21897=PLANE ( 'NONE',  #3843 ) ;
#21899=ORIENTED_EDGE ( 'NONE', *, *, #40701, .F. ) ;
#21900=LINE ( 'NONE', #46338, #34976 ) ;
#21903=CARTESIAN_POINT ( 'NONE',  ( -339.1964088526558498, -175.5095439275177398, -27.86139516340860212 ) ) ;
#21909=DIRECTION ( 'NONE',  ( 0.000000000000000000, -0.000000000000000000, 1.000000000000000000 ) ) ;
#21910=DIRECTION ( 'NONE',  ( -0.000000000000000000, 0.8229838658936613482, 0.5680647467311485954 ) ) ;
#21911=DIRECTION ( 'NONE',  ( -1.000000000000000000, -0.000000000000000000, -0.000000000000000000 ) ) ;
#21916=DIRECTION ( 'NONE',  ( 0.000000000000000000, 1.595945597898662527E-14, -1.000000000000000000 ) ) ;
#21918=CARTESIAN_POINT ( 'NONE',  ( -330.4913330509368166, -70.60684477890994515, -28.32515014536850018 ) ) ;
#21921=CARTESIAN_POINT ( 'NONE',  ( -336.3521761649654422, -123.5000000000000284, 0.000000000000000000 ) ) ;
#21924=VERTEX_POINT ( 'NONE', #13490 ) ;
#21926=CARTESIAN_POINT ( 'NONE',  ( -330.4913330509368166, -162.2499814621210419, 44.49369547121568758 ) ) ;
#21929=VERTEX_POINT ( 'NONE', #29509 ) ;
#21930=PLANE ( 'NONE',  #19158 ) ;
#21932=AXIS2_PLACEMENT_3D ( 'NONE', #1351, #17662, #2121 ) ;
#21933=DIRECTION ( 'NONE',  ( 0.000000000000000000, 0.9927088740980538617, -0.1205366802553232974 ) ) ;
#21943=LINE ( 'NONE', #2233, #7893 ) ;
#21945=VECTOR ( 'NONE', #12469, 999.9999999999998863 ) ;
#21948=EDGE_LOOP ( 'NONE', ( #45106, #28006, #34121, #20154 ) ) ;
#21955=ORIENTED_EDGE ( 'NONE', *, *, #12180, .F. ) ;
#21958=ORIENTED_EDGE ( 'NONE', *, *, #24543, .T. ) ;
#21960=CARTESIAN_POINT ( 'NONE',  ( -339.1964088526558498, -123.5000000000000284, 0.000000000000000000 ) ) ;
#21961=EDGE_CURVE ( 'NONE', #5935, #43387, #21900, .T. ) ;
#21965=FACE_OUTER_BOUND ( 'NONE', #41252, .T. ) ;
#21969=CARTESIAN_POINT ( 'NONE',  ( -339.1964088526558498, -144.8891964568526305, -54.98865587491811624 ) ) ;
#21970=CIRCLE ( 'NONE', #35388, 60.00000000000000000 ) ;
#21973=DIRECTION ( 'NONE',  ( -1.000000000000000000, 0.000000000000000000, 0.000000000000000000 ) ) ;
#21974=VERTEX_POINT ( 'NONE', #37397 ) ;
#21978=DIRECTION ( 'NONE',  ( -1.000000000000000000, -0.000000000000000000, -0.000000000000000000 ) ) ;
#21980=ORIENTED_EDGE ( 'NONE', *, *, #37215, .F. ) ;
#21985=EDGE_CURVE ( 'NONE', #39885, #44797, #23195, .T. ) ;
#21986=AXIS2_PLACEMENT_3D ( 'NONE', #21999, #50640, #30389 ) ;
#21988=DIRECTION ( 'NONE',  ( 0.000000000000000000, 0.8229838658936536877, -0.5680647467311596976 ) ) ;
#21992=ORIENTED_EDGE ( 'NONE', *, *, #51366, .T. ) ;
#21999=CARTESIAN_POINT ( 'NONE',  ( -332.3517673607765914, -67.40061919120938683, 18.46045550523129819 ) ) ;
#22004=VECTOR ( 'NONE', #25475, 1000.000000000000000 ) ;
#22008=ORIENTED_EDGE ( 'NONE', *, *, #35392, .T. ) ;
#22009=ORIENTED_EDGE ( 'NONE', *, *, #31274, .F. ) ;
#22015=ORIENTED_EDGE ( 'NONE', *, *, #10116, .F. ) ;
#22017=ORIENTED_EDGE ( 'NONE', *, *, #16737, .F. ) ;
#22021=LINE ( 'NONE', #38569, #18673 ) ;
#22023=DIRECTION ( 'NONE',  ( 0.000000000000000000, 1.047444401652940007E-14, 1.000000000000000000 ) ) ;
#22025=ORIENTED_EDGE ( 'NONE', *, *, #17351, .F. ) ;
#22028=EDGE_CURVE ( 'NONE', #41304, #31069, #18988, .T. ) ;
#22030=DIRECTION ( 'NONE',  ( 0.000000000000000000, 5.851800525628429686E-14, -1.000000000000000000 ) ) ;
#22033=DIRECTION ( 'NONE',  ( 0.000000000000000000, 0.000000000000000000, -1.000000000000000000 ) ) ;
#22036=ORIENTED_EDGE ( 'NONE', *, *, #46192, .T. ) ;
#22039=CIRCLE ( 'NONE', #2715, 60.00000000000000000 ) ;
#22048=EDGE_CURVE ( 'NONE', #50461, #37855, #3716, .T. ) ;
#22052=LINE ( 'NONE', #6031, #43425 ) ;
#22056=LINE ( 'NONE', #37825, #35729 ) ;
#22059=VECTOR ( 'NONE', #26372, 1000.000000000000000 ) ;
#22060=VECTOR ( 'NONE', #45322, 1000.000000000000000 ) ;
#22063=CIRCLE ( 'NONE', #13665, 60.00000000000000000 ) ;
#22069=ORIENTED_EDGE ( 'NONE', *, *, #5882, .T. ) ;
#22075=LINE ( 'NONE', #38094, #39269 ) ;
#22085=ORIENTED_EDGE ( 'NONE', *, *, #15654, .T. ) ;
#22087=DIRECTION ( 'NONE',  ( -1.000000000000000000, -1.036104688092336522E-14, -1.258058860540498485E-15 ) ) ;
#22088=DIRECTION ( 'NONE',  ( 0.000000000000000000, -1.595945597898662527E-14, -1.000000000000000000 ) ) ;
#22099=VECTOR ( 'NONE', #19090, 1000.000000000000114 ) ;
#22105=LINE ( 'NONE', #5842, #35719 ) ;
#22109=DIRECTION ( 'NONE',  ( 1.000000000000000000, -0.000000000000000000, -0.000000000000000000 ) ) ;
#22110=AXIS2_PLACEMENT_3D ( 'NONE', #9129, #13324, #34066 ) ;
#22113=FACE_OUTER_BOUND ( 'NONE', #32570, .T. ) ;
#22115=CARTESIAN_POINT ( 'NONE',  ( -339.1964088526558498, -167.9936954712150339, 38.74998146212178796 ) ) ;
#22123=CIRCLE ( 'NONE', #28815, 60.00000000000000000 ) ;
#22125=DIRECTION ( 'NONE',  ( -0.000000000000000000, 0.000000000000000000, 1.000000000000000000 ) ) ;
#22127=ORIENTED_EDGE ( 'NONE', *, *, #17032, .F. ) ;
#22129=FACE_OUTER_BOUND ( 'NONE', #44830, .T. ) ;
#22131=CARTESIAN_POINT ( 'NONE',  ( -330.4913330509368166, -123.5000000000000284, 0.000000000000000000 ) ) ;
#22134=ADVANCED_FACE ( 'NONE', ( #27999 ), #8542, .F. ) ;
#22136=CARTESIAN_POINT ( 'NONE',  ( -330.4913330509368166, -109.8658467157472813, -57.40522506028090532 ) ) ;
#22139=EDGE_LOOP ( 'NONE', ( #18042, #5450, #44860, #51674 ) ) ;
#22142=ORIENTED_EDGE ( 'NONE', *, *, #29275, .F. ) ;
#22145=DIRECTION ( 'NONE',  ( 0.000000000000000000, 1.047444401652940007E-14, 1.000000000000000000 ) ) ;
#22146=CARTESIAN_POINT ( 'NONE',  ( -332.3517673607765914, -153.2494431741581025, -51.01861988938816950 ) ) ;
#22151=DIRECTION ( 'NONE',  ( -0.000000000000000000, 0.000000000000000000, -1.000000000000000000 ) ) ;
#22152=ORIENTED_EDGE ( 'NONE', *, *, #30859, .T. ) ;
#22154=VECTOR ( 'NONE', #1278, 1000.000000000000000 ) ;
#22158=FACE_BOUND ( 'NONE', #11153, .T. ) ;
#22159=DIRECTION ( 'NONE',  ( -0.000000000000000000, 0.8229838658936556861, -0.5680647467311569221 ) ) ;
#22162=DIRECTION ( 'NONE',  ( 1.000000000000000000, 0.000000000000000000, 0.000000000000000000 ) ) ;
#22165=LINE ( 'NONE', #34250, #31221 ) ;
#22166=ORIENTED_EDGE ( 'NONE', *, *, #39755, .T. ) ;
#22168=CARTESIAN_POINT ( 'NONE',  ( -339.1964088526558498, -79.00630452878473875, -38.74998146212148953 ) ) ;
#22171=VERTEX_POINT ( 'NONE', #19862 ) ;
#22173=ORIENTED_EDGE ( 'NONE', *, *, #37212, .T. ) ;
#22174=EDGE_CURVE ( 'NONE', #44157, #13761, #20375, .T. ) ;
#22176=DIRECTION ( 'NONE',  ( 0.000000000000000000, 0.000000000000000000, -1.000000000000000000 ) ) ;
#22178=EDGE_LOOP ( 'NONE', ( #47527, #44610, #23792, #47960 ) ) ;
#22181=DIRECTION ( 'NONE',  ( 0.000000000000000000, 0.6631226582408017434, 0.7485107481710954191 ) ) ;
#22183=DIRECTION ( 'NONE',  ( -1.000000000000000000, -0.000000000000000000, 0.000000000000000000 ) ) ;
#22187=CARTESIAN_POINT ( 'NONE',  ( -339.1964088526558498, -75.22798428563942252, 33.92731199008440512 ) ) ;
#22188=DIRECTION ( 'NONE',  ( -8.718379230999709592E-17, 0.8854560256532079121, -0.4647231720437725033 ) ) ;
#22193=VERTEX_POINT ( 'NONE', #51944 ) ;
#22194=VERTEX_POINT ( 'NONE', #20118 ) ;
#22197=DIRECTION ( 'NONE',  ( -0.000000000000000000, -0.1205366802553233113, -0.9927088740980538617 ) ) ;
#22205=CARTESIAN_POINT ( 'NONE',  ( -332.3517673607765914, -148.5878911270064009, 53.46519113769075204 ) ) ;
#22208=DIRECTION ( 'NONE',  ( -0.000000000000000000, -0.5680647467311596976, -0.8229838658936536877 ) ) ;
#22209=CARTESIAN_POINT ( 'NONE',  ( -339.1964088526558498, -162.9984922102927385, -43.83057281297435992 ) ) ;
#22213=EDGE_LOOP ( 'NONE', ( #34980, #49303, #33127, #5156 ) ) ;
#22223=DIRECTION ( 'NONE',  ( 0.000000000000000000, 0.9709418174260526779, 0.2393156642875547968 ) ) ;
#22225=LINE ( 'NONE', #2265, #22368 ) ;
#22226=AXIS2_PLACEMENT_3D ( 'NONE', #45984, #48680, #12650 ) ;
#22227=CARTESIAN_POINT ( 'NONE',  ( -332.3517673607765914, -110.9652333097088217, -57.67619951860654481 ) ) ;
#22238=DIRECTION ( 'NONE',  ( -1.000000000000000000, 0.000000000000000000, 0.000000000000000000 ) ) ;
#22239=DIRECTION ( 'NONE',  ( 0.000000000000000000, -0.8854560256532044704, 0.4647231720437789981 ) ) ;
#22240=ORIENTED_EDGE ( 'NONE', *, *, #47190, .F. ) ;
#22243=CARTESIAN_POINT ( 'NONE',  ( -305.0000000000000568, -123.5000000000000284, 0.000000000000000000 ) ) ;
#22244=VERTEX_POINT ( 'NONE', #5925 ) ;
#22247=CARTESIAN_POINT ( 'NONE',  ( -330.4913330509368166, -103.0458197858324496, 55.34326076196052213 ) ) ;
#22253=DIRECTION ( 'NONE',  ( -0.000000000000000000, -0.4647231720437724478, -0.8854560256532078011 ) ) ;
#22259=ORIENTED_EDGE ( 'NONE', *, *, #50961, .F. ) ;
#22260=LINE ( 'NONE', #18340, #34858 ) ;
#22261=ORIENTED_EDGE ( 'NONE', *, *, #51905, .T. ) ;
#22268=VERTEX_POINT ( 'NONE', #25615 ) ;
#22270=EDGE_CURVE ( 'NONE', #20473, #40560, #32975, .T. ) ;
#22271=CARTESIAN_POINT ( 'NONE',  ( -305.0000000000000568, -103.7577981350106313, -56.65902810251876787 ) ) ;
#22275=VERTEX_POINT ( 'NONE', #12739 ) ;
#22279=EDGE_CURVE ( 'NONE', #20473, #31066, #45862, .T. ) ;
#22280=CARTESIAN_POINT ( 'NONE',  ( -336.3521761649654422, -121.8677111499054320, 59.00000000000001421 ) ) ;
#22282=EDGE_LOOP ( 'NONE', ( #46380, #42127, #26816, #10375 ) ) ;
#22283=CARTESIAN_POINT ( 'NONE',  ( -330.4913330509368166, -64.50000000000000000, -0.4999999999999549249 ) ) ;
#22291=ORIENTED_EDGE ( 'NONE', *, *, #23285, .T. ) ;
#22296=VECTOR ( 'NONE', #12646, 999.9999999999998863 ) ;
#22302=CARTESIAN_POINT ( 'NONE',  ( -336.3521761649654422, -127.9985676343858501, 58.88711093124869222 ) ) ;
#22304=CARTESIAN_POINT ( 'NONE',  ( -336.3521761649654422, -169.4076645216271402, -37.15394033962039089 ) ) ;
#22305=AXIS2_PLACEMENT_3D ( 'NONE', #17259, #44847, #49837 ) ;
#22306=LINE ( 'NONE', #30443, #4828 ) ;
#22307=AXIS2_PLACEMENT_3D ( 'NONE', #34034, #2746, #18782 ) ;
#22311=ORIENTED_EDGE ( 'NONE', *, *, #44941, .F. ) ;
#22318=DIRECTION ( 'NONE',  ( 0.000000000000000000, -0.1205366802553095168, 0.9927088740980556381 ) ) ;
#22323=VECTOR ( 'NONE', #34385, 1000.000000000000000 ) ;
#22325=DIRECTION ( 'NONE',  ( -1.000000000000000000, 0.000000000000000000, 0.000000000000000000 ) ) ;
#22328=CARTESIAN_POINT ( 'NONE',  ( -339.1964088526558498, -84.00150778970699150, 43.83057281297409702 ) ) ;
#22329=ORIENTED_EDGE ( 'NONE', *, *, #45830, .F. ) ;
#22332=DIRECTION ( 'NONE',  ( -0.000000000000000000, 0.3546048870425235200, -0.9350162426854194964 ) ) ;
#22333=CARTESIAN_POINT ( 'NONE',  ( -305.0000000000000568, -122.9999999999997158, 59.99791663049642665 ) ) ;
#22334=CARTESIAN_POINT ( 'NONE',  ( -339.1964088526558498, -143.9541802141672235, -55.34326076196065003 ) ) ;
#22337=EDGE_CURVE ( 'NONE', #4879, #51539, #22378, .T. ) ;
#22339=CARTESIAN_POINT ( 'NONE',  ( -336.3521761649654422, -83.15397741537739762, 43.07972642080338233 ) ) ;
#22352=AXIS2_PLACEMENT_3D ( 'NONE', #38886, #7099, #23389 ) ;
#22354=EDGE_LOOP ( 'NONE', ( #20371, #22962, #24973, #4024 ) ) ;
#22358=PLANE ( 'NONE',  #40770 ) ;
#22363=CARTESIAN_POINT ( 'NONE',  ( -330.4913330509368166, -89.57268800991444380, 48.27201571435978877 ) ) ;
#22364=CARTESIAN_POINT ( 'NONE',  ( -332.3517673607765914, -143.2422018649890276, 56.65902810251888155 ) ) ;
#22368=VECTOR ( 'NONE', #10660, 1000.000000000000227 ) ;
#22369=CIRCLE ( 'NONE', #50108, 60.00000000000000000 ) ;
#22370=CARTESIAN_POINT ( 'NONE',  ( -336.3521761649654422, -126.1322888500942270, -59.94223098458773080 ) ) ;
#22373=ORIENTED_EDGE ( 'NONE', *, *, #8283, .F. ) ;
#22374=DIRECTION ( 'NONE',  ( 0.000000000000000000, 0.9709418174260553425, 0.2393156642875448881 ) ) ;
#22376=DIRECTION ( 'NONE',  ( 0.000000000000000000, 0.000000000000000000, -1.000000000000000000 ) ) ;
#22378=CIRCLE ( 'NONE', #11494, 60.00000000000000000 ) ;
#22380=AXIS2_PLACEMENT_3D ( 'NONE', #32030, #24171, #4194 ) ;
#22383=AXIS2_PLACEMENT_3D ( 'NONE', #39350, #10458, #47510 ) ;
#22385=ADVANCED_FACE ( 'NONE', ( #29303 ), #29555, .F. ) ;
#22386=ADVANCED_FACE ( 'NONE', ( #5147 ), #5404, .F. ) ;
#22387=EDGE_CURVE ( 'NONE', #20132, #16530, #25366, .T. ) ;
#22390=DIRECTION ( 'NONE',  ( -1.000000000000000000, -0.000000000000000000, 0.000000000000000000 ) ) ;
#22395=LINE ( 'NONE', #22136, #21033 ) ;
#22399=EDGE_CURVE ( 'NONE', #19699, #17256, #5669, .T. ) ;
#22400=CARTESIAN_POINT ( 'NONE',  ( -336.3521761649654422, -180.4803820837415458, -18.79457521708939183 ) ) ;
#22401=ORIENTED_EDGE ( 'NONE', *, *, #4499, .T. ) ;
#22405=EDGE_CURVE ( 'NONE', #6473, #26602, #1707, .T. ) ;
#22406=CARTESIAN_POINT ( 'NONE',  ( -365.0000000000001137, -168.5000000000000284, 0.000000000000000000 ) ) ;
#22411=ORIENTED_EDGE ( 'NONE', *, *, #26895, .F. ) ;
#22413=VECTOR ( 'NONE', #26815, 1000.000000000000000 ) ;
#22419=CARTESIAN_POINT ( 'NONE',  ( -332.3517673607765914, -126.1322888500942270, -59.00000000000001421 ) ) ;
#22422=FACE_BOUND ( 'NONE', #40445, .T. ) ;
#22424=EDGE_LOOP ( 'NONE', ( #24996, #22173, #16709, #33306 ) ) ;
#22425=CARTESIAN_POINT ( 'NONE',  ( -332.3517673607765914, -174.5186198893880771, 29.74944317415823392 ) ) ;
#22426=ORIENTED_EDGE ( 'NONE', *, *, #21388, .F. ) ;
#22430=CARTESIAN_POINT ( 'NONE',  ( -330.4913330509368166, -157.1712093821527390, 49.66134974749710551 ) ) ;
#22432=AXIS2_PLACEMENT_3D ( 'NONE', #38675, #18718, #25442 ) ;
#22433=VECTOR ( 'NONE', #26355, 1000.000000000000000 ) ;
#22435=LINE ( 'NONE', #34254, #4560 ) ;
#22440=LINE ( 'NONE', #46108, #6946 ) ;
#22442=ORIENTED_EDGE ( 'NONE', *, *, #2922, .T. ) ;
#22443=FACE_OUTER_BOUND ( 'NONE', #6305, .T. ) ;
#22446=ORIENTED_EDGE ( 'NONE', *, *, #15402, .T. ) ;
#22452=AXIS2_PLACEMENT_3D ( 'NONE', #18660, #30727, #3393 ) ;
#22455=EDGE_LOOP ( 'NONE', ( #3925, #24707, #21539, #26779 ) ) ;
#22457=DIRECTION ( 'NONE',  ( -1.000000000000000000, -0.000000000000000000, 0.000000000000000000 ) ) ;
#22461=EDGE_CURVE ( 'NONE', #49313, #7901, #6181, .T. ) ;
#22462=EDGE_CURVE ( 'NONE', #45033, #2959, #2226, .T. ) ;
#22467=EDGE_CURVE ( 'NONE', #4655, #21321, #22715, .T. ) ;
#22471=CIRCLE ( 'NONE', #14104, 60.00000000000000000 ) ;
#22477=DIRECTION ( 'NONE',  ( 1.000000000000000000, -0.000000000000000000, -0.000000000000000000 ) ) ;
#22482=EDGE_CURVE ( 'NONE', #18723, #5376, #28299, .T. ) ;
#22485=ORIENTED_EDGE ( 'NONE', *, *, #1061, .F. ) ;
#22486=EDGE_CURVE ( 'NONE', #37313, #23381, #14579, .T. ) ;
#22489=EDGE_CURVE ( 'NONE', #48882, #30266, #46905, .T. ) ;
#22496=DIRECTION ( 'NONE',  ( 0.000000000000000000, -7.100801428331730794E-14, 1.000000000000000000 ) ) ;
#22497=VECTOR ( 'NONE', #18282, 1000.000000000000000 ) ;
#22505=DIRECTION ( 'NONE',  ( -1.000000000000000000, 0.000000000000000000, 8.718379230999707126E-17 ) ) ;
#22506=EDGE_CURVE ( 'NONE', #15659, #6808, #51119, .T. ) ;
#22510=DIRECTION ( 'NONE',  ( 0.000000000000000000, -0.7485107481710954191, 0.6631226582408017434 ) ) ;
#22513=DIRECTION ( 'NONE',  ( 1.000000000000000000, 2.086444717177488260E-17, -8.465038975556413550E-17 ) ) ;
#22514=ORIENTED_EDGE ( 'NONE', *, *, #24571, .F. ) ;
#22520=EDGE_LOOP ( 'NONE', ( #10430, #12701, #4999, #24317 ) ) ;
#22524=DIRECTION ( 'NONE',  ( -1.000000000000000000, 0.000000000000000000, 0.000000000000000000 ) ) ;
#22532=CIRCLE ( 'NONE', #51910, 60.00000000000000000 ) ;
#22535=CARTESIAN_POINT ( 'NONE',  ( -336.3521761649654422, -176.5004679656469477, -25.97334715265976612 ) ) ;
#22537=EDGE_LOOP ( 'NONE', ( #38212, #37916, #51430, #22591 ) ) ;
#22544=ORIENTED_EDGE ( 'NONE', *, *, #7912, .T. ) ;
#22550=CARTESIAN_POINT ( 'NONE',  ( -305.0000000000000568, -157.1712093821529947, 49.66134974749694209 ) ) ;
#22551=ORIENTED_EDGE ( 'NONE', *, *, #42988, .T. ) ;
#22557=DIRECTION ( 'NONE',  ( 0.000000000000000000, 0.000000000000000000, -1.000000000000000000 ) ) ;
#22562=CARTESIAN_POINT ( 'NONE',  ( -305.0000000000000568, -89.00580675195290326, 49.09328500076543378 ) ) ;
#22564=CARTESIAN_POINT ( 'NONE',  ( 0.000000000000000000, -89.98417994286123189, 48.55604808772534398 ) ) ;
#22568=FACE_OUTER_BOUND ( 'NONE', #129, .T. ) ;
#22572=AXIS2_PLACEMENT_3D ( 'NONE', #16786, #28580, #29103 ) ;
#22577=CARTESIAN_POINT ( 'NONE',  ( -332.3517673607765914, -123.5000000000000284, 0.000000000000000000 ) ) ;
#22580=DIRECTION ( 'NONE',  ( 1.000000000000000000, 3.091579882402645797E-17, 8.151826190875899055E-17 ) ) ;
#22581=DIRECTION ( 'NONE',  ( 0.000000000000000000, 0.8229838658936556861, -0.5680647467311569221 ) ) ;
#22591=ORIENTED_EDGE ( 'NONE', *, *, #50643, .T. ) ;
#22594=CARTESIAN_POINT ( 'NONE',  ( -336.3521761649654422, -178.0871407151310279, 22.44790492310219676 ) ) ;
#22597=LINE ( 'NONE', #18648, #39019 ) ;
#22601=FACE_OUTER_BOUND ( 'NONE', #39089, .T. ) ;
#22604=VECTOR ( 'NONE', #10167, 1000.000000000000000 ) ;
#22610=ORIENTED_EDGE ( 'NONE', *, *, #5735, .F. ) ;
#22616=CARTESIAN_POINT ( 'NONE',  ( -339.1964088526558498, -116.8846903019852164, -58.63009191191289915 ) ) ;
#22618=FACE_OUTER_BOUND ( 'NONE', #42771, .T. ) ;
#22625=AXIS2_PLACEMENT_3D ( 'NONE', #42172, #6195, #17244 ) ;
#22626=DIRECTION ( 'NONE',  ( -0.000000000000000000, -0.3546048870425267951, 0.9350162426854181641 ) ) ;
#22629=CARTESIAN_POINT ( 'NONE',  ( -336.3521761649654422, -182.5000000000000568, 2.632288850093980503 ) ) ;
#22636=DIRECTION ( 'NONE',  ( 1.000000000000000000, 0.000000000000000000, -0.000000000000000000 ) ) ;
#22638=AXIS2_PLACEMENT_3D ( 'NONE', #25755, #33635, #4747 ) ;
#22651=VERTEX_POINT ( 'NONE', #15609 ) ;
#22653=AXIS2_PLACEMENT_3D ( 'NONE', #50310, #18750, #22176 ) ;
#22655=DIRECTION ( 'NONE',  ( 0.000000000000000000, 0.2393156642875615969, 0.9709418174260511236 ) ) ;
#22658=ORIENTED_EDGE ( 'NONE', *, *, #4429, .F. ) ;
#22659=EDGE_CURVE ( 'NONE', #32832, #13489, #30822, .T. ) ;
#22660=DIRECTION ( 'NONE',  ( 1.000000000000000000, -0.000000000000000000, -0.000000000000000000 ) ) ;
#22662=DIRECTION ( 'NONE',  ( 0.000000000000000000, 0.000000000000000000, -1.000000000000000000 ) ) ;
#22667=ORIENTED_EDGE ( 'NONE', *, *, #7472, .F. ) ;
#22676=FACE_BOUND ( 'NONE', #31931, .T. ) ;
#22679=VERTEX_POINT ( 'NONE', #8477 ) ;
#22688=DIRECTION ( 'NONE',  ( 1.000000000000000000, 0.000000000000000000, 0.000000000000000000 ) ) ;
#22689=EDGE_CURVE ( 'NONE', #38924, #13962, #27935, .T. ) ;
#22691=CIRCLE ( 'NONE', #16845, 60.00000000000000000 ) ;
#22694=DIRECTION ( 'NONE',  ( -1.000000000000000000, -0.000000000000000000, -0.000000000000000000 ) ) ;
#22695=FACE_OUTER_BOUND ( 'NONE', #25747, .T. ) ;
#22698=LINE ( 'NONE', #2717, #2273 ) ;
#22699=ADVANCED_FACE ( 'NONE', ( #3763 ), #11658, .T. ) ;
#22700=EDGE_CURVE ( 'NONE', #17498, #12667, #40012, .T. ) ;
#22705=DIRECTION ( 'NONE',  ( 0.000000000000000000, -0.4647231720437755564, -0.8854560256532062468 ) ) ;
#22707=DIRECTION ( 'NONE',  ( -0.000000000000000000, 0.2393156642875685636, 0.9709418174260492362 ) ) ;
#22715=LINE ( 'NONE', #7202, #23289 ) ;
#22728=FACE_OUTER_BOUND ( 'NONE', #48908, .T. ) ;
#22736=ADVANCED_FACE ( 'NONE', ( #28698 ), #20570, .F. ) ;
#22737=VERTEX_POINT ( 'NONE', #2283 ) ;
#22740=CARTESIAN_POINT ( 'NONE',  ( -332.3517673607765914, -114.7679482383557144, 58.37307289257701370 ) ) ;
#22742=EDGE_CURVE ( 'NONE', #25920, #33208, #18814, .T. ) ;
#22747=EDGE_CURVE ( 'NONE', #5970, #19616, #31160, .T. ) ;
#22748=LINE ( 'NONE', #6210, #16487 ) ;
#22749=EDGE_CURVE ( 'NONE', #4422, #16821, #42206, .T. ) ;
#22755=ORIENTED_EDGE ( 'NONE', *, *, #15359, .F. ) ;
#22756=AXIS2_PLACEMENT_3D ( 'NONE', #41034, #40503, #48677 ) ;
#22768=ORIENTED_EDGE ( 'NONE', *, *, #41552, .T. ) ;
#22773=VERTEX_POINT ( 'NONE', #3045 ) ;
#22774=ORIENTED_EDGE ( 'NONE', *, *, #48828, .F. ) ;
#22778=LINE ( 'NONE', #2793, #14254 ) ;
#22780=DIRECTION ( 'NONE',  ( -0.000000000000000000, 0.9350162426854107256, -0.3546048870425463906 ) ) ;
#22782=PLANE ( 'NONE',  #43166 ) ;
#22796=CARTESIAN_POINT ( 'NONE',  ( 0.000000000000000000, -102.5783116644905562, -55.16595831843955722 ) ) ;
#22797=VECTOR ( 'NONE', #21448, 1000.000000000000000 ) ;
#22798=ORIENTED_EDGE ( 'NONE', *, *, #37705, .F. ) ;
#22802=CARTESIAN_POINT ( 'NONE',  ( -339.1964088526558498, -150.4759391377552618, 52.47426709956155122 ) ) ;
#22803=CARTESIAN_POINT ( 'NONE',  ( 0.000000000000000000, -64.50000000000000000, 0.000000000000000000 ) ) ;
#22804=VERTEX_POINT ( 'NONE', #39034 ) ;
#22807=EDGE_CURVE ( 'NONE', #27872, #48164, #619, .T. ) ;
#22809=CARTESIAN_POINT ( 'NONE',  ( -339.1964088526558498, -84.75001853787875916, -44.49369547121548862 ) ) ;
#22811=ORIENTED_EDGE ( 'NONE', *, *, #14816, .T. ) ;
#22812=DIRECTION ( 'NONE',  ( -0.000000000000000000, 0.8229838658936494689, -0.5680647467311658039 ) ) ;
#22815=EDGE_CURVE ( 'NONE', #32799, #39057, #38779, .T. ) ;
#22819=AXIS2_PLACEMENT_3D ( 'NONE', #27350, #11060, #2423 ) ;
#22824=VERTEX_POINT ( 'NONE', #3562 ) ;
#22828=LINE ( 'NONE', #14433, #27931 ) ;
#22829=VECTOR ( 'NONE', #46025, 1000.000000000000000 ) ;
#22832=VERTEX_POINT ( 'NONE', #19853 ) ;
#22837=VERTEX_POINT ( 'NONE', #19592 ) ;
#22838=CARTESIAN_POINT ( 'NONE',  ( -332.3517673607765914, -123.5000000000000284, 0.000000000000000000 ) ) ;
#22839=VECTOR ( 'NONE', #12921, 1000.000000000000000 ) ;
#22842=ORIENTED_EDGE ( 'NONE', *, *, #49242, .T. ) ;
#22843=CARTESIAN_POINT ( 'NONE',  ( -332.3517673607765914, -152.3639871485048900, -51.48334306143194539 ) ) ;
#22844=LINE ( 'NONE', #35967, #12155 ) ;
#22845=ORIENTED_EDGE ( 'NONE', *, *, #8944, .T. ) ;
#22847=AXIS2_PLACEMENT_3D ( 'NONE', #8481, #40534, #24781 ) ;
#22851=ORIENTED_EDGE ( 'NONE', *, *, #49983, .T. ) ;
#22854=ORIENTED_EDGE ( 'NONE', *, *, #29793, .T. ) ;
#22857=EDGE_LOOP ( 'NONE', ( #5955, #39108, #6665, #36875 ) ) ;
#22861=CARTESIAN_POINT ( 'NONE',  ( 0.000000000000000000, -182.0698235717852924, -7.111664135063673342 ) ) ;
#22863=ORIENTED_EDGE ( 'NONE', *, *, #16291, .T. ) ;
#22865=PLANE ( 'NONE',  #22352 ) ;
#22866=DIRECTION ( 'NONE',  ( 0.000000000000000000, 0.000000000000000000, 1.000000000000000000 ) ) ;
#22871=FACE_OUTER_BOUND ( 'NONE', #15634, .T. ) ;
#22875=ORIENTED_EDGE ( 'NONE', *, *, #5580, .T. ) ;
#22877=CARTESIAN_POINT ( 'NONE',  ( -332.3517673607765914, -113.7752393642576720, 58.25253621232167944 ) ) ;
#22878=CARTESIAN_POINT ( 'NONE',  ( -339.1964088526558498, -180.6659093959934523, -14.60509510167853264 ) ) ;
#22887=PLANE ( 'NONE',  #11433 ) ;
#22893=VECTOR ( 'NONE', #12009, 1000.000000000000000 ) ;
#22894=LINE ( 'NONE', #47333, #41119 ) ;
#22895=EDGE_CURVE ( 'NONE', #34569, #49741, #36391, .T. ) ;
#22900=LINE ( 'NONE', #46828, #43495 ) ;
#22902=EDGE_CURVE ( 'NONE', #18461, #49438, #22471, .T. ) ;
#22913=EDGE_LOOP ( 'NONE', ( #16779, #7677, #7663, #19098 ) ) ;
#22914=DIRECTION ( 'NONE',  ( 0.000000000000000000, 0.000000000000000000, 1.000000000000000000 ) ) ;
#22915=EDGE_LOOP ( 'NONE', ( #5282, #29537, #49357, #11510 ) ) ;
#22920=VECTOR ( 'NONE', #2349, 1000.000000000000000 ) ;
#22921=VERTEX_POINT ( 'NONE', #36135 ) ;
#22927=ORIENTED_EDGE ( 'NONE', *, *, #6628, .F. ) ;
#22929=PLANE ( 'NONE',  #11403 ) ;
#22931=EDGE_CURVE ( 'NONE', #39919, #45092, #48510, .T. ) ;
#22952=EDGE_CURVE ( 'NONE', #3411, #32153, #37580, .T. ) ;
#22954=PLANE ( 'NONE',  #37923 ) ;
#22959=DIRECTION ( 'NONE',  ( 1.000000000000000000, -0.000000000000000000, -0.000000000000000000 ) ) ;
#22962=ORIENTED_EDGE ( 'NONE', *, *, #9365, .F. ) ;
#22970=ORIENTED_EDGE ( 'NONE', *, *, #29996, .F. ) ;
#22974=PLANE ( 'NONE',  #35800 ) ;
#22978=VERTEX_POINT ( 'NONE', #12218 ) ;
#22983=AXIS2_PLACEMENT_3D ( 'NONE', #33856, #41994, #5770 ) ;
#22988=DIRECTION ( 'NONE',  ( -1.000000000000000000, 8.589602288500872567E-15, 5.928974370888848022E-15 ) ) ;
#22989=LINE ( 'NONE', #10902, #3056 ) ;
#22990=FACE_OUTER_BOUND ( 'NONE', #35770, .T. ) ;
#22994=DIRECTION ( 'NONE',  ( 1.000000000000000000, -0.000000000000000000, -0.000000000000000000 ) ) ;
#22999=EDGE_CURVE ( 'NONE', #25253, #13145, #4602, .T. ) ;
#23000=CARTESIAN_POINT ( 'NONE',  ( -339.1964088526558498, -84.00150778970767362, -43.83057281297470098 ) ) ;
#23001=EDGE_LOOP ( 'NONE', ( #38692, #47232, #49020, #29470 ) ) ;
#23004=CARTESIAN_POINT ( 'NONE',  ( -339.1964088526558498, -124.0000000000002700, -59.00000000000002132 ) ) ;
#23009=CARTESIAN_POINT ( 'NONE',  ( -336.3521761649654422, -73.44864141332200802, 31.34948880313848107 ) ) ;
#23015=ORIENTED_EDGE ( 'NONE', *, *, #24239, .F. ) ;
#23022=CARTESIAN_POINT ( 'NONE',  ( -332.3517673607765914, -92.15051119686104641, -50.05135858667769355 ) ) ;
#23032=CARTESIAN_POINT ( 'NONE',  ( -339.1964088526558498, -115.7716958700746233, 59.50019592636127896 ) ) ;
#23035=ADVANCED_FACE ( 'NONE', ( #17740 ), #1701, .F. ) ;
#23037=ADVANCED_FACE ( 'NONE', ( #9333 ), #33754, .F. ) ;
#23038=CARTESIAN_POINT ( 'NONE',  ( -305.0000000000000568, -161.2787550547969033, 46.61293454085098631 ) ) ;
#23039=EDGE_LOOP ( 'NONE', ( #7359, #495, #12612, #45105 ) ) ;
#23047=VECTOR ( 'NONE', #50716, 1000.000000000000000 ) ;
#23054=EDGE_LOOP ( 'NONE', ( #40384, #1157, #30421, #17899 ) ) ;
#23055=CIRCLE ( 'NONE', #49885, 14.36509618646847386 ) ;
#23059=CARTESIAN_POINT ( 'NONE',  ( -330.4913330509368166, -179.7763290203209579, -20.80804632820165168 ) ) ;
#23061=ADVANCED_FACE ( 'NONE', ( #20629 ), #36664, .F. ) ;
#23073=FACE_OUTER_BOUND ( 'NONE', #4764, .T. ) ;
#23074=CARTESIAN_POINT ( 'NONE',  ( -330.4913330509368166, -71.49045607248250178, -27.86139516340898581 ) ) ;
#23077=LINE ( 'NONE', #47517, #5996 ) ;
#23080=VERTEX_POINT ( 'NONE', #12992 ) ;
#23081=EDGE_CURVE ( 'NONE', #47556, #32799, #44295, .T. ) ;
#23082=LINE ( 'NONE', #31215, #25119 ) ;
#23088=DIRECTION ( 'NONE',  ( 0.000000000000000000, 0.4647231720437631775, -0.8854560256532126861 ) ) ;
#23093=LINE ( 'NONE', #19401, #46042 ) ;
#23095=MECHANICAL_DESIGN_GEOMETRIC_PRESENTATION_REPRESENTATION('',(#2078),#28099);
#23097=AXIS2_PLACEMENT_3D ( 'NONE', #35882, #34829, #35103 ) ;
#23099=EDGE_CURVE ( 'NONE', #8637, #29121, #18762, .T. ) ;
#23102=EDGE_CURVE ( 'NONE', #32388, #39056, #30074, .T. ) ;
#23103=VECTOR ( 'NONE', #33048, 1000.000000000000000 ) ;
#23107=LINE ( 'NONE', #38351, #25030 ) ;
#23110=EDGE_CURVE ( 'NONE', #22832, #27333, #17994, .T. ) ;
#23112=ORIENTED_EDGE ( 'NONE', *, *, #24146, .F. ) ;
#23115=DIRECTION ( 'NONE',  ( -0.000000000000000000, -0.8854560256532062468, 0.4647231720437755564 ) ) ;
#23117=EDGE_CURVE ( 'NONE', #36354, #21929, #18257, .T. ) ;
#23118=PLANE ( 'NONE',  #49266 ) ;
#23119=LINE ( 'NONE', #11268, #5696 ) ;
#23122=ORIENTED_EDGE ( 'NONE', *, *, #48967, .T. ) ;
#23124=VECTOR ( 'NONE', #9044, 1000.000000000000000 ) ;
#23130=DIRECTION ( 'NONE',  ( 0.000000000000000000, 0.9350162426854146114, -0.3546048870425363986 ) ) ;
#23132=LINE ( 'NONE', #11278, #24887 ) ;
#23139=EDGE_CURVE ( 'NONE', #37538, #37621, #5916, .T. ) ;
#23141=ORIENTED_EDGE ( 'NONE', *, *, #8409, .T. ) ;
#23142=CARTESIAN_POINT ( 'NONE',  ( -330.4913330509368166, -178.4886558749180949, 21.38919645685269444 ) ) ;
#23157=DIRECTION ( 'NONE',  ( 1.043714542225393697E-14, -0.5680647467311569221, -0.8229838658936556861 ) ) ;
#23159=DIRECTION ( 'NONE',  ( 0.000000000000000000, 0.000000000000000000, 1.000000000000000000 ) ) ;
#23160=VERTEX_POINT ( 'NONE', #22187 ) ;
#23161=ORIENTED_EDGE ( 'NONE', *, *, #43583, .T. ) ;
#23162=VECTOR ( 'NONE', #9963, 1000.000000000000000 ) ;
#23168=EDGE_CURVE ( 'NONE', #6473, #39339, #34519, .T. ) ;
#23169=DIRECTION ( 'NONE',  ( 0.000000000000000000, 0.9709418174260511236, -0.2393156642875615969 ) ) ;
#23171=DIRECTION ( 'NONE',  ( 0.000000000000000000, -0.2393156642875685636, -0.9709418174260492362 ) ) ;
#23174=CARTESIAN_POINT ( 'NONE',  ( -332.3517673607765914, -182.5000000000000568, 2.632288850093980503 ) ) ;
#23175=ORIENTED_EDGE ( 'NONE', *, *, #6799, .F. ) ;
#23178=DIRECTION ( 'NONE',  ( 0.000000000000000000, -4.093947403305264743E-14, -1.000000000000000000 ) ) ;
#23184=DIRECTION ( 'NONE',  ( -0.000000000000000000, 0.3546048870425331789, -0.9350162426854158326 ) ) ;
#23193=ORIENTED_EDGE ( 'NONE', *, *, #30601, .T. ) ;
#23195=LINE ( 'NONE', #39212, #7307 ) ;
#23197=EDGE_LOOP ( 'NONE', ( #31818, #17707, #22329, #38300 ) ) ;
#23198=CYLINDRICAL_SURFACE ( 'NONE', #724, 60.00000000000000000 ) ;
#23199=FACE_OUTER_BOUND ( 'NONE', #32823, .T. ) ;
#23203=VERTEX_POINT ( 'NONE', #2983 ) ;
#23204=AXIS2_PLACEMENT_3D ( 'NONE', #41417, #5438, #21457 ) ;
#23205=VECTOR ( 'NONE', #4136, 1000.000000000000000 ) ;
#23210=DIRECTION ( 'NONE',  ( -0.000000000000000000, 0.4647231720437789981, 0.8854560256532044704 ) ) ;
#23214=AXIS2_PLACEMENT_3D ( 'NONE', #6139, #33971, #50021 ) ;
#23216=DIRECTION ( 'NONE',  ( 0.000000000000000000, -1.942890293094023946E-14, -1.000000000000000000 ) ) ;
#23220=VECTOR ( 'NONE', #10729, 1000.000000000000000 ) ;
#23222=ORIENTED_EDGE ( 'NONE', *, *, #50526, .T. ) ;
#23224=AXIS2_PLACEMENT_3D ( 'NONE', #44813, #5141, #37436 ) ;
#23228=ORIENTED_EDGE ( 'NONE', *, *, #36862, .F. ) ;
#23232=CARTESIAN_POINT ( 'NONE',  ( -339.1964088526558498, -171.7720157143604069, -33.92731199008472487 ) ) ;
#23236=VERTEX_POINT ( 'NONE', #50831 ) ;
#23239=CARTESIAN_POINT ( 'NONE',  ( -330.4913330509368166, -167.9936954712156023, -38.74998146212117689 ) ) ;
#23241=AXIS2_PLACEMENT_3D ( 'NONE', #41885, #26813, #21664 ) ;
#23245=DIRECTION ( 'NONE',  ( -1.000000000000000000, 0.000000000000000000, 0.000000000000000000 ) ) ;
#23251=ORIENTED_EDGE ( 'NONE', *, *, #15398, .F. ) ;
#23255=CARTESIAN_POINT ( 'NONE',  ( -305.0000000000000568, -65.36517161715264024, 14.84391218300897464 ) ) ;
#23258=ADVANCED_FACE ( 'NONE', ( #9848 ), #21930, .F. ) ;
#23259=DIRECTION ( 'NONE',  ( -0.000000000000000000, 0.6631226582407937498, -0.7485107481711024136 ) ) ;
#23260=VECTOR ( 'NONE', #6127, 1000.000000000000000 ) ;
#23262=CARTESIAN_POINT ( 'NONE',  ( -330.4913330509368166, -179.4217241332781612, 21.74306257088775141 ) ) ;
#23267=AXIS2_PLACEMENT_3D ( 'NONE', #5821, #33646, #9739 ) ;
#23268=VERTEX_POINT ( 'NONE', #32129 ) ;
#23276=LINE ( 'NONE', #27715, #29491 ) ;
#23277=ORIENTED_EDGE ( 'NONE', *, *, #1105, .T. ) ;
#23278=ORIENTED_EDGE ( 'NONE', *, *, #35411, .T. ) ;
#23279=AXIS2_PLACEMENT_3D ( 'NONE', #32857, #2029, #4759 ) ;
#23282=CARTESIAN_POINT ( 'NONE',  ( -336.3521761649653854, -71.15086438280971493, -29.31839013542551342 ) ) ;
#23284=CIRCLE ( 'NONE', #25792, 60.00000000000000000 ) ;
#23285=EDGE_CURVE ( 'NONE', #47681, #50353, #35817, .T. ) ;
#23286=ORIENTED_EDGE ( 'NONE', *, *, #16996, .F. ) ;
#23289=VECTOR ( 'NONE', #31107, 1000.000000000000000 ) ;
#23293=CARTESIAN_POINT ( 'NONE',  ( -339.1964088526558498, -102.1108035431470427, 54.98865587491797413 ) ) ;
#23299=DIRECTION ( 'NONE',  ( 0.000000000000000000, 0.000000000000000000, 1.000000000000000000 ) ) ;
#23301=ORIENTED_EDGE ( 'NONE', *, *, #38525, .T. ) ;
#23304=VERTEX_POINT ( 'NONE', #27149 ) ;
#23314=ORIENTED_EDGE ( 'NONE', *, *, #3190, .T. ) ;
#23317=ORIENTED_EDGE ( 'NONE', *, *, #25665, .F. ) ;
#23320=VECTOR ( 'NONE', #18080, 1000.000000000000000 ) ;
#23324=VECTOR ( 'NONE', #22457, 1000.000000000000000 ) ;
#23325=LINE ( 'NONE', #44051, #48131 ) ;
#23331=CARTESIAN_POINT ( 'NONE',  ( -330.4913330509368166, -182.0095552316575152, 7.608018572113473432 ) ) ;
#23334=CARTESIAN_POINT ( 'NONE',  ( -330.4913330509368166, -71.02573290043878274, -26.97593913775585150 ) ) ;
#23338=VERTEX_POINT ( 'NONE', #47395 ) ;
#23347=ADVANCED_FACE ( 'NONE', ( #3750 ), #28895, .F. ) ;
#23349=EDGE_LOOP ( 'NONE', ( #32644, #16406, #6469, #8779 ) ) ;
#23356=EDGE_CURVE ( 'NONE', #20241, #4422, #19781, .T. ) ;
#23365=FACE_OUTER_BOUND ( 'NONE', #33760, .T. ) ;
#23369=ORIENTED_EDGE ( 'NONE', *, *, #38870, .F. ) ;
#23370=CARTESIAN_POINT ( 'NONE',  ( -336.3521761649654422, -128.9912765084839066, 58.76657425099337928 ) ) ;
#23373=CARTESIAN_POINT ( 'NONE',  ( -330.4913330509368166, -151.3613951634091848, -52.00954392751743427 ) ) ;
#23377=DIRECTION ( 'NONE',  ( -1.000000000000000000, -0.000000000000000000, 0.000000000000000000 ) ) ;
#23379=CARTESIAN_POINT ( 'NONE',  ( -332.3517673607765914, -123.5000000000000284, 0.000000000000000000 ) ) ;
#23381=VERTEX_POINT ( 'NONE', #3494 ) ;
#23386=AXIS2_PLACEMENT_3D ( 'NONE', #30294, #50539, #14539 ) ;
#23387=LINE ( 'NONE', #28077, #20641 ) ;
#23388=LINE ( 'NONE', #20211, #34743 ) ;
#23389=DIRECTION ( 'NONE',  ( 0.000000000000000000, 0.4647231720437631775, -0.8854560256532126861 ) ) ;
#23395=CARTESIAN_POINT ( 'NONE',  ( -339.1964088526558498, -123.5000000000000142, 60.00000000000000000 ) ) ;
#23405=EDGE_LOOP ( 'NONE', ( #7289, #6122, #51080, #24498 ) ) ;
#23411=LINE ( 'NONE', #19451, #21202 ) ;
#23414=CARTESIAN_POINT ( 'NONE',  ( -336.3521761649654422, -66.84438072661991725, -16.67542351306652648 ) ) ;
#23416=VERTEX_POINT ( 'NONE', #38341 ) ;
#23422=ADVANCED_FACE ( 'NONE', ( #49668 ), #13923, .F. ) ;
#23428=DIRECTION ( 'NONE',  ( 1.000000000000000000, 0.000000000000000000, 0.000000000000000000 ) ) ;
#23429=EDGE_LOOP ( 'NONE', ( #16782, #21955, #19449, #24516 ) ) ;
#23432=FACE_OUTER_BOUND ( 'NONE', #39578, .T. ) ;
#23433=VECTOR ( 'NONE', #50120, 1000.000000000000000 ) ;
#23434=CARTESIAN_POINT ( 'NONE',  ( -339.1964088526558498, -109.8658467157473666, -57.40522506028092664 ) ) ;
#23437=CARTESIAN_POINT ( 'NONE',  ( -330.4913330509368166, -123.5000000000000284, 0.000000000000000000 ) ) ;
#23439=PLANE ( 'NONE',  #13826 ) ;
#23440=ORIENTED_EDGE ( 'NONE', *, *, #7048, .T. ) ;
#23443=CARTESIAN_POINT ( 'NONE',  ( -336.3521761649654422, -133.2247606357419443, -58.25253621232173629 ) ) ;
#23447=AXIS2_PLACEMENT_3D ( 'NONE', #29199, #40035, #45501 ) ;
#23448=EDGE_CURVE ( 'NONE', #24719, #43748, #37579, .T. ) ;
#23449=FACE_OUTER_BOUND ( 'NONE', #33751, .T. ) ;
#23459=VERTEX_POINT ( 'NONE', #29678 ) ;
#23465=CARTESIAN_POINT ( 'NONE',  ( -332.3517673607765914, -94.63601285149479736, 51.48334306143172512 ) ) ;
#23469=EDGE_CURVE ( 'NONE', #20782, #15531, #14194, .T. ) ;
#23474=DIRECTION ( 'NONE',  ( 0.000000000000000000, -0.3546048870425463906, -0.9350162426854107256 ) ) ;
#23476=ORIENTED_EDGE ( 'NONE', *, *, #11280, .F. ) ;
#23481=ORIENTED_EDGE ( 'NONE', *, *, #50884, .T. ) ;
#23485=CARTESIAN_POINT ( 'NONE',  ( -339.1964088526558498, -182.1300919119129560, -6.615309698014600670 ) ) ;
#23487=LINE ( 'NONE', #7709, #16554 ) ;
#23495=AXIS2_PLACEMENT_3D ( 'NONE', #1574, #42273, #6289 ) ;
#23496=DIRECTION ( 'NONE',  ( -0.000000000000000000, -0.9709418174260502354, 0.2393156642875652051 ) ) ;
#23498=ORIENTED_EDGE ( 'NONE', *, *, #7275, .F. ) ;
#23503=VERTEX_POINT ( 'NONE', #10480 ) ;
#23504=CARTESIAN_POINT ( 'NONE',  ( -336.3521761649654422, -123.5000000000000284, 0.000000000000000000 ) ) ;
#23507=DIRECTION ( 'NONE',  ( 1.000000000000000000, -0.000000000000000000, -0.000000000000000000 ) ) ;
#23508=CARTESIAN_POINT ( 'NONE',  ( -336.3521761649654422, -87.81784868886214213, 47.06073758877343494 ) ) ;
#23513=VECTOR ( 'NONE', #16701, 1000.000000000000000 ) ;
#23523=DIRECTION ( 'NONE',  ( -8.718379230999704661E-17, -0.8229838658936613482, -0.5680647467311485954 ) ) ;
#23527=DIRECTION ( 'NONE',  ( 0.000000000000000000, 0.6631226582407964143, 0.7485107481710999711 ) ) ;
#23529=EDGE_LOOP ( 'NONE', ( #47535, #45619, #23112, #41440 ) ) ;
#23530=ORIENTED_EDGE ( 'NONE', *, *, #19255, .T. ) ;
#23536=EDGE_CURVE ( 'NONE', #34048, #19724, #31484, .T. ) ;
#23539=DIRECTION ( 'NONE',  ( 1.000000000000000000, 0.000000000000000000, -0.000000000000000000 ) ) ;
#23542=VERTEX_POINT ( 'NONE', #14443 ) ;
#23543=ORIENTED_EDGE ( 'NONE', *, *, #49768, .T. ) ;
#23544=AXIS2_PLACEMENT_3D ( 'NONE', #21036, #49433, #20249 ) ;
#23548=DIRECTION ( 'NONE',  ( -0.000000000000000000, 0.000000000000000000, 1.000000000000000000 ) ) ;
#23550=CARTESIAN_POINT ( 'NONE',  ( -330.4913330509368166, -68.15673923803930734, -20.45418021416698551 ) ) ;
#23555=EDGE_LOOP ( 'NONE', ( #18902, #27415, #20199, #51250 ) ) ;
#23559=VECTOR ( 'NONE', #28507, 1000.000000000000000 ) ;
#23562=DIRECTION ( 'NONE',  ( 1.043714542225393381E-14, -1.000000000000000000, 3.491481338843133355E-15 ) ) ;
#23564=LINE ( 'NONE', #27756, #3266 ) ;
#23565=VERTEX_POINT ( 'NONE', #43582 ) ;
#23569=ORIENTED_EDGE ( 'NONE', *, *, #6685, .T. ) ;
#23571=CARTESIAN_POINT ( 'NONE',  ( -332.3517673607765914, -123.5000000000000284, 0.000000000000000000 ) ) ;
#23572=DIRECTION ( 'NONE',  ( -0.000000000000000000, -0.6631226582407885317, 0.7485107481711069655 ) ) ;
#23573=CIRCLE ( 'NONE', #22756, 60.00000000000000000 ) ;
#23576=EDGE_CURVE ( 'NONE', #6394, #33644, #6565, .T. ) ;
#23578=CARTESIAN_POINT ( 'NONE',  ( -305.0000000000000568, -147.2170408776451609, -55.11353710303946940 ) ) ;
#23588=LINE ( 'NONE', #44861, #32969 ) ;
#23589=ORIENTED_EDGE ( 'NONE', *, *, #14695, .T. ) ;
#23591=VECTOR ( 'NONE', #1107, 1000.000000000000000 ) ;
#23593=DIRECTION ( 'NONE',  ( -1.000000000000000000, 0.000000000000000000, -0.000000000000000000 ) ) ;
#23598=ORIENTED_EDGE ( 'NONE', *, *, #5927, .T. ) ;
#23601=ORIENTED_EDGE ( 'NONE', *, *, #5033, .F. ) ;
#23606=ORIENTED_EDGE ( 'NONE', *, *, #2922, .F. ) ;
#23609=VERTEX_POINT ( 'NONE', #27021 ) ;
#23613=ORIENTED_EDGE ( 'NONE', *, *, #43974, .F. ) ;
#23615=EDGE_CURVE ( 'NONE', #21465, #31069, #23093, .T. ) ;
#23619=DIRECTION ( 'NONE',  ( -1.000000000000000000, 0.000000000000000000, 0.000000000000000000 ) ) ;
#23622=DIRECTION ( 'NONE',  ( 0.000000000000000000, 7.170190367370802131E-15, 1.000000000000000000 ) ) ;
#23625=DIRECTION ( 'NONE',  ( -0.000000000000000000, 1.000000000000000000, -1.047444401652940007E-14 ) ) ;
#23626=AXIS2_PLACEMENT_3D ( 'NONE', #15536, #12559, #36458 ) ;
#23630=DIRECTION ( 'NONE',  ( -0.000000000000000000, 0.5680647467311625842, 0.8229838658936516893 ) ) ;
#23633=ADVANCED_FACE ( 'NONE', ( #34905 ), #31226, .F. ) ;
#23640=DIRECTION ( 'NONE',  ( 0.000000000000000000, 0.9709418174260526779, 0.2393156642875547968 ) ) ;
#23653=DIRECTION ( 'NONE',  ( 1.000000000000000000, -0.000000000000000000, -0.000000000000000000 ) ) ;
#23655=FACE_OUTER_BOUND ( 'NONE', #4027, .T. ) ;
#23656=VECTOR ( 'NONE', #16885, 1000.000000000000000 ) ;
#23660=VECTOR ( 'NONE', #45613, 999.9999999999998863 ) ;
#23662=PLANE ( 'NONE',  #36783 ) ;
#23663=VERTEX_POINT ( 'NONE', #32255 ) ;
#23664=DIRECTION ( 'NONE',  ( 0.000000000000000000, 0.8854560256532110207, 0.4647231720437664526 ) ) ;
#23668=VERTEX_POINT ( 'NONE', #36453 ) ;
#23683=ADVANCED_FACE ( 'NONE', ( #44091 ), #51739, .F. ) ;
#23684=AXIS2_PLACEMENT_3D ( 'NONE', #33872, #30201, #30439 ) ;
#23685=DIRECTION ( 'NONE',  ( 0.000000000000000000, 0.000000000000000000, 1.000000000000000000 ) ) ;
#23687=CARTESIAN_POINT ( 'NONE',  ( -339.1964088526558498, -182.5000000000000568, -0.4999999999999543698 ) ) ;
#23690=CARTESIAN_POINT ( 'NONE',  ( -336.3521761649654422, -66.60506506233235768, -15.70448169564047092 ) ) ;
#23691=DIRECTION ( 'NONE',  ( 0.000000000000000000, -1.811051308919786607E-13, 1.000000000000000000 ) ) ;
#23701=ORIENTED_EDGE ( 'NONE', *, *, #12492, .F. ) ;
#23702=DIRECTION ( 'NONE',  ( 1.000000000000000000, 0.000000000000000000, 0.000000000000000000 ) ) ;
#23705=AXIS2_PLACEMENT_3D ( 'NONE', #17191, #45058, #21909 ) ;
#23707=LINE ( 'NONE', #27901, #34850 ) ;
#23709=EDGE_CURVE ( 'NONE', #4036, #13526, #3254, .T. ) ;
#23718=ORIENTED_EDGE ( 'NONE', *, *, #14346, .F. ) ;
#23719=CIRCLE ( 'NONE', #5287, 60.00000000000000000 ) ;
#23721=FACE_OUTER_BOUND ( 'NONE', #8627, .T. ) ;
#23727=PLANE ( 'NONE',  #8833 ) ;
#23730=FACE_OUTER_BOUND ( 'NONE', #21619, .T. ) ;
#23739=CARTESIAN_POINT ( 'NONE',  ( 0.000000000000000000, -137.6196241929653752, 57.28556722813723212 ) ) ;
#23740=CARTESIAN_POINT ( 'NONE',  ( -332.3517673607765914, -179.5993808087905279, -18.46045550523168899 ) ) ;
#23742=CARTESIAN_POINT ( 'NONE',  ( -336.3521761649654422, -85.59754891220836726, -45.24454186338619621 ) ) ;
#23749=EDGE_CURVE ( 'NONE', #7602, #11338, #12803, .T. ) ;
#23751=VECTOR ( 'NONE', #29147, 1000.000000000000000 ) ;
#23754=EDGE_CURVE ( 'NONE', #21574, #21379, #25424, .T. ) ;
#23755=ORIENTED_EDGE ( 'NONE', *, *, #5807, .T. ) ;
#23757=EDGE_LOOP ( 'NONE', ( #25516, #26616, #45976, #48564 ) ) ;
#23763=FACE_OUTER_BOUND ( 'NONE', #46784, .T. ) ;
#23764=FACE_OUTER_BOUND ( 'NONE', #8214, .T. ) ;
#23769=DIRECTION ( 'NONE',  ( -1.000000000000000000, 0.000000000000000000, 0.000000000000000000 ) ) ;
#23771=EDGE_CURVE ( 'NONE', #30123, #14634, #17556, .T. ) ;
#23779=CARTESIAN_POINT ( 'NONE',  ( -305.0000000000000568, -183.0001959263614424, -7.728304129924262078 ) ) ;
#23782=DIRECTION ( 'NONE',  ( 0.000000000000000000, -0.9350162426854107256, 0.3546048870425463906 ) ) ;
#23785=AXIS2_PLACEMENT_3D ( 'NONE', #35284, #47124, #51578 ) ;
#23789=LINE ( 'NONE', #39796, #14005 ) ;
#23790=AXIS2_PLACEMENT_3D ( 'NONE', #45913, #21978, #25659 ) ;
#23792=ORIENTED_EDGE ( 'NONE', *, *, #24215, .F. ) ;
#23810=VERTEX_POINT ( 'NONE', #33819 ) ;
#23820=DIRECTION ( 'NONE',  ( 1.000000000000000000, 1.043714542225393381E-14, 0.000000000000000000 ) ) ;
#23823=EDGE_LOOP ( 'NONE', ( #46511, #34342, #40843, #19291 ) ) ;
#23828=ADVANCED_FACE ( 'NONE', ( #21481, #33041, #49352 ), #41181, .T. ) ;
#23830=DIRECTION ( 'NONE',  ( 0.000000000000000000, 0.000000000000000000, 1.000000000000000000 ) ) ;
#23832=DIRECTION ( 'NONE',  ( -1.000000000000000000, -0.000000000000000000, -0.000000000000000000 ) ) ;
#23837=CARTESIAN_POINT ( 'NONE',  ( -336.3521761649654422, -168.7445418633863596, -37.90245108779149064 ) ) ;
#23840=EDGE_CURVE ( 'NONE', #1636, #33208, #8274, .T. ) ;
#23864=CARTESIAN_POINT ( 'NONE',  ( -336.3521761649654422, -181.4155151828941825, -11.56382487286496463 ) ) ;
#23867=CARTESIAN_POINT ( 'NONE',  ( -332.3517673607765914, -123.5000000000000284, 0.000000000000000000 ) ) ;
#23871=DIRECTION ( 'NONE',  ( -0.000000000000000000, 0.1205366802553199113, -0.9927088740980544168 ) ) ;
#23872=VERTEX_POINT ( 'NONE', #20969 ) ;
#23876=ORIENTED_EDGE ( 'NONE', *, *, #35175, .T. ) ;
#23877=DIRECTION ( 'NONE',  ( -8.718379230999705894E-17, -0.8854560256532044704, 0.4647231720437789981 ) ) ;
#23882=EDGE_LOOP ( 'NONE', ( #48686, #7055, #51724, #49667 ) ) ;
#23887=PLANE ( 'NONE',  #16586 ) ;
#23891=DIRECTION ( 'NONE',  ( -0.000000000000000000, 0.8854560256532110207, 0.4647231720437664526 ) ) ;
#23897=VECTOR ( 'NONE', #15547, 1000.000000000000000 ) ;
#23899=DIRECTION ( 'NONE',  ( -1.000000000000000000, -0.000000000000000000, -0.000000000000000000 ) ) ;
#23900=CARTESIAN_POINT ( 'NONE',  ( -336.3521761649654422, -65.82380048139334860, 12.53476669029061519 ) ) ;
#23902=ORIENTED_EDGE ( 'NONE', *, *, #47853, .T. ) ;
#23903=ORIENTED_EDGE ( 'NONE', *, *, #50961, .T. ) ;
#23905=CARTESIAN_POINT ( 'NONE',  ( -332.3517673607765914, -181.4155151828941825, -11.56382487286496463 ) ) ;
#23911=VERTEX_POINT ( 'NONE', #38015 ) ;
#23915=EDGE_CURVE ( 'NONE', #42173, #18306, #34083, .T. ) ;
#23920=FACE_OUTER_BOUND ( 'NONE', #39689, .T. ) ;
#23928=DIRECTION ( 'NONE',  ( -0.000000000000000000, 0.000000000000000000, 1.000000000000000000 ) ) ;
#23930=ADVANCED_FACE ( 'NONE', ( #26964 ), #35113, .T. ) ;
#23940=DIRECTION ( 'NONE',  ( 0.000000000000000000, -0.4647231720437724478, -0.8854560256532078011 ) ) ;
#23941=DIRECTION ( 'NONE',  ( 1.000000000000000000, 0.000000000000000000, -0.000000000000000000 ) ) ;
#23944=VERTEX_POINT ( 'NONE', #50386 ) ;
#23946=PLANE ( 'NONE',  #28692 ) ;
#23947=SHAPE_REPRESENTATION_RELATIONSHIP ( 'NONE' , 'NONE' ,  #33116, #7414 ) ;
#23951=VECTOR ( 'NONE', #13562, 1000.000000000000114 ) ;
#23955=AXIS2_PLACEMENT_3D ( 'NONE', #37322, #49165, #8688 ) ;
#23956=CARTESIAN_POINT ( 'NONE',  ( -336.3521761649654422, -82.40546666720629787, 42.41660376256258047 ) ) ;
#23960=ORIENTED_EDGE ( 'NONE', *, *, #20183, .T. ) ;
#23965=LINE ( 'NONE', #40766, #2270 ) ;
#23967=AXIS2_PLACEMENT_3D ( 'NONE', #51009, #15005, #39152 ) ;
#23970=FACE_OUTER_BOUND ( 'NONE', #2920, .T. ) ;
#23974=EDGE_CURVE ( 'NONE', #36669, #9672, #26714, .T. ) ;
#23976=EDGE_CURVE ( 'NONE', #21496, #28486, #10792, .T. ) ;
#23980=ORIENTED_EDGE ( 'NONE', *, *, #30472, .F. ) ;
#23983=EDGE_LOOP ( 'NONE', ( #34476, #25931, #47724, #42773 ) ) ;
#23990=CIRCLE ( 'NONE', #1344, 60.00000000000000000 ) ;
#23991=DIRECTION ( 'NONE',  ( -0.000000000000000000, -0.4647231720437724478, -0.8854560256532078011 ) ) ;
#23995=EDGE_LOOP ( 'NONE', ( #10005, #30559, #14042, #7627 ) ) ;
#23997=DIRECTION ( 'NONE',  ( 0.000000000000000000, -0.9709418174260544543, -0.2393156642875482465 ) ) ;
#24000=EDGE_CURVE ( 'NONE', #3155, #50821, #39330, .T. ) ;
#24001=DIRECTION ( 'NONE',  ( 0.000000000000000000, 0.6631226582407911962, -0.7485107481711046340 ) ) ;
#24002=CARTESIAN_POINT ( 'NONE',  ( -339.1964088526558498, -115.8919814278862503, 58.50955523165745831 ) ) ;
#24004=CARTESIAN_POINT ( 'NONE',  ( -332.3517673607765914, -140.1754235130667610, -56.65561927338005432 ) ) ;
#24010=ORIENTED_EDGE ( 'NONE', *, *, #788, .T. ) ;
#24011=AXIS2_PLACEMENT_3D ( 'NONE', #7808, #16222, #15454 ) ;
#24015=DIRECTION ( 'NONE',  ( 0.000000000000000000, -0.1205366802553199113, 0.9927088740980544168 ) ) ;
#24018=CIRCLE ( 'NONE', #12229, 60.00000000000000000 ) ;
#24021=DIRECTION ( 'NONE',  ( 1.000000000000000000, -0.000000000000000000, -0.000000000000000000 ) ) ;
#24023=CARTESIAN_POINT ( 'NONE',  ( -336.3521761649654422, -65.24746378767824240, -9.724760635741734660 ) ) ;
#24026=FACE_OUTER_BOUND ( 'NONE', #17357, .T. ) ;
#24027=VERTEX_POINT ( 'NONE', #22247 ) ;
#24039=DIRECTION ( 'NONE',  ( 1.000000000000000000, -0.000000000000000000, -0.000000000000000000 ) ) ;
#24040=ORIENTED_EDGE ( 'NONE', *, *, #1576, .T. ) ;
#24041=PLANE ( 'NONE',  #37038 ) ;
#24044=EDGE_CURVE ( 'NONE', #13064, #2622, #26443, .T. ) ;
#24046=LINE ( 'NONE', #19838, #42793 ) ;
#24052=ADVANCED_FACE ( 'NONE', ( #3320 ), #19354, .T. ) ;
#24055=EDGE_CURVE ( 'NONE', #49368, #19699, #640, .T. ) ;
#24056=CARTESIAN_POINT ( 'NONE',  ( -336.3521761649654422, -159.1821513111375452, -47.06073758877369073 ) ) ;
#24061=EDGE_CURVE ( 'NONE', #28636, #48811, #40299, .T. ) ;
#24065=DIRECTION ( 'NONE',  ( 1.000000000000000000, -0.000000000000000000, -0.000000000000000000 ) ) ;
#24068=DIRECTION ( 'NONE',  ( 0.000000000000000000, 1.850371707708594366E-15, 1.000000000000000000 ) ) ;
#24072=EDGE_CURVE ( 'NONE', #29379, #26067, #33032, .T. ) ;
#24073=VERTEX_POINT ( 'NONE', #32248 ) ;
#24076=VECTOR ( 'NONE', #31576, 1000.000000000000000 ) ;
#24077=EDGE_CURVE ( 'NONE', #42568, #49872, #41889, .T. ) ;
#24082=FACE_BOUND ( 'NONE', #32179, .T. ) ;
#24083=AXIS2_PLACEMENT_3D ( 'NONE', #42384, #22162, #45820 ) ;
#24088=EDGE_CURVE ( 'NONE', #22824, #16966, #24133, .T. ) ;
#24095=PLANE ( 'NONE',  #3118 ) ;
#24096=FACE_OUTER_BOUND ( 'NONE', #15103, .T. ) ;
#24097=CARTESIAN_POINT ( 'NONE',  ( -305.0000000000000568, -123.5000000000000284, 20.00000000000001066 ) ) ;
#24099=ORIENTED_EDGE ( 'NONE', *, *, #1027, .T. ) ;
#24100=DIRECTION ( 'NONE',  ( 1.000000000000000000, 0.000000000000000000, 0.000000000000000000 ) ) ;
#24102=EDGE_CURVE ( 'NONE', #19363, #48057, #16734, .T. ) ;
#24114=ORIENTED_EDGE ( 'NONE', *, *, #32332, .F. ) ;
#24115=DIRECTION ( 'NONE',  ( 1.000000000000000000, 0.000000000000000000, 0.000000000000000000 ) ) ;
#24128=VECTOR ( 'NONE', #7955, 1000.000000000000000 ) ;
#24129=VERTEX_POINT ( 'NONE', #37239 ) ;
#24131=ADVANCED_FACE ( 'NONE', ( #36979 ), #29346, .F. ) ;
#24133=LINE ( 'NONE', #41174, #4990 ) ;
#24134=DIRECTION ( 'NONE',  ( -0.000000000000000000, -0.6631226582407989678, -0.7485107481710977506 ) ) ;
#24135=CARTESIAN_POINT ( 'NONE',  ( -305.0000000000000568, -64.15626348514393840, -8.849911663702499709 ) ) ;
#24141=ORIENTED_EDGE ( 'NONE', *, *, #22747, .T. ) ;
#24142=EDGE_CURVE ( 'NONE', #29051, #38775, #10822, .T. ) ;
#24143=DIRECTION ( 'NONE',  ( -1.000000000000000000, 0.000000000000000000, 0.000000000000000000 ) ) ;
#24145=AXIS2_PLACEMENT_3D ( 'NONE', #49661, #12868, #32839 ) ;
#24146=EDGE_CURVE ( 'NONE', #35564, #21924, #28817, .T. ) ;
#24150=FACE_OUTER_BOUND ( 'NONE', #27125, .T. ) ;
#24154=VECTOR ( 'NONE', #1834, 1000.000000000000000 ) ;
#24157=ORIENTED_EDGE ( 'NONE', *, *, #11333, .T. ) ;
#24159=ORIENTED_EDGE ( 'NONE', *, *, #20947, .F. ) ;
#24162=CARTESIAN_POINT ( 'NONE',  ( -339.1964088526558498, -96.52406086224361559, 52.47426709956096147 ) ) ;
#24165=VECTOR ( 'NONE', #51233, 1000.000000000000000 ) ;
#24169=LINE ( 'NONE', #40178, #12074 ) ;
#24171=DIRECTION ( 'NONE',  ( -0.000000000000000000, 0.9709418174260527890, 0.2393156642875547968 ) ) ;
#24174=PLANE ( 'NONE',  #25488 ) ;
#24177=ORIENTED_EDGE ( 'NONE', *, *, #45830, .T. ) ;
#24179=DIRECTION ( 'NONE',  ( -0.000000000000000000, 0.5680647467311540355, -0.8229838658936575735 ) ) ;
#24181=DIRECTION ( 'NONE',  ( 0.000000000000000000, 5.319818659662208160E-15, -1.000000000000000000 ) ) ;
#24182=PLANE ( 'NONE',  #17408 ) ;
#24190=LINE ( 'NONE', #23414, #44708 ) ;
#24193=CARTESIAN_POINT ( 'NONE',  ( -330.4913330509368166, -63.50208336950359467, 0.4999999999999551470 ) ) ;
#24194=EDGE_LOOP ( 'NONE', ( #48591, #27497, #3189, #41816 ) ) ;
#24195=CIRCLE ( 'NONE', #6611, 60.00000000000000000 ) ;
#24196=VERTEX_POINT ( 'NONE', #37752 ) ;
#24204=CARTESIAN_POINT ( 'NONE',  ( 0.000000000000000000, -116.3883358649353141, 58.56982357178514320 ) ) ;
#24207=VECTOR ( 'NONE', #23664, 1000.000000000000000 ) ;
#24209=PLANE ( 'NONE',  #40715 ) ;
#24215=EDGE_CURVE ( 'NONE', #39946, #43466, #41050, .T. ) ;
#24216=DIRECTION ( 'NONE',  ( 0.000000000000000000, -0.7485107481711069655, -0.6631226582407885317 ) ) ;
#24219=VECTOR ( 'NONE', #28825, 1000.000000000000000 ) ;
#24221=CARTESIAN_POINT ( 'NONE',  ( -330.4913330509368166, -79.66942718702547666, -39.49849221029252533 ) ) ;
#24225=FACE_OUTER_BOUND ( 'NONE', #35438, .T. ) ;
#24226=ORIENTED_EDGE ( 'NONE', *, *, #9138, .F. ) ;
#24233=EDGE_LOOP ( 'NONE', ( #20911, #2841, #3500, #3526 ) ) ;
#24238=LINE ( 'NONE', #48417, #10629 ) ;
#24239=EDGE_CURVE ( 'NONE', #7213, #5675, #37493, .T. ) ;
#24241=DIRECTION ( 'NONE',  ( -1.000000000000000000, -2.497772389992478923E-15, 1.013386094502324929E-14 ) ) ;
#24245=CARTESIAN_POINT ( 'NONE',  ( -339.1964088526558498, -74.40671499923389831, 34.49419324804615172 ) ) ;
#24247=CARTESIAN_POINT ( 'NONE',  ( -339.1964088526558498, -167.9936954712150339, 38.74998146212178796 ) ) ;
#24249=AXIS2_PLACEMENT_3D ( 'NONE', #26776, #14698, #43065 ) ;
#24250=ORIENTED_EDGE ( 'NONE', *, *, #6916, .T. ) ;
#24257=EDGE_CURVE ( 'NONE', #1001, #43120, #25666, .T. ) ;
#24258=PLANE ( 'NONE',  #20804 ) ;
#24260=FACE_OUTER_BOUND ( 'NONE', #30746, .T. ) ;
#24261=EDGE_LOOP ( 'NONE', ( #29677, #41820, #43464, #46955 ) ) ;
#24263=ORIENTED_EDGE ( 'NONE', *, *, #5314, .T. ) ;
#24264=VECTOR ( 'NONE', #13299, 1000.000000000000000 ) ;
#24267=FACE_OUTER_BOUND ( 'NONE', #42385, .T. ) ;
#24268=CARTESIAN_POINT ( 'NONE',  ( -336.3521761649654422, -172.9832938399466684, -32.17247266903247294 ) ) ;
#24269=LINE ( 'NONE', #24002, #21377 ) ;
#24274=CARTESIAN_POINT ( 'NONE',  ( -336.3521761649654422, -182.2665742509934148, -5.491276508484069119 ) ) ;
#24279=PLANE ( 'NONE',  #7377 ) ;
#24288=CARTESIAN_POINT ( 'NONE',  ( -336.3521761649654422, -142.8954717479169574, 55.74477592174805096 ) ) ;
#24290=ORIENTED_EDGE ( 'NONE', *, *, #49583, .F. ) ;
#24294=CARTESIAN_POINT ( 'NONE',  ( -336.3521761649654422, -114.7679482383557144, 58.37307289257701370 ) ) ;
#24295=DIRECTION ( 'NONE',  ( -1.000000000000000000, -0.000000000000000000, 0.000000000000000000 ) ) ;
#24297=ADVANCED_FACE ( 'NONE', ( #18316 ), #10152, .F. ) ;
#24303=ORIENTED_EDGE ( 'NONE', *, *, #19516, .T. ) ;
#24308=EDGE_LOOP ( 'NONE', ( #44565, #39654, #32922, #35127 ) ) ;
#24311=CARTESIAN_POINT ( 'NONE',  ( -339.1964088526558498, -64.50000000000000000, -0.5000000000000457412 ) ) ;
#24314=AXIS2_PLACEMENT_3D ( 'NONE', #2530, #51407, #10406 ) ;
#24316=CARTESIAN_POINT ( 'NONE',  ( -330.4913330509368166, -123.5000000000000284, 0.000000000000000000 ) ) ;
#24317=ORIENTED_EDGE ( 'NONE', *, *, #47190, .T. ) ;
#24326=CARTESIAN_POINT ( 'NONE',  ( 0.000000000000000000, -150.9186671505826212, -52.24190551353930090 ) ) ;
#24327=LINE ( 'NONE', #4354, #4982 ) ;
#24328=FACE_BOUND ( 'NONE', #17180, .T. ) ;
#24341=CARTESIAN_POINT ( 'NONE',  ( -336.3521761649654422, -170.1129345408508868, -37.77875505479702412 ) ) ;
#24345=ORIENTED_EDGE ( 'NONE', *, *, #852, .F. ) ;
#24347=EDGE_LOOP ( 'NONE', ( #2788, #46637, #26354, #12640 ) ) ;
#24351=VECTOR ( 'NONE', #16837, 1000.000000000000000 ) ;
#24352=EDGE_CURVE ( 'NONE', #31195, #12905, #10932, .T. ) ;
#24361=DIRECTION ( 'NONE',  ( 1.000000000000000000, -0.000000000000000000, -0.000000000000000000 ) ) ;
#24369=ADVANCED_FACE ( 'NONE', ( #47725 ), #15923, .F. ) ;
#24370=ORIENTED_EDGE ( 'NONE', *, *, #34681, .F. ) ;
#24371=CARTESIAN_POINT ( 'NONE',  ( -336.3521761649654422, -126.1322888500942270, -59.00000000000001421 ) ) ;
#24373=ADVANCED_FACE ( 'NONE', ( #46682 ), #19088, .T. ) ;
#24389=DIRECTION ( 'NONE',  ( 0.000000000000000000, -0.5680647467311625842, -0.8229838658936516893 ) ) ;
#24390=DIRECTION ( 'NONE',  ( 0.000000000000000000, -0.1205366802553303196, -0.9927088740980530845 ) ) ;
#24402=CARTESIAN_POINT ( 'NONE',  ( -336.3521761649654422, -100.1170788342122080, 54.23253582808833073 ) ) ;
#24410=VECTOR ( 'NONE', #25984, 1000.000000000000000 ) ;
#24416=CARTESIAN_POINT ( 'NONE',  ( -336.3521761649654422, -78.25545813661345562, 37.90245108779119931 ) ) ;
#24432=ORIENTED_EDGE ( 'NONE', *, *, #33427, .F. ) ;
#24435=CARTESIAN_POINT ( 'NONE',  ( 0.000000000000000000, -178.6659583184393796, 20.92168833551003004 ) ) ;
#24440=DIRECTION ( 'NONE',  ( 0.000000000000000000, 0.000000000000000000, -1.000000000000000000 ) ) ;
#24445=CIRCLE ( 'NONE', #17645, 60.00000000000000000 ) ;
#24446=VERTEX_POINT ( 'NONE', #40849 ) ;
#24447=DIRECTION ( 'NONE',  ( -1.000000000000000000, -0.000000000000000000, 0.000000000000000000 ) ) ;
#24451=DIRECTION ( 'NONE',  ( -0.000000000000000000, 0.9927088740980526405, -0.1205366802553337890 ) ) ;
#24458=EDGE_CURVE ( 'NONE', #11058, #41322, #47449, .T. ) ;
#24463=DIRECTION ( 'NONE',  ( 0.000000000000000000, -6.846375318521798245E-14, -1.000000000000000000 ) ) ;
#24469=CARTESIAN_POINT ( 'NONE',  ( -330.4913330509368166, -116.8846903019851311, -58.63009191191288494 ) ) ;
#24474=VECTOR ( 'NONE', #50417, 1000.000000000000000 ) ;
#24484=PLANE ( 'NONE',  #9844 ) ;
#24485=AXIS2_PLACEMENT_3D ( 'NONE', #6922, #2971, #35039 ) ;
#24488=VECTOR ( 'NONE', #49358, 1000.000000000000000 ) ;
#24490=LINE ( 'NONE', #40509, #1242 ) ;
#24493=ORIENTED_EDGE ( 'NONE', *, *, #1663, .T. ) ;
#24494=CARTESIAN_POINT ( 'NONE',  ( 0.000000000000000000, -74.94395191227431496, -33.51582005713827783 ) ) ;
#24498=ORIENTED_EDGE ( 'NONE', *, *, #2145, .F. ) ;
#24502=CARTESIAN_POINT ( 'NONE',  ( -330.4913330509368166, -130.2355952558261549, 59.62073260661674112 ) ) ;
#24503=CARTESIAN_POINT ( 'NONE',  ( -336.3521761649654422, -174.5186198893880771, 29.74944317415823392 ) ) ;
#24504=CIRCLE ( 'NONE', #54, 60.00000000000000000 ) ;
#24507=AXIS2_PLACEMENT_3D ( 'NONE', #16294, #50443, #34139 ) ;
#24508=VERTEX_POINT ( 'NONE', #20626 ) ;
#24514=DIRECTION ( 'NONE',  ( 1.000000000000000000, 0.000000000000000000, -0.000000000000000000 ) ) ;
#24515=FACE_OUTER_BOUND ( 'NONE', #14758, .T. ) ;
#24516=ORIENTED_EDGE ( 'NONE', *, *, #17614, .T. ) ;
#24517=PLANE ( 'NONE',  #12939 ) ;
#24518=EDGE_CURVE ( 'NONE', #27048, #47761, #32715, .T. ) ;
#24519=DIRECTION ( 'NONE',  ( 1.000000000000000000, 0.000000000000000000, 0.000000000000000000 ) ) ;
#24523=VECTOR ( 'NONE', #31814, 1000.000000000000000 ) ;
#24525=ORIENTED_EDGE ( 'NONE', *, *, #21021, .T. ) ;
#24527=EDGE_CURVE ( 'NONE', #27120, #36746, #36389, .T. ) ;
#24528=ORIENTED_EDGE ( 'NONE', *, *, #47267, .F. ) ;
#24533=DIRECTION ( 'NONE',  ( 0.000000000000000000, -0.6631226582408017434, -0.7485107481710954191 ) ) ;
#24535=ADVANCED_FACE ( 'NONE', ( #12729 ), #4878, .F. ) ;
#24538=DIRECTION ( 'NONE',  ( -0.000000000000000000, 0.7485107481711089639, 0.6631226582407863113 ) ) ;
#24539=ORIENTED_EDGE ( 'NONE', *, *, #7338, .F. ) ;
#24542=LINE ( 'NONE', #20336, #42968 ) ;
#24543=EDGE_CURVE ( 'NONE', #13751, #6162, #20108, .T. ) ;
#24545=VECTOR ( 'NONE', #36229, 1000.000000000000114 ) ;
#24546=DIRECTION ( 'NONE',  ( -0.000000000000000000, 0.4647231720437664526, -0.8854560256532110207 ) ) ;
#24547=FACE_OUTER_BOUND ( 'NONE', #13660, .T. ) ;
#24550=AXIS2_PLACEMENT_3D ( 'NONE', #44936, #40984, #36512 ) ;
#24556=CARTESIAN_POINT ( 'NONE',  ( 0.000000000000000000, -182.0698235717851787, 7.111664135064491354 ) ) ;
#24559=LINE ( 'NONE', #48232, #9369 ) ;
#24560=AXIS2_PLACEMENT_3D ( 'NONE', #25163, #41175, #17278 ) ;
#24564=CIRCLE ( 'NONE', #17865, 60.00000000000000000 ) ;
#24571=EDGE_CURVE ( 'NONE', #26067, #9084, #32191, .T. ) ;
#24574=EDGE_LOOP ( 'NONE', ( #37694, #43020, #12840, #19057 ) ) ;
#24575=EDGE_LOOP ( 'NONE', ( #27183, #35398, #33190, #9384 ) ) ;
#24580=FACE_BOUND ( 'NONE', #23197, .T. ) ;
#24582=AXIS2_PLACEMENT_3D ( 'NONE', #16749, #13558, #49315 ) ;
#24583=ORIENTED_EDGE ( 'NONE', *, *, #6975, .F. ) ;
#24584=EDGE_CURVE ( 'NONE', #51089, #8376, #48237, .T. ) ;
#24585=EDGE_CURVE ( 'NONE', #6023, #11792, #30619, .T. ) ;
#24587=ORIENTED_EDGE ( 'NONE', *, *, #14379, .F. ) ;
#24590=ORIENTED_EDGE ( 'NONE', *, *, #26584, .T. ) ;
#24593=DIRECTION ( 'NONE',  ( 1.000000000000000000, -0.000000000000000000, -0.000000000000000000 ) ) ;
#24594=LINE ( 'NONE', #4627, #4418 ) ;
#24597=FACE_OUTER_BOUND ( 'NONE', #38821, .T. ) ;
#24599=ORIENTED_EDGE ( 'NONE', *, *, #11988, .T. ) ;
#24603=AXIS2_PLACEMENT_3D ( 'NONE', #46300, #45771, #9766 ) ;
#24604=LINE ( 'NONE', #16995, #30362 ) ;
#24606=CARTESIAN_POINT ( 'NONE',  ( -330.4913330509368166, -182.0095552316575152, 7.608018572113473432 ) ) ;
#24608=LINE ( 'NONE', #40621, #21201 ) ;
#24611=DIRECTION ( 'NONE',  ( 0.000000000000000000, 0.000000000000000000, -1.000000000000000000 ) ) ;
#24616=CARTESIAN_POINT ( 'NONE',  ( -330.4913330509368166, -66.09477493971897388, 13.63415328425216622 ) ) ;
#24619=DIRECTION ( 'NONE',  ( -0.000000000000000000, 0.000000000000000000, 1.000000000000000000 ) ) ;
#24626=CARTESIAN_POINT ( 'NONE',  ( -339.1964088526558498, -162.2499814621216672, -44.49369547121515467 ) ) ;
#24627=ORIENTED_EDGE ( 'NONE', *, *, #4956, .T. ) ;
#24637=ORIENTED_EDGE ( 'NONE', *, *, #1188, .F. ) ;
#24640=ADVANCED_FACE ( 'NONE', ( #45852 ), #50319, .F. ) ;
#24641=LINE ( 'NONE', #27617, #18618 ) ;
#24642=PLANE ( 'NONE',  #43951 ) ;
#24653=DIRECTION ( 'NONE',  ( -0.000000000000000000, -0.5680647467311596976, -0.8229838658936536877 ) ) ;
#24656=VECTOR ( 'NONE', #22812, 1000.000000000000000 ) ;
#24659=DIRECTION ( 'NONE',  ( -0.000000000000000000, 0.9927088740980538617, -0.1205366802553232974 ) ) ;
#24661=ORIENTED_EDGE ( 'NONE', *, *, #48090, .T. ) ;
#24663=DIRECTION ( 'NONE',  ( 0.000000000000000000, 0.1205366802553199113, -0.9927088740980544168 ) ) ;
#24667=CARTESIAN_POINT ( 'NONE',  ( -336.3521761649654422, -181.7525362123217292, 9.724760635742144999 ) ) ;
#24669=DIRECTION ( 'NONE',  ( 0.000000000000000000, -0.5680647467311510379, 0.8229838658936596829 ) ) ;
#24671=DIRECTION ( 'NONE',  ( -0.000000000000000000, -0.1205366802553164696, 0.9927088740980548609 ) ) ;
#24676=LINE ( 'NONE', #39650, #6185 ) ;
#24678=CARTESIAN_POINT ( 'NONE',  ( -339.1964088526558498, -84.75001853787875916, -44.49369547121548862 ) ) ;
#24683=DIRECTION ( 'NONE',  ( -0.000000000000000000, 0.7485107481710999711, -0.6631226582407964143 ) ) ;
#24687=ORIENTED_EDGE ( 'NONE', *, *, #7006, .T. ) ;
#24693=VECTOR ( 'NONE', #21889, 1000.000000000000000 ) ;
#24694=ORIENTED_EDGE ( 'NONE', *, *, #37666, .T. ) ;
#24696=ADVANCED_FACE ( 'NONE', ( #26116 ), #37950, .T. ) ;
#24699=DIRECTION ( 'NONE',  ( 1.000000000000000000, -0.000000000000000000, -0.000000000000000000 ) ) ;
#24702=ORIENTED_EDGE ( 'NONE', *, *, #1158, .F. ) ;
#24704=EDGE_CURVE ( 'NONE', #22194, #27513, #29805, .T. ) ;
#24706=ORIENTED_EDGE ( 'NONE', *, *, #7669, .T. ) ;
#24707=ORIENTED_EDGE ( 'NONE', *, *, #6695, .T. ) ;
#24711=ADVANCED_FACE ( 'NONE', ( #46895 ), #38970, .F. ) ;
#24713=ADVANCED_FACE ( 'NONE', ( #10872 ), #23727, .T. ) ;
#24714=CARTESIAN_POINT ( 'NONE',  ( -339.1964088526558498, -96.52406086224443982, -52.47426709956138069 ) ) ;
#24719=VERTEX_POINT ( 'NONE', #26890 ) ;
#24721=CARTESIAN_POINT ( 'NONE',  ( -339.1964088526558498, -90.39567187580880159, -48.84008046109142498 ) ) ;
#24722=ORIENTED_EDGE ( 'NONE', *, *, #12161, .F. ) ;
#24740=VECTOR ( 'NONE', #12401, 1000.000000000000000 ) ;
#24754=VECTOR ( 'NONE', #42356, 1000.000000000000000 ) ;
#24756=FACE_OUTER_BOUND ( 'NONE', #9172, .T. ) ;
#24758=DIRECTION ( 'NONE',  ( 0.000000000000000000, 0.000000000000000000, 1.000000000000000000 ) ) ;
#24767=ORIENTED_EDGE ( 'NONE', *, *, #42903, .T. ) ;
#24773=ORIENTED_EDGE ( 'NONE', *, *, #41611, .F. ) ;
#24780=EDGE_CURVE ( 'NONE', #21924, #13387, #47392, .T. ) ;
#24781=DIRECTION ( 'NONE',  ( 0.000000000000000000, 0.8854560256532126861, 0.4647231720437631775 ) ) ;
#24786=ORIENTED_EDGE ( 'NONE', *, *, #11476, .F. ) ;
#24788=AXIS2_PLACEMENT_3D ( 'NONE', #39950, #47869, #11842 ) ;
#24794=ORIENTED_EDGE ( 'NONE', *, *, #35670, .T. ) ;
#24801=FACE_BOUND ( 'NONE', #36479, .T. ) ;
#24805=ORIENTED_EDGE ( 'NONE', *, *, #7609, .T. ) ;
#24806=CARTESIAN_POINT ( 'NONE',  ( -305.0000000000000568, -91.61526299123897843, -50.82679948493848343 ) ) ;
#24812=CARTESIAN_POINT ( 'NONE',  ( -330.4913330509368166, -178.4886558749180949, 21.38919645685269444 ) ) ;
#24822=ORIENTED_EDGE ( 'NONE', *, *, #35175, .F. ) ;
#24830=ORIENTED_EDGE ( 'NONE', *, *, #51726, .T. ) ;
#24835=LINE ( 'NONE', #16445, #23559 ) ;
#24836=CARTESIAN_POINT ( 'NONE',  ( -336.3521761649654422, -75.87119766449505676, -34.85916744524372746 ) ) ;
#24837=VERTEX_POINT ( 'NONE', #15595 ) ;
#24838=ORIENTED_EDGE ( 'NONE', *, *, #48029, .F. ) ;
#24848=CARTESIAN_POINT ( 'NONE',  ( -336.3521761649654422, -174.5186198893880771, 29.74944317415823392 ) ) ;
#24851=ORIENTED_EDGE ( 'NONE', *, *, #10521, .F. ) ;
#24852=CARTESIAN_POINT ( 'NONE',  ( -305.0000000000000568, -64.31210272782786319, -9.838334030657643225 ) ) ;
#24855=DIRECTION ( 'NONE',  ( 0.000000000000000000, 0.9350162426854146114, -0.3546048870425363986 ) ) ;
#24856=AXIS2_PLACEMENT_3D ( 'NONE', #40232, #11616, #23691 ) ;
#24863=LINE ( 'NONE', #36695, #13260 ) ;
#24864=VECTOR ( 'NONE', #29442, 1000.000000000000000 ) ;
#24868=LINE ( 'NONE', #25392, #3575 ) ;
#24873=PLANE ( 'NONE',  #13914 ) ;
#24880=CARTESIAN_POINT ( 'NONE',  ( -330.4913330509368166, -123.5000000000000284, 0.000000000000000000 ) ) ;
#24884=AXIS2_PLACEMENT_3D ( 'NONE', #19631, #34623, #43289 ) ;
#24887=VECTOR ( 'NONE', #39146, 1000.000000000000000 ) ;
#24889=VERTEX_POINT ( 'NONE', #33381 ) ;
#24890=LINE ( 'NONE', #13050, #48103 ) ;
#24895=AXIS2_PLACEMENT_3D ( 'NONE', #39767, #11146, #27172 ) ;
#24896=EDGE_CURVE ( 'NONE', #30672, #30972, #42415, .T. ) ;
#24898=AXIS2_PLACEMENT_3D ( 'NONE', #14728, #35202, #10264 ) ;
#24901=VECTOR ( 'NONE', #28357, 1000.000000000000114 ) ;
#24905=PLANE ( 'NONE',  #32754 ) ;
#24908=ORIENTED_EDGE ( 'NONE', *, *, #2799, .T. ) ;
#24912=EDGE_LOOP ( 'NONE', ( #41561, #8322, #49483, #15094 ) ) ;
#24917=PLANE ( 'NONE',  #51699 ) ;
#24921=ORIENTED_EDGE ( 'NONE', *, *, #29821, .F. ) ;
#24922=AXIS2_PLACEMENT_3D ( 'NONE', #15385, #27188, #39015 ) ;
#24925=CARTESIAN_POINT ( 'NONE',  ( -330.4913330509368166, -90.39567187580801999, 48.84008046109089918 ) ) ;
#24927=FACE_OUTER_BOUND ( 'NONE', #6837, .T. ) ;
#24928=ORIENTED_EDGE ( 'NONE', *, *, #19407, .F. ) ;
#24930=CARTESIAN_POINT ( 'NONE',  ( -330.4913330509368166, -180.9052250602807703, 13.63415328425337236 ) ) ;
#24934=ORIENTED_EDGE ( 'NONE', *, *, #15985, .T. ) ;
#24935=ORIENTED_EDGE ( 'NONE', *, *, #46256, .T. ) ;
#24939=AXIS2_PLACEMENT_3D ( 'NONE', #50774, #2670, #19723 ) ;
#24940=DIRECTION ( 'NONE',  ( 0.000000000000000000, -0.7485107481710934207, 0.6631226582408039638 ) ) ;
#24943=VECTOR ( 'NONE', #13607, 1000.000000000000000 ) ;
#24946=ADVANCED_FACE ( 'NONE', ( #24977 ), #21285, .F. ) ;
#24952=CARTESIAN_POINT ( 'NONE',  ( -339.1964088526558498, -175.9742670995615015, -26.97593913775538965 ) ) ;
#24958=LINE ( 'NONE', #9701, #48930 ) ;
#24962=EDGE_LOOP ( 'NONE', ( #36264, #18441, #32800, #3804 ) ) ;
#24969=DIRECTION ( 'NONE',  ( 1.000000000000000000, -0.000000000000000000, -0.000000000000000000 ) ) ;
#24973=ORIENTED_EDGE ( 'NONE', *, *, #45415, .F. ) ;
#24977=FACE_OUTER_BOUND ( 'NONE', #48733, .T. ) ;
#24980=AXIS2_PLACEMENT_3D ( 'NONE', #23739, #19792, #23997 ) ;
#24982=VERTEX_POINT ( 'NONE', #4740 ) ;
#24984=AXIS2_PLACEMENT_3D ( 'NONE', #30658, #37778, #30933 ) ;
#24990=CARTESIAN_POINT ( 'NONE',  ( -332.3517673607765914, -178.0871407151310279, 22.44790492310219676 ) ) ;
#24992=CARTESIAN_POINT ( 'NONE',  ( -336.3521761649654422, -68.91285928486892942, -22.44790492310182017 ) ) ;
#24996=ORIENTED_EDGE ( 'NONE', *, *, #22999, .T. ) ;
#24997=CARTESIAN_POINT ( 'NONE',  ( -339.1964088526558498, -66.09477493971894546, 13.63415328425207917 ) ) ;
#25000=ORIENTED_EDGE ( 'NONE', *, *, #43627, .F. ) ;
#25002=CARTESIAN_POINT ( 'NONE',  ( -330.4913330509368166, -144.3080463282022663, -56.27632902032068785 ) ) ;
#25008=DIRECTION ( 'NONE',  ( -1.000000000000000000, 0.000000000000000000, 0.000000000000000000 ) ) ;
#25011=CARTESIAN_POINT ( 'NONE',  ( -336.3521761649654422, -64.50000000000000000, -2.632288850093980503 ) ) ;
#25013=EDGE_CURVE ( 'NONE', #35455, #12928, #49146, .T. ) ;
#25016=DIRECTION ( 'NONE',  ( -0.000000000000000000, 0.6631226582408016323, 0.7485107481710953081 ) ) ;
#25021=CARTESIAN_POINT ( 'NONE',  ( -336.3521761649654422, -120.8677111499054320, 59.00000000000000000 ) ) ;
#25022=EDGE_CURVE ( 'NONE', #50532, #37883, #1299, .T. ) ;
#25026=FACE_OUTER_BOUND ( 'NONE', #888, .T. ) ;
#25028=EDGE_CURVE ( 'NONE', #33448, #32690, #22056, .T. ) ;
#25030=VECTOR ( 'NONE', #10239, 1000.000000000000000 ) ;
#25034=PLANE ( 'NONE',  #30370 ) ;
#25036=EDGE_CURVE ( 'NONE', #47279, #47521, #38598, .T. ) ;
#25038=CARTESIAN_POINT ( 'NONE',  ( -339.1964088526558498, -78.25935320507949200, -39.41172259083896279 ) ) ;
#25041=EDGE_LOOP ( 'NONE', ( #39071, #2951, #47790, #7697 ) ) ;
#25043=ORIENTED_EDGE ( 'NONE', *, *, #46719, .F. ) ;
#25046=CARTESIAN_POINT ( 'NONE',  ( -330.4913330509368166, -74.65991953890832633, 33.10432812419081472 ) ) ;
#25047=VECTOR ( 'NONE', #50512, 1000.000000000000114 ) ;
#25058=ORIENTED_EDGE ( 'NONE', *, *, #12540, .F. ) ;
#25059=LINE ( 'NONE', #41065, #33921 ) ;
#25072=ADVANCED_FACE ( 'NONE', ( #10478 ), #2074, .F. ) ;
#25073=ADVANCED_FACE ( 'NONE', ( #42275 ), #26507, .F. ) ;
#25075=DIRECTION ( 'NONE',  ( 1.000000000000000000, 0.000000000000000000, 0.000000000000000000 ) ) ;
#25078=EDGE_CURVE ( 'NONE', #13689, #28174, #16433, .T. ) ;
#25082=VECTOR ( 'NONE', #50863, 1000.000000000000000 ) ;
#25085=DIRECTION ( 'NONE',  ( 0.000000000000000000, 0.8229838658936536877, -0.5680647467311596976 ) ) ;
#25088=DIRECTION ( 'NONE',  ( -0.000000000000000000, -0.9350162426854121689, 0.3546048870425426158 ) ) ;
#25101=ORIENTED_EDGE ( 'NONE', *, *, #36441, .F. ) ;
#25103=EDGE_CURVE ( 'NONE', #45420, #50591, #49054, .T. ) ;
#25110=DIRECTION ( 'NONE',  ( 1.000000000000000000, 0.000000000000000000, -0.000000000000000000 ) ) ;
#25112=DIRECTION ( 'NONE',  ( -0.000000000000000000, 0.000000000000000000, 1.000000000000000000 ) ) ;
#25113=CARTESIAN_POINT ( 'NONE',  ( -330.4913330509368166, -123.5000000000000284, 0.000000000000000000 ) ) ;
#25114=EDGE_LOOP ( 'NONE', ( #23876, #48697 ) ) ;
#25119=VECTOR ( 'NONE', #47271, 1000.000000000000000 ) ;
#25120=CARTESIAN_POINT ( 'NONE',  ( -330.4913330509368166, -178.4886558749180949, 21.38919645685269444 ) ) ;
#25121=FACE_BOUND ( 'NONE', #11349, .T. ) ;
#25130=CARTESIAN_POINT ( 'NONE',  ( -339.1964088526558498, -123.5000000000000284, 0.000000000000000000 ) ) ;
#25132=DIRECTION ( 'NONE',  ( -1.000000000000000000, 0.000000000000000000, 0.000000000000000000 ) ) ;
#25133=EDGE_CURVE ( 'NONE', #29857, #27624, #6373, .T. ) ;
#25139=ORIENTED_EDGE ( 'NONE', *, *, #47731, .F. ) ;
#25140=DIRECTION ( 'NONE',  ( 1.000000000000000000, -0.000000000000000000, 0.000000000000000000 ) ) ;
#25143=CARTESIAN_POINT ( 'NONE',  ( -339.1964088526558498, -182.1300919119129560, -6.615309698014600670 ) ) ;
#25148=DIRECTION ( 'NONE',  ( 1.000000000000000000, 0.000000000000000000, 0.000000000000000000 ) ) ;
#25154=PLANE ( 'NONE',  #39869 ) ;
#25158=EDGE_LOOP ( 'NONE', ( #51667, #40336, #45138, #36337 ) ) ;
#25163=CARTESIAN_POINT ( 'NONE',  ( -336.3521761649654422, -176.9651911376907094, -25.08789112700655721 ) ) ;
#25167=ORIENTED_EDGE ( 'NONE', *, *, #6449, .T. ) ;
#25169=AXIS2_PLACEMENT_3D ( 'NONE', #24326, #47985, #19355 ) ;
#25171=CARTESIAN_POINT ( 'NONE',  ( -336.3521761649654422, -181.8730728925770563, 8.732051761644092025 ) ) ;
#25173=ORIENTED_EDGE ( 'NONE', *, *, #6799, .T. ) ;
#25175=CARTESIAN_POINT ( 'NONE',  ( -305.0000000000000568, -183.1207326066167127, -6.735595255826561711 ) ) ;
#25176=LINE ( 'NONE', #13075, #42296 ) ;
#25177=ORIENTED_EDGE ( 'NONE', *, *, #17338, .F. ) ;
#25181=ORIENTED_EDGE ( 'NONE', *, *, #2231, .F. ) ;
#25184=ORIENTED_EDGE ( 'NONE', *, *, #32273, .T. ) ;
#25187=CARTESIAN_POINT ( 'NONE',  ( -339.1964088526558498, -84.75001853787809125, 44.49369547121489887 ) ) ;
#25188=ORIENTED_EDGE ( 'NONE', *, *, #42692, .F. ) ;
#25191=CARTESIAN_POINT ( 'NONE',  ( -332.3517673607765914, -65.12692710742291524, -8.732051761643681687 ) ) ;
#25194=ORIENTED_EDGE ( 'NONE', *, *, #36160, .F. ) ;
#25196=ORIENTED_EDGE ( 'NONE', *, *, #41256, .F. ) ;
#25200=PLANE ( 'NONE',  #45749 ) ;
#25202=DIRECTION ( 'NONE',  ( -0.000000000000000000, -0.8229838658936596829, -0.5680647467311510379 ) ) ;
#25203=VERTEX_POINT ( 'NONE', #36961 ) ;
#25204=CARTESIAN_POINT ( 'NONE',  ( -305.0000000000000568, -145.2430625708868206, 55.92172413327848801 ) ) ;
#25206=DIRECTION ( 'NONE',  ( 0.000000000000000000, 0.000000000000000000, 1.000000000000000000 ) ) ;
#25207=DIRECTION ( 'NONE',  ( -0.000000000000000000, 0.3546048870425331789, -0.9350162426854158326 ) ) ;
#25208=CARTESIAN_POINT ( 'NONE',  ( -365.0000000000001137, -168.5000000000000284, 0.000000000000000000 ) ) ;
#25209=CARTESIAN_POINT ( 'NONE',  ( -305.0000000000000568, -144.3080463282017263, 56.27632902032089390 ) ) ;
#25210=CIRCLE ( 'NONE', #14292, 60.00000000000000000 ) ;
#25211=VECTOR ( 'NONE', #5574, 1000.000000000000000 ) ;
#25215=DIRECTION ( 'NONE',  ( 0.000000000000000000, -0.1205366802553130001, 0.9927088740980553050 ) ) ;
#25216=DIRECTION ( 'NONE',  ( -0.000000000000000000, -0.4647231720437724478, -0.8854560256532078011 ) ) ;
#25218=DIRECTION ( 'NONE',  ( 0.000000000000000000, -0.2393156642875516604, 0.9709418174260535661 ) ) ;
#25221=VECTOR ( 'NONE', #20964, 1000.000000000000000 ) ;
#25226=PLANE ( 'NONE',  #24145 ) ;
#25227=PLANE ( 'NONE',  #17660 ) ;
#25231=ORIENTED_EDGE ( 'NONE', *, *, #15429, .T. ) ;
#25233=ADVANCED_FACE ( 'NONE', ( #12769 ), #24873, .F. ) ;
#25238=LINE ( 'NONE', #17107, #2582 ) ;
#25240=DIRECTION ( 'NONE',  ( -0.000000000000000000, 0.8229838658936634577, 0.5680647467311457088 ) ) ;
#25242=EDGE_LOOP ( 'NONE', ( #11061, #24157, #35624, #44184 ) ) ;
#25243=CARTESIAN_POINT ( 'NONE',  ( -330.4913330509368166, -123.5000000000000284, 0.000000000000000000 ) ) ;
#25247=ORIENTED_EDGE ( 'NONE', *, *, #1081, .T. ) ;
#25250=CARTESIAN_POINT ( 'NONE',  ( -339.1964088526558498, -68.51134412508150717, 21.38919645685156112 ) ) ;
#25251=DIRECTION ( 'NONE',  ( -1.000000000000000000, -0.000000000000000000, 0.000000000000000000 ) ) ;
#25253=VERTEX_POINT ( 'NONE', #706 ) ;
#25259=VECTOR ( 'NONE', #27993, 1000.000000000000000 ) ;
#25262=CARTESIAN_POINT ( 'NONE',  ( -336.3521761649654422, -111.9361751271348879, -57.91551518289410438 ) ) ;
#25273=AXIS2_PLACEMENT_3D ( 'NONE', #22877, #11288, #43374 ) ;
#25275=DIRECTION ( 'NONE',  ( 0.000000000000000000, 0.000000000000000000, -1.000000000000000000 ) ) ;
#25279=CARTESIAN_POINT ( 'NONE',  ( -336.3521761649654422, -169.4076645216271402, -37.15394033962039089 ) ) ;
#25287=ORIENTED_EDGE ( 'NONE', *, *, #45162, .T. ) ;
#25289=VERTEX_POINT ( 'NONE', #5175 ) ;
#25295=DIRECTION ( 'NONE',  ( 0.000000000000000000, 0.000000000000000000, -1.000000000000000000 ) ) ;
#25300=ADVANCED_FACE ( 'NONE', ( #21965 ), #38754, .F. ) ;
#25302=DIRECTION ( 'NONE',  ( 0.000000000000000000, -1.066276696567077385E-13, -1.000000000000000000 ) ) ;
#25305=AXIS2_PLACEMENT_3D ( 'NONE', #24880, #20948, #9628 ) ;
#25310=VECTOR ( 'NONE', #6472, 1000.000000000000000 ) ;
#25311=FACE_OUTER_BOUND ( 'NONE', #29963, .T. ) ;
#25318=DIRECTION ( 'NONE',  ( 1.000000000000000000, -0.000000000000000000, -0.000000000000000000 ) ) ;
#25319=ORIENTED_EDGE ( 'NONE', *, *, #43981, .F. ) ;
#25320=DIRECTION ( 'NONE',  ( 0.000000000000000000, -0.9350162426854194964, -0.3546048870425235200 ) ) ;
#25323=FACE_BOUND ( 'NONE', #49758, .T. ) ;
#25325=LINE ( 'NONE', #45052, #23124 ) ;
#25333=DIRECTION ( 'NONE',  ( 1.000000000000000000, -0.000000000000000000, -0.000000000000000000 ) ) ;
#25334=DIRECTION ( 'NONE',  ( 1.043714542225393697E-14, 0.9927088740980527515, -0.1205366802553337890 ) ) ;
#25335=CARTESIAN_POINT ( 'NONE',  ( -332.3517673607765914, -82.40546666720629787, 42.41660376256258047 ) ) ;
#25340=ORIENTED_EDGE ( 'NONE', *, *, #31143, .T. ) ;
#25342=DIRECTION ( 'NONE',  ( -0.9993908270190956511, 0.000000000000000000, 0.03489949670250096919 ) ) ;
#25361=EDGE_LOOP ( 'NONE', ( #30025, #38046, #7829, #51474 ) ) ;
#25366=LINE ( 'NONE', #1449, #2278 ) ;
#25370=DIRECTION ( 'NONE',  ( 1.000000000000000000, -0.000000000000000000, -0.000000000000000000 ) ) ;
#25374=EDGE_CURVE ( 'NONE', #38762, #30320, #47707, .T. ) ;
#25375=ORIENTED_EDGE ( 'NONE', *, *, #40547, .F. ) ;
#25379=EDGE_CURVE ( 'NONE', #5922, #26098, #27709, .T. ) ;
#25380=CARTESIAN_POINT ( 'NONE',  ( -332.3517673607765914, -173.5513585866778214, -31.34948880313881503 ) ) ;
#25383=CARTESIAN_POINT ( 'NONE',  ( -332.3517673607765914, -183.2372378732723632, -5.609136410542877371 ) ) ;
#25385=FACE_OUTER_BOUND ( 'NONE', #15692, .T. ) ;
#25392=CARTESIAN_POINT ( 'NONE',  ( -330.4913330509368166, -109.8658467157472813, -57.40522506028090532 ) ) ;
#25396=DIRECTION ( 'NONE',  ( 0.000000000000000000, -0.5680647467311540355, 0.8229838658936575735 ) ) ;
#25403=PLANE ( 'NONE',  #3461 ) ;
#25414=CARTESIAN_POINT ( 'NONE',  ( -336.3521761649654422, -91.32752733096738496, -49.48329383994654052 ) ) ;
#25415=FACE_OUTER_BOUND ( 'NONE', #24575, .T. ) ;
#25418=EDGE_CURVE ( 'NONE', #37409, #1436, #18971, .T. ) ;
#25424=LINE ( 'NONE', #25171, #20895 ) ;
#25426=ORIENTED_EDGE ( 'NONE', *, *, #49119, .F. ) ;
#25429=DIRECTION ( 'NONE',  ( 1.000000000000000000, -0.000000000000000000, -0.000000000000000000 ) ) ;
#25433=LINE ( 'NONE', #21490, #6624 ) ;
#25434=CARTESIAN_POINT ( 'NONE',  ( -332.3517673607765914, -123.5000000000000284, 0.000000000000000000 ) ) ;
#25435=ORIENTED_EDGE ( 'NONE', *, *, #22931, .F. ) ;
#25439=ORIENTED_EDGE ( 'NONE', *, *, #31929, .F. ) ;
#25441=VERTEX_POINT ( 'NONE', #31913 ) ;
#25442=DIRECTION ( 'NONE',  ( 0.000000000000000000, 0.000000000000000000, 1.000000000000000000 ) ) ;
#25444=ORIENTED_EDGE ( 'NONE', *, *, #14421, .F. ) ;
#25449=LINE ( 'NONE', #46211, #23320 ) ;
#25452=EDGE_LOOP ( 'NONE', ( #23903, #16106, #17827, #5022 ) ) ;
#25453=DIRECTION ( 'NONE',  ( 1.000000000000000000, -0.000000000000000000, -0.000000000000000000 ) ) ;
#25454=DIRECTION ( 'NONE',  ( 1.000000000000000000, 0.000000000000000000, -0.000000000000000000 ) ) ;
#25463=DIRECTION ( 'NONE',  ( -1.000000000000000000, -7.812315528781888245E-15, -6.921107616850760573E-15 ) ) ;
#25466=ORIENTED_EDGE ( 'NONE', *, *, #17338, .T. ) ;
#25468=CARTESIAN_POINT ( 'NONE',  ( -336.3521761649654422, -64.73342574900661361, 5.491276508483657892 ) ) ;
#25475=DIRECTION ( 'NONE',  ( -0.000000000000000000, 0.8854560256532093554, -0.4647231720437695057 ) ) ;
#25476=FACE_OUTER_BOUND ( 'NONE', #15674, .T. ) ;
#25480=LINE ( 'NONE', #15470, #31092 ) ;
#25485=ADVANCED_FACE ( 'NONE', ( #44272 ), #8263, .F. ) ;
#25488=AXIS2_PLACEMENT_3D ( 'NONE', #48342, #40433, #4452 ) ;
#25489=ORIENTED_EDGE ( 'NONE', *, *, #41387, .F. ) ;
#25492=CARTESIAN_POINT ( 'NONE',  ( 0.000000000000000000, -64.93017642821470758, 7.111664135063263892 ) ) ;
#25495=CARTESIAN_POINT ( 'NONE',  ( -365.0000000000001137, -168.5000000000000284, -5.000000000000001776 ) ) ;
#25496=ORIENTED_EDGE ( 'NONE', *, *, #23840, .F. ) ;
#25497=EDGE_CURVE ( 'NONE', #11938, #22244, #40303, .T. ) ;
#25498=LINE ( 'NONE', #41515, #45770 ) ;
#25499=ORIENTED_EDGE ( 'NONE', *, *, #40643, .F. ) ;
#25503=DIRECTION ( 'NONE',  ( -1.000000000000000000, -4.850383327711889945E-15, 9.241633304753590273E-15 ) ) ;
#25505=ORIENTED_EDGE ( 'NONE', *, *, #29462, .T. ) ;
#25513=LINE ( 'NONE', #5560, #2245 ) ;
#25516=ORIENTED_EDGE ( 'NONE', *, *, #12422, .T. ) ;
#25527=CIRCLE ( 'NONE', #47334, 60.00000000000000000 ) ;
#25528=LINE ( 'NONE', #33677, #2771 ) ;
#25530=DIRECTION ( 'NONE',  ( 0.000000000000000000, 0.000000000000000000, 1.000000000000000000 ) ) ;
#25531=DIRECTION ( 'NONE',  ( -1.000000000000000000, 0.000000000000000000, 0.000000000000000000 ) ) ;
#25532=LINE ( 'NONE', #29727, #32918 ) ;
#25534=ORIENTED_EDGE ( 'NONE', *, *, #4956, .F. ) ;
#25537=AXIS2_PLACEMENT_3D ( 'NONE', #17754, #40598, #32979 ) ;
#25538=ADVANCED_FACE ( 'NONE', ( #5369 ), #17194, .T. ) ;
#25546=LINE ( 'NONE', #49995, #23591 ) ;
#25556=ORIENTED_EDGE ( 'NONE', *, *, #41539, .F. ) ;
#25557=CARTESIAN_POINT ( 'NONE',  ( -336.3521761649654422, -127.9985676343858501, 58.88711093124869222 ) ) ;
#25562=ORIENTED_EDGE ( 'NONE', *, *, #47853, .F. ) ;
#25572=PLANE ( 'NONE',  #24083 ) ;
#25573=ORIENTED_EDGE ( 'NONE', *, *, #8282, .F. ) ;
#25581=EDGE_CURVE ( 'NONE', #1746, #7213, #39916, .T. ) ;
#25582=LINE ( 'NONE', #17725, #10628 ) ;
#25585=ORIENTED_EDGE ( 'NONE', *, *, #46229, .F. ) ;
#25595=EDGE_CURVE ( 'NONE', #32525, #41934, #5640, .T. ) ;
#25596=VECTOR ( 'NONE', #34883, 999.9999999999998863 ) ;
#25602=AXIS2_PLACEMENT_3D ( 'NONE', #4686, #20712, #36748 ) ;
#25603=ORIENTED_EDGE ( 'NONE', *, *, #10816, .T. ) ;
#25605=CARTESIAN_POINT ( 'NONE',  ( -336.3521761649653854, -171.9335100611925213, 35.41461708323791413 ) ) ;
#25609=CIRCLE ( 'NONE', #18081, 60.00000000000000000 ) ;
#25610=DIRECTION ( 'NONE',  ( -1.000000000000000000, -0.000000000000000000, -0.000000000000000000 ) ) ;
#25611=ORIENTED_EDGE ( 'NONE', *, *, #4486, .F. ) ;
#25615=CARTESIAN_POINT ( 'NONE',  ( -330.4913330509368166, -131.2283041299249362, -59.50019592636134291 ) ) ;
#25622=ORIENTED_EDGE ( 'NONE', *, *, #42303, .F. ) ;
#25623=ORIENTED_EDGE ( 'NONE', *, *, #16284, .F. ) ;
#25624=AXIS2_PLACEMENT_3D ( 'NONE', #33426, #49705, #45260 ) ;
#25626=DIRECTION ( 'NONE',  ( 0.000000000000000000, -0.3546048870425396182, -0.9350162426854132791 ) ) ;
#25632=CARTESIAN_POINT ( 'NONE',  ( -336.3521761649654422, -123.5000000000000284, 0.000000000000000000 ) ) ;
#25638=LINE ( 'NONE', #34310, #13565 ) ;
#25642=ADVANCED_FACE ( 'NONE', ( #45064 ), #1143, .F. ) ;
#25647=EDGE_CURVE ( 'NONE', #46182, #42588, #9560, .T. ) ;
#25648=AXIS2_PLACEMENT_3D ( 'NONE', #26675, #50592, #42705 ) ;
#25649=PLANE ( 'NONE',  #28243 ) ;
#25659=DIRECTION ( 'NONE',  ( 0.000000000000000000, 0.000000000000000000, -1.000000000000000000 ) ) ;
#25660=EDGE_CURVE ( 'NONE', #21253, #33963, #38450, .T. ) ;
#25664=VECTOR ( 'NONE', #3408, 1000.000000000000000 ) ;
#25665=EDGE_CURVE ( 'NONE', #32381, #20194, #2458, .T. ) ;
#25666=LINE ( 'NONE', #25414, #23433 ) ;
#25667=CARTESIAN_POINT ( 'NONE',  ( -305.0000000000000568, -67.22367097967905636, 20.80804632820150957 ) ) ;
#25668=ORIENTED_EDGE ( 'NONE', *, *, #37092, .T. ) ;
#25669=AXIS2_PLACEMENT_3D ( 'NONE', #13949, #29975, #34680 ) ;
#25671=EDGE_CURVE ( 'NONE', #12665, #20473, #2191, .T. ) ;
#25673=ORIENTED_EDGE ( 'NONE', *, *, #19483, .T. ) ;
#25677=CARTESIAN_POINT ( 'NONE',  ( -340.0000000000000568, -63.50000000000002842, 0.000000000000000000 ) ) ;
#25690=CARTESIAN_POINT ( 'NONE',  ( 0.000000000000000000, -89.98417994286123189, 48.55604808772534398 ) ) ;
#25691=DIRECTION ( 'NONE',  ( -1.000000000000000000, -0.000000000000000000, -0.000000000000000000 ) ) ;
#25692=ORIENTED_EDGE ( 'NONE', *, *, #20184, .T. ) ;
#25697=CARTESIAN_POINT ( 'NONE',  ( -336.3521761649654422, -81.78065195202964333, 43.12187378178631292 ) ) ;
#25698=DIRECTION ( 'NONE',  ( 0.000000000000000000, 0.2393156642875685913, 0.9709418174260493473 ) ) ;
#25701=CARTESIAN_POINT ( 'NONE',  ( -330.4913330509368166, -66.33409060400670398, -14.60509510167892522 ) ) ;
#25702=ORIENTED_EDGE ( 'NONE', *, *, #46223, .T. ) ;
#25706=DIRECTION ( 'NONE',  ( 0.000000000000000000, 0.8229838658936633466, 0.5680647467311457088 ) ) ;
#25708=LINE ( 'NONE', #4848, #7945 ) ;
#25710=CARTESIAN_POINT ( 'NONE',  ( -336.3521761649653854, -181.3443148879387081, 15.93848283698911317 ) ) ;
#25711=ORIENTED_EDGE ( 'NONE', *, *, #25078, .T. ) ;
#25715=EDGE_CURVE ( 'NONE', #10873, #76, #1936, .T. ) ;
#25716=ADVANCED_FACE ( 'NONE', ( #5896 ), #17975, .T. ) ;
#25719=EDGE_LOOP ( 'NONE', ( #1744, #16059, #19588, #35067 ) ) ;
#25720=DIRECTION ( 'NONE',  ( 0.000000000000000000, 0.9709418174260526779, 0.2393156642875547968 ) ) ;
#25728=AXIS2_PLACEMENT_3D ( 'NONE', #44766, #4830, #7971 ) ;
#25736=AXIS2_PLACEMENT_3D ( 'NONE', #23443, #30285, #42883 ) ;
#25737=CARTESIAN_POINT ( 'NONE',  ( -339.1964088526558498, -89.00580675195338642, -49.09328500076576773 ) ) ;
#25741=DIRECTION ( 'NONE',  ( 1.000000000000000000, -0.000000000000000000, -0.000000000000000000 ) ) ;
#25747=EDGE_LOOP ( 'NONE', ( #38561, #11788, #25811, #11335 ) ) ;
#25755=CARTESIAN_POINT ( 'NONE',  ( -332.3517673607765914, -165.9166037625627439, 41.09453333279358134 ) ) ;
#25760=ORIENTED_EDGE ( 'NONE', *, *, #50363, .T. ) ;
#25762=AXIS2_PLACEMENT_3D ( 'NONE', #46328, #10314, #22145 ) ;
#25765=ORIENTED_EDGE ( 'NONE', *, *, #8061, .T. ) ;
#25769=DIRECTION ( 'NONE',  ( -0.000000000000000000, -0.9350162426854121689, 0.3546048870425426158 ) ) ;
#25771=ORIENTED_EDGE ( 'NONE', *, *, #45474, .T. ) ;
#25774=LINE ( 'NONE', #1846, #34091 ) ;
#25777=ORIENTED_EDGE ( 'NONE', *, *, #18250, .F. ) ;
#25780=DIRECTION ( 'NONE',  ( 1.043714542225393381E-14, 0.5680647467311457088, -0.8229838658936634577 ) ) ;
#25782=ORIENTED_EDGE ( 'NONE', *, *, #31710, .T. ) ;
#25786=DIRECTION ( 'NONE',  ( 0.000000000000000000, -0.7485107481710934207, 0.6631226582408039638 ) ) ;
#25792=AXIS2_PLACEMENT_3D ( 'NONE', #28629, #1036, #45220 ) ;
#25794=CARTESIAN_POINT ( 'NONE',  ( -336.3521761649654422, -123.5000000000000284, 0.000000000000000000 ) ) ;
#25795=DIRECTION ( 'NONE',  ( 0.000000000000000000, 0.6631226582407989678, 0.7485107481710977506 ) ) ;
#25796=VECTOR ( 'NONE', #36604, 999.9999999999998863 ) ;
#25803=VECTOR ( 'NONE', #46454, 1000.000000000000000 ) ;
#25805=DIRECTION ( 'NONE',  ( 0.000000000000000000, 0.000000000000000000, 1.000000000000000000 ) ) ;
#25811=ORIENTED_EDGE ( 'NONE', *, *, #40118, .F. ) ;
#25814=DIRECTION ( 'NONE',  ( 0.000000000000000000, 1.323015771011644961E-13, 1.000000000000000000 ) ) ;
#25819=DIRECTION ( 'NONE',  ( 1.000000000000000000, 0.000000000000000000, -0.000000000000000000 ) ) ;
#25820=ORIENTED_EDGE ( 'NONE', *, *, #30302, .F. ) ;
#25821=VECTOR ( 'NONE', #29378, 1000.000000000000227 ) ;
#25835=DIRECTION ( 'NONE',  ( 0.000000000000000000, -0.6631226582407989678, -0.7485107481710977506 ) ) ;
#25843=DIRECTION ( 'NONE',  ( 0.000000000000000000, -0.8854560256532157947, -0.4647231720437573488 ) ) ;
#25846=CARTESIAN_POINT ( 'NONE',  ( -332.3517673607765914, -72.48138011061176655, -29.74944317415788930 ) ) ;
#25850=LINE ( 'NONE', #41877, #15549 ) ;
#25851=LINE ( 'NONE', #18229, #36137 ) ;
#25857=ORIENTED_EDGE ( 'NONE', *, *, #42697, .F. ) ;
#25863=LINE ( 'NONE', #13776, #20284 ) ;
#25871=ORIENTED_EDGE ( 'NONE', *, *, #23448, .F. ) ;
#25873=PLANE ( 'NONE',  #12416 ) ;
#25874=PLANE ( 'NONE',  #39492 ) ;
#25875=PLANE ( 'NONE',  #33304 ) ;
#25876=VERTEX_POINT ( 'NONE', #55 ) ;
#25877=ORIENTED_EDGE ( 'NONE', *, *, #7275, .T. ) ;
#25880=CARTESIAN_POINT ( 'NONE',  ( -330.4913330509368166, -89.57268800991514013, -48.27201571436026484 ) ) ;
#25886=EDGE_CURVE ( 'NONE', #4967, #3140, #11629, .T. ) ;
#25887=ORIENTED_EDGE ( 'NONE', *, *, #20635, .F. ) ;
#25892=AXIS2_PLACEMENT_3D ( 'NONE', #35580, #20594, #36629 ) ;
#25893=DIRECTION ( 'NONE',  ( 0.000000000000000000, 0.000000000000000000, -1.000000000000000000 ) ) ;
#25897=DIRECTION ( 'NONE',  ( -0.000000000000000000, 0.8229838658936556861, -0.5680647467311569221 ) ) ;
#25904=ORIENTED_EDGE ( 'NONE', *, *, #51631, .F. ) ;
#25908=LINE ( 'NONE', #41932, #25310 ) ;
#25910=EDGE_CURVE ( 'NONE', #23459, #34925, #11355, .T. ) ;
#25918=CARTESIAN_POINT ( 'NONE',  ( -332.3517673607765914, -180.3949349376675855, 15.70448169564087770 ) ) ;
#25919=ORIENTED_EDGE ( 'NONE', *, *, #43281, .T. ) ;
#25920=VERTEX_POINT ( 'NONE', #7441 ) ;
#25931=ORIENTED_EDGE ( 'NONE', *, *, #32725, .F. ) ;
#25936=CARTESIAN_POINT ( 'NONE',  ( -330.4913330509368166, -79.00630452878421295, 38.74998146212088557 ) ) ;
#25938=PLANE ( 'NONE',  #28465 ) ;
#25940=CARTESIAN_POINT ( 'NONE',  ( -339.1964088526558498, -124.0000000000002700, -59.00000000000002132 ) ) ;
#25944=EDGE_CURVE ( 'NONE', #4655, #16559, #20029, .T. ) ;
#25945=EDGE_CURVE ( 'NONE', #15564, #30781, #22691, .T. ) ;
#25949=PLANE ( 'NONE',  #29801 ) ;
#25958=DIRECTION ( 'NONE',  ( 1.000000000000000000, -0.000000000000000000, -0.000000000000000000 ) ) ;
#25963=EDGE_CURVE ( 'NONE', #20384, #51691, #13192, .T. ) ;
#25970=CARTESIAN_POINT ( 'NONE',  ( -339.1964088526558498, -172.3400804610915600, -33.10432812419107051 ) ) ;
#25971=VERTEX_POINT ( 'NONE', #40504 ) ;
#25974=EDGE_CURVE ( 'NONE', #186, #40642, #28937, .T. ) ;
#25975=DIRECTION ( 'NONE',  ( -1.000000000000000000, -0.000000000000000000, -0.000000000000000000 ) ) ;
#25976=CARTESIAN_POINT ( 'NONE',  ( -339.1964088526558498, -180.6659093959934523, -14.60509510167853264 ) ) ;
#25978=PLANE ( 'NONE',  #36393 ) ;
#25984=DIRECTION ( 'NONE',  ( 1.000000000000000000, -0.000000000000000000, -0.000000000000000000 ) ) ;
#25988=ORIENTED_EDGE ( 'NONE', *, *, #27237, .F. ) ;
#25992=DIRECTION ( 'NONE',  ( 1.000000000000000000, -0.000000000000000000, -0.000000000000000000 ) ) ;
#25995=CARTESIAN_POINT ( 'NONE',  ( -339.1964088526558498, -150.4759391377552618, 52.47426709956155122 ) ) ;
#25996=CARTESIAN_POINT ( 'NONE',  ( -339.1964088526558498, -71.49045607248255862, -27.86139516340906397 ) ) ;
#25997=ORIENTED_EDGE ( 'NONE', *, *, #43094, .T. ) ;
#25998=CARTESIAN_POINT ( 'NONE',  ( -339.1964088526558498, -84.00150778970699150, 43.83057281297409702 ) ) ;
#26003=ORIENTED_EDGE ( 'NONE', *, *, #8520, .F. ) ;
#26005=EDGE_CURVE ( 'NONE', #22651, #19986, #28673, .T. ) ;
#26011=ORIENTED_EDGE ( 'NONE', *, *, #40464, .T. ) ;
#26016=ORIENTED_EDGE ( 'NONE', *, *, #33719, .F. ) ;
#26018=ORIENTED_EDGE ( 'NONE', *, *, #21961, .T. ) ;
#26022=ORIENTED_EDGE ( 'NONE', *, *, #46913, .F. ) ;
#26025=AXIS2_PLACEMENT_3D ( 'NONE', #42398, #22694, #42911 ) ;
#26026=CARTESIAN_POINT ( 'NONE',  ( -339.1964088526558498, -70.60684477890951882, 28.32515014536776832 ) ) ;
#26035=LINE ( 'NONE', #42060, #44451 ) ;
#26036=PLANE ( 'NONE',  #39126 ) ;
#26038=VERTEX_POINT ( 'NONE', #29463 ) ;
#26040=CARTESIAN_POINT ( 'NONE',  ( -339.1964088526558498, -172.5932850007659169, -34.49419324804647147 ) ) ;
#26041=ADVANCED_FACE ( 'NONE', ( #8454 ), #45513, .F. ) ;
#26042=CARTESIAN_POINT ( 'NONE',  ( -305.0000000000000568, -107.5615171630107056, 57.84431488793861575 ) ) ;
#26044=VECTOR ( 'NONE', #43315, 1000.000000000000000 ) ;
#26054=CARTESIAN_POINT ( 'NONE',  ( -305.0000000000000568, -83.33976666099019326, -44.57752413667995484 ) ) ;
#26058=DIRECTION ( 'NONE',  ( -1.000000000000000000, -1.013386094502322405E-14, 2.497772389992582658E-15 ) ) ;
#26059=ORIENTED_EDGE ( 'NONE', *, *, #6675, .T. ) ;
#26067=VERTEX_POINT ( 'NONE', #1870 ) ;
#26068=DIRECTION ( 'NONE',  ( 1.000000000000000000, 0.000000000000000000, 0.000000000000000000 ) ) ;
#26071=VERTEX_POINT ( 'NONE', #22364 ) ;
#26072=AXIS2_PLACEMENT_3D ( 'NONE', #30076, #21683, #25112 ) ;
#26075=DIRECTION ( 'NONE',  ( 1.000000000000000000, 0.000000000000000000, 0.000000000000000000 ) ) ;
#26077=LINE ( 'NONE', #14006, #23260 ) ;
#26084=ORIENTED_EDGE ( 'NONE', *, *, #3814, .F. ) ;
#26088=ORIENTED_EDGE ( 'NONE', *, *, #37666, .F. ) ;
#26089=FACE_BOUND ( 'NONE', #38507, .T. ) ;
#26090=DIRECTION ( 'NONE',  ( 0.000000000000000000, 0.3546048870425300148, -0.9350162426854169428 ) ) ;
#26098=VERTEX_POINT ( 'NONE', #2400 ) ;
#26100=PLANE ( 'NONE',  #18847 ) ;
#26103=ORIENTED_EDGE ( 'NONE', *, *, #3406, .F. ) ;
#26104=LINE ( 'NONE', #6156, #30418 ) ;
#26107=DIRECTION ( 'NONE',  ( 0.000000000000000000, 0.000000000000000000, -1.000000000000000000 ) ) ;
#26112=CARTESIAN_POINT ( 'NONE',  ( -336.3521761649654422, -165.9166037625627439, 41.09453333279358134 ) ) ;
#26116=FACE_OUTER_BOUND ( 'NONE', #39018, .T. ) ;
#26126=CIRCLE ( 'NONE', #15218, 60.00000000000000000 ) ;
#26127=ORIENTED_EDGE ( 'NONE', *, *, #42303, .T. ) ;
#26132=DIRECTION ( 'NONE',  ( 0.000000000000000000, 0.000000000000000000, 1.000000000000000000 ) ) ;
#26139=CIRCLE ( 'NONE', #14424, 60.00000000000000000 ) ;
#26142=CARTESIAN_POINT ( 'NONE',  ( -336.3521761649654422, -69.20050475944881896, 25.52576769896172237 ) ) ;
#26143=PLANE ( 'NONE',  #33794 ) ;
#26144=DIRECTION ( 'NONE',  ( 1.000000000000000000, -0.000000000000000000, -0.000000000000000000 ) ) ;
#26147=ORIENTED_EDGE ( 'NONE', *, *, #47561, .T. ) ;
#26162=ORIENTED_EDGE ( 'NONE', *, *, #48090, .F. ) ;
#26164=ORIENTED_EDGE ( 'NONE', *, *, #1395, .T. ) ;
#26166=EDGE_CURVE ( 'NONE', #32359, #15270, #33923, .T. ) ;
#26168=VECTOR ( 'NONE', #8462, 1000.000000000000000 ) ;
#26169=DIRECTION ( 'NONE',  ( -0.000000000000000000, -0.4647231720437604574, 0.8854560256532141294 ) ) ;
#26173=CARTESIAN_POINT ( 'NONE',  ( 0.000000000000000000, -96.08133284941705199, 52.24190551353909484 ) ) ;
#26175=DIRECTION ( 'NONE',  ( -0.000000000000000000, -0.000000000000000000, -1.000000000000000000 ) ) ;
#26178=FACE_OUTER_BOUND ( 'NONE', #42232, .T. ) ;
#26181=EDGE_CURVE ( 'NONE', #27368, #36071, #26814, .T. ) ;
#26182=ORIENTED_EDGE ( 'NONE', *, *, #21305, .T. ) ;
#26187=CARTESIAN_POINT ( 'NONE',  ( -330.4913330509368166, -102.1108035431471279, 54.98865587491800255 ) ) ;
#26192=CIRCLE ( 'NONE', #48884, 60.00000000000000000 ) ;
#26194=ORIENTED_EDGE ( 'NONE', *, *, #1571, .F. ) ;
#26197=ORIENTED_EDGE ( 'NONE', *, *, #27386, .T. ) ;
#26199=ORIENTED_EDGE ( 'NONE', *, *, #2699, .F. ) ;
#26210=LINE ( 'NONE', #7032, #6924 ) ;
#26214=CARTESIAN_POINT ( 'NONE',  ( 0.000000000000000000, -144.4216883355091170, 55.16595831843969933 ) ) ;
#26221=DIRECTION ( 'NONE',  ( 0.000000000000000000, -0.9350162426854181641, -0.3546048870425267951 ) ) ;
#26226=AXIS2_PLACEMENT_3D ( 'NONE', #4634, #25140, #20938 ) ;
#26230=ORIENTED_EDGE ( 'NONE', *, *, #29141, .F. ) ;
#26231=EDGE_CURVE ( 'NONE', #17577, #5759, #47063, .T. ) ;
#26232=PLANE ( 'NONE',  #38001 ) ;
#26236=CARTESIAN_POINT ( 'NONE',  ( -339.1964088526558498, -68.15673923803898049, 20.45418021416614351 ) ) ;
#26238=DIRECTION ( 'NONE',  ( -1.000000000000000000, -0.000000000000000000, -0.000000000000000000 ) ) ;
#26240=DIRECTION ( 'NONE',  ( -1.000000000000000000, 0.000000000000000000, -0.000000000000000000 ) ) ;
#26246=DIRECTION ( 'NONE',  ( 0.000000000000000000, -0.9350162426854121689, 0.3546048870425426158 ) ) ;
#26251=EDGE_CURVE ( 'NONE', #22171, #36591, #5145, .T. ) ;
#26255=VECTOR ( 'NONE', #27010, 1000.000000000000000 ) ;
#26256=DIRECTION ( 'NONE',  ( -0.000000000000000000, 0.8854560256532141294, 0.4647231720437604574 ) ) ;
#26260=FACE_OUTER_BOUND ( 'NONE', #10506, .T. ) ;
#26261=ORIENTED_EDGE ( 'NONE', *, *, #19145, .F. ) ;
#26263=ORIENTED_EDGE ( 'NONE', *, *, #8678, .T. ) ;
#26267=DIRECTION ( 'NONE',  ( 0.000000000000000000, 0.000000000000000000, 1.000000000000000000 ) ) ;
#26270=ORIENTED_EDGE ( 'NONE', *, *, #46913, .T. ) ;
#26280=DIRECTION ( 'NONE',  ( -1.000000000000000000, 0.000000000000000000, 0.000000000000000000 ) ) ;
#26281=DIRECTION ( 'NONE',  ( 0.000000000000000000, 0.9350162426854132791, -0.3546048870425396182 ) ) ;
#26282=CARTESIAN_POINT ( 'NONE',  ( -339.1964088526558498, -74.65991953890826949, 33.10432812419072945 ) ) ;
#26283=CARTESIAN_POINT ( 'NONE',  ( -330.4913330509368166, -183.4979166304964622, 0.4999999999999549249 ) ) ;
#26287=LINE ( 'NONE', #38383, #7215 ) ;
#26291=AXIS2_PLACEMENT_3D ( 'NONE', #35797, #51855, #27660 ) ;
#26293=DIRECTION ( 'NONE',  ( -8.718379230999704661E-17, -0.5680647467311626952, -0.8229838658936516893 ) ) ;
#26296=EDGE_CURVE ( 'NONE', #37376, #5960, #15255, .T. ) ;
#26300=VECTOR ( 'NONE', #37232, 1000.000000000000000 ) ;
#26301=VERTEX_POINT ( 'NONE', #38899 ) ;
#26302=EDGE_CURVE ( 'NONE', #18571, #23872, #6852, .T. ) ;
#26309=VERTEX_POINT ( 'NONE', #31805 ) ;
#26310=EDGE_CURVE ( 'NONE', #51040, #27425, #12654, .T. ) ;
#26312=VECTOR ( 'NONE', #2657, 1000.000000000000000 ) ;
#26313=EDGE_CURVE ( 'NONE', #17026, #37409, #43875, .T. ) ;
#26316=ORIENTED_EDGE ( 'NONE', *, *, #49430, .T. ) ;
#26320=DIRECTION ( 'NONE',  ( -0.000000000000000000, -0.9927088740980544168, -0.1205366802553199251 ) ) ;
#26322=CARTESIAN_POINT ( 'NONE',  ( -332.3517673607765914, -70.03480886230919111, 25.08789112700620194 ) ) ;
#26324=VECTOR ( 'NONE', #30030, 1000.000000000000000 ) ;
#26326=EDGE_CURVE ( 'NONE', #6390, #29097, #4721, .T. ) ;
#26329=DIRECTION ( 'NONE',  ( -0.000000000000000000, -0.9350162426854158326, -0.3546048870425331234 ) ) ;
#26332=VECTOR ( 'NONE', #24659, 1000.000000000000227 ) ;
#26339=FACE_OUTER_BOUND ( 'NONE', #39187, .T. ) ;
#26342=ORIENTED_EDGE ( 'NONE', *, *, #45897, .F. ) ;
#26344=DIRECTION ( 'NONE',  ( 0.000000000000000000, -0.3546048870425235200, 0.9350162426854194964 ) ) ;
#26347=VECTOR ( 'NONE', #37286, 1000.000000000000000 ) ;
#26351=FACE_BOUND ( 'NONE', #15880, .T. ) ;
#26354=ORIENTED_EDGE ( 'NONE', *, *, #14279, .F. ) ;
#26355=DIRECTION ( 'NONE',  ( -0.000000000000000000, 1.000000000000000000, -0.000000000000000000 ) ) ;
#26357=CARTESIAN_POINT ( 'NONE',  ( -332.3517673607765914, -179.0013928959018301, 22.79463504017430253 ) ) ;
#26360=ADVANCED_FACE ( 'NONE', ( #9193 ), #36500, .T. ) ;
#26361=CARTESIAN_POINT ( 'NONE',  ( -305.0000000000000568, -114.6500883362968892, 59.34373651485599055 ) ) ;
#26362=CARTESIAN_POINT ( 'NONE',  ( -339.1964088526558498, -123.0000000000002700, -59.00000000000002132 ) ) ;
#26366=VERTEX_POINT ( 'NONE', #21269 ) ;
#26369=VERTEX_POINT ( 'NONE', #44413 ) ;
#26370=CARTESIAN_POINT ( 'NONE',  ( -339.1964088526558498, -123.5000000000000284, 0.000000000000000000 ) ) ;
#26372=DIRECTION ( 'NONE',  ( -1.000000000000000000, 0.000000000000000000, 0.000000000000000000 ) ) ;
#26373=EDGE_LOOP ( 'NONE', ( #30405, #50381, #49213, #3066 ) ) ;
#26374=ORIENTED_EDGE ( 'NONE', *, *, #36631, .T. ) ;
#26376=DIRECTION ( 'NONE',  ( 0.000000000000000000, -0.6631226582407911962, 0.7485107481711046340 ) ) ;
#26377=ORIENTED_EDGE ( 'NONE', *, *, #8283, .T. ) ;
#26379=ADVANCED_FACE ( 'NONE', ( #8656 ), #40976, .F. ) ;
#26382=CARTESIAN_POINT ( 'NONE',  ( -336.3521761649654422, -69.26746417191145611, -23.38292116578723068 ) ) ;
#26383=AXIS2_PLACEMENT_3D ( 'NONE', #46581, #50273, #22914 ) ;
#26385=PLANE ( 'NONE',  #49606 ) ;
#26397=VECTOR ( 'NONE', #50912, 1000.000000000000000 ) ;
#26400=ORIENTED_EDGE ( 'NONE', *, *, #33665, .F. ) ;
#26401=CARTESIAN_POINT ( 'NONE',  ( -332.3517673607765914, -182.3303666475049170, -11.78931550685388707 ) ) ;
#26406=CARTESIAN_POINT ( 'NONE',  ( -305.0000000000000568, -179.4217241332782464, 21.74306257088749206 ) ) ;
#26408=DIRECTION ( 'NONE',  ( 1.000000000000000000, 0.000000000000000000, -0.000000000000000000 ) ) ;
#26413=VECTOR ( 'NONE', #19510, 1000.000000000000000 ) ;
#26418=DIRECTION ( 'NONE',  ( -1.000000000000000000, 0.000000000000000000, 0.000000000000000000 ) ) ;
#26419=AXIS2_PLACEMENT_3D ( 'NONE', #34390, #2060, #18102 ) ;
#26424=ORIENTED_EDGE ( 'NONE', *, *, #9365, .T. ) ;
#26434=LINE ( 'NONE', #14363, #42222 ) ;
#26436=ORIENTED_EDGE ( 'NONE', *, *, #29434, .F. ) ;
#26439=CARTESIAN_POINT ( 'NONE',  ( -332.3517673607765914, -72.01665693856799066, -28.86398714850468039 ) ) ;
#26441=EDGE_LOOP ( 'NONE', ( #8346, #3912, #20074, #14711 ) ) ;
#26443=LINE ( 'NONE', #42478, #734 ) ;
#26445=VECTOR ( 'NONE', #27118, 1000.000000000000000 ) ;
#26446=CARTESIAN_POINT ( 'NONE',  ( -336.3521761649654422, -149.4733471526596134, 53.00046796564699036 ) ) ;
#26448=DIRECTION ( 'NONE',  ( -1.000000000000000000, 0.000000000000000000, 0.000000000000000000 ) ) ;
#26451=CIRCLE ( 'NONE', #35679, 60.00000000000000000 ) ;
#26455=CARTESIAN_POINT ( 'NONE',  ( -339.1964088526558498, -151.3613951634092700, -52.00954392751739164 ) ) ;
#26456=ORIENTED_EDGE ( 'NONE', *, *, #45897, .T. ) ;
#26461=CARTESIAN_POINT ( 'NONE',  ( -330.4913330509368166, -66.09477493971897388, 13.63415328425216622 ) ) ;
#26466=ORIENTED_EDGE ( 'NONE', *, *, #32224, .F. ) ;
#26469=ORIENTED_EDGE ( 'NONE', *, *, #29929, .T. ) ;
#26473=CARTESIAN_POINT ( 'NONE',  ( -332.3517673607765914, -123.5000000000000284, 0.000000000000000000 ) ) ;
#26485=EDGE_CURVE ( 'NONE', #35874, #39674, #49594, .T. ) ;
#26495=PLANE ( 'NONE',  #43037 ) ;
#26496=ORIENTED_EDGE ( 'NONE', *, *, #38224, .F. ) ;
#26497=DIRECTION ( 'NONE',  ( 0.000000000000000000, 0.000000000000000000, -1.000000000000000000 ) ) ;
#26498=PLANE ( 'NONE',  #35420 ) ;
#26502=AXIS2_PLACEMENT_3D ( 'NONE', #35859, #47952, #51917 ) ;
#26503=DIRECTION ( 'NONE',  ( -0.000000000000000000, 0.7485107481711069655, 0.6631226582407885317 ) ) ;
#26504=AXIS2_PLACEMENT_3D ( 'NONE', #32268, #17053, #40666 ) ;
#26507=PLANE ( 'NONE',  #33179 ) ;
#26508=ORIENTED_EDGE ( 'NONE', *, *, #23081, .F. ) ;
#26518=EDGE_LOOP ( 'NONE', ( #45134, #10238, #43079, #9311 ) ) ;
#26536=DIRECTION ( 'NONE',  ( 0.000000000000000000, 0.000000000000000000, 1.000000000000000000 ) ) ;
#26541=DIRECTION ( 'NONE',  ( 0.000000000000000000, -0.1205366802553233113, -0.9927088740980539727 ) ) ;
#26545=AXIS2_PLACEMENT_3D ( 'NONE', #36233, #4446, #40427 ) ;
#26550=LINE ( 'NONE', #6601, #13712 ) ;
#26571=VERTEX_POINT ( 'NONE', #18621 ) ;
#26574=AXIS2_PLACEMENT_3D ( 'NONE', #30486, #23130, #27315 ) ;
#26575=ORIENTED_EDGE ( 'NONE', *, *, #46958, .F. ) ;
#26576=DIRECTION ( 'NONE',  ( 0.000000000000000000, 0.000000000000000000, -1.000000000000000000 ) ) ;
#26582=ORIENTED_EDGE ( 'NONE', *, *, #7502, .T. ) ;
#26584=EDGE_CURVE ( 'NONE', #48562, #38308, #42005, .T. ) ;
#26585=CARTESIAN_POINT ( 'NONE',  ( -305.0000000000000568, -131.2283041299246520, -59.50019592636137844 ) ) ;
#26589=ORIENTED_EDGE ( 'NONE', *, *, #28824, .T. ) ;
#26592=CARTESIAN_POINT ( 'NONE',  ( -305.0000000000000568, -169.4764303083190384, -38.55084767037274673 ) ) ;
#26593=ORIENTED_EDGE ( 'NONE', *, *, #18951, .F. ) ;
#26594=EDGE_CURVE ( 'NONE', #14763, #30653, #46258, .T. ) ;
#26597=DIRECTION ( 'NONE',  ( -0.000000000000000000, 0.9709418174260492362, -0.2393156642875685636 ) ) ;
#26601=AXIS2_PLACEMENT_3D ( 'NONE', #1148, #4582, #48490 ) ;
#26602=VERTEX_POINT ( 'NONE', #35408 ) ;
#26607=ADVANCED_FACE ( 'NONE', ( #7053 ), #6797, .F. ) ;
#26609=AXIS2_PLACEMENT_3D ( 'NONE', #65, #47658, #44219 ) ;
#26612=FACE_BOUND ( 'NONE', #11308, .T. ) ;
#26614=DIRECTION ( 'NONE',  ( 0.000000000000000000, 0.000000000000000000, -1.000000000000000000 ) ) ;
#26615=EDGE_CURVE ( 'NONE', #15638, #1527, #26126, .T. ) ;
#26616=ORIENTED_EDGE ( 'NONE', *, *, #36879, .F. ) ;
#26619=VECTOR ( 'NONE', #26175, 1000.000000000000000 ) ;
#26622=AXIS2_PLACEMENT_3D ( 'NONE', #31829, #47866, #12087 ) ;
#26624=ORIENTED_EDGE ( 'NONE', *, *, #46503, .F. ) ;
#26631=EDGE_CURVE ( 'NONE', #12833, #46014, #23077, .T. ) ;
#26632=ORIENTED_EDGE ( 'NONE', *, *, #26631, .F. ) ;
#26636=CARTESIAN_POINT ( 'NONE',  ( -330.4913330509368166, -123.5000000000000284, 0.000000000000000000 ) ) ;
#26639=EDGE_LOOP ( 'NONE', ( #45372, #31720, #15474, #6315 ) ) ;
#26641=DIRECTION ( 'NONE',  ( -1.000000000000000000, -0.000000000000000000, -0.000000000000000000 ) ) ;
#26644=VECTOR ( 'NONE', #8961, 1000.000000000000000 ) ;
#26648=ORIENTED_EDGE ( 'NONE', *, *, #264, .T. ) ;
#26649=CARTESIAN_POINT ( 'NONE',  ( -305.0000000000000568, -149.0257676989619142, 54.29949524055110999 ) ) ;
#26653=CARTESIAN_POINT ( 'NONE',  ( -339.1964088526558498, -71.02573290043838483, 26.97593913775504504 ) ) ;
#26654=ORIENTED_EDGE ( 'NONE', *, *, #41683, .F. ) ;
#26655=ORIENTED_EDGE ( 'NONE', *, *, #30676, .T. ) ;
#26659=VECTOR ( 'NONE', #7519, 1000.000000000000000 ) ;
#26674=ORIENTED_EDGE ( 'NONE', *, *, #11042, .F. ) ;
#26675=CARTESIAN_POINT ( 'NONE',  ( 0.000000000000000000, -130.6116641350643022, -58.56982357178517873 ) ) ;
#26684=VECTOR ( 'NONE', #16206, 1000.000000000000000 ) ;
#26686=CARTESIAN_POINT ( 'NONE',  ( -336.3521761649654422, -123.5000000000000284, 0.000000000000000000 ) ) ;
#26688=VECTOR ( 'NONE', #42678, 1000.000000000000114 ) ;
#26690=DIRECTION ( 'NONE',  ( 0.000000000000000000, 0.8229838658936634577, 0.5680647467311457088 ) ) ;
#26692=FACE_OUTER_BOUND ( 'NONE', #34526, .T. ) ;
#26695=ORIENTED_EDGE ( 'NONE', *, *, #22467, .T. ) ;
#26698=ORIENTED_EDGE ( 'NONE', *, *, #29929, .F. ) ;
#26705=DIRECTION ( 'NONE',  ( -1.000000000000000000, 0.000000000000000000, 0.000000000000000000 ) ) ;
#26706=CARTESIAN_POINT ( 'NONE',  ( -332.3517673607765914, -113.7752393642576720, 58.25253621232167944 ) ) ;
#26709=DIRECTION ( 'NONE',  ( 0.000000000000000000, 0.000000000000000000, 1.000000000000000000 ) ) ;
#26712=ORIENTED_EDGE ( 'NONE', *, *, #49729, .T. ) ;
#26714=LINE ( 'NONE', #50903, #33458 ) ;
#26717=CARTESIAN_POINT ( 'NONE',  ( -336.3521761649654422, -118.0087234915157381, -58.76657425099333665 ) ) ;
#26719=VERTEX_POINT ( 'NONE', #16492 ) ;
#26720=VECTOR ( 'NONE', #18959, 1000.000000000000114 ) ;
#26722=CARTESIAN_POINT ( 'NONE',  ( -332.3517673607765914, -87.81784868886214213, 47.06073758877343494 ) ) ;
#26729=CARTESIAN_POINT ( 'NONE',  ( -336.3521761649654422, -165.9166037625627439, 41.09453333279358134 ) ) ;
#26731=DIRECTION ( 'NONE',  ( 0.000000000000000000, 0.000000000000000000, 1.000000000000000000 ) ) ;
#26732=VERTEX_POINT ( 'NONE', #438 ) ;
#26733=PLANE ( 'NONE',  #27534 ) ;
#26741=DIRECTION ( 'NONE',  ( 1.000000000000000000, -0.000000000000000000, -0.000000000000000000 ) ) ;
#26743=DIRECTION ( 'NONE',  ( -0.000000000000000000, 0.8854560256532093554, -0.4647231720437695057 ) ) ;
#26745=PLANE ( 'NONE',  #50676 ) ;
#26753=ORIENTED_EDGE ( 'NONE', *, *, #8922, .T. ) ;
#26764=DIRECTION ( 'NONE',  ( -1.000000000000000000, -3.701062773504815647E-15, 9.758900497077172511E-15 ) ) ;
#26765=FACE_OUTER_BOUND ( 'NONE', #51519, .T. ) ;
#26767=PLANE ( 'NONE',  #10704 ) ;
#26771=DIRECTION ( 'NONE',  ( -1.000000000000000000, 0.000000000000000000, -0.000000000000000000 ) ) ;
#26772=ADVANCED_FACE ( 'NONE', ( #49065 ), #28811, .T. ) ;
#26776=CARTESIAN_POINT ( 'NONE',  ( -340.0000000000000568, -123.5000000000000284, 0.000000000000000000 ) ) ;
#26779=ORIENTED_EDGE ( 'NONE', *, *, #40971, .T. ) ;
#26790=DIRECTION ( 'NONE',  ( -1.000000000000000000, 0.000000000000000000, 0.000000000000000000 ) ) ;
#26791=FACE_OUTER_BOUND ( 'NONE', #2002, .T. ) ;
#26796=PLANE ( 'NONE',  #47182 ) ;
#26801=DIRECTION ( 'NONE',  ( 1.000000000000000000, -0.000000000000000000, 0.000000000000000000 ) ) ;
#26803=PLANE ( 'NONE',  #20095 ) ;
#26805=VERTEX_POINT ( 'NONE', #15974 ) ;
#26807=CARTESIAN_POINT ( 'NONE',  ( -336.3521761649654422, -113.7752393642576720, 58.25253621232167944 ) ) ;
#26808=CIRCLE ( 'NONE', #22625, 60.00000000000000000 ) ;
#26813=DIRECTION ( 'NONE',  ( 1.000000000000000000, -0.000000000000000000, -0.000000000000000000 ) ) ;
#26814=LINE ( 'NONE', #50241, #36108 ) ;
#26815=DIRECTION ( 'NONE',  ( -0.000000000000000000, 1.000000000000000000, -0.000000000000000000 ) ) ;
#26816=ORIENTED_EDGE ( 'NONE', *, *, #27479, .F. ) ;
#26817=CARTESIAN_POINT ( 'NONE',  ( -339.1964088526558498, -150.4759391377552618, 52.47426709956155122 ) ) ;
#26823=ORIENTED_EDGE ( 'NONE', *, *, #28506, .T. ) ;
#26824=ADVANCED_FACE ( 'NONE', ( #181 ), #36972, .T. ) ;
#26825=ADVANCED_FACE ( 'NONE', ( #32513 ), #12007, .F. ) ;
#26832=EDGE_CURVE ( 'NONE', #48811, #15941, #11863, .T. ) ;
#26841=CARTESIAN_POINT ( 'NONE',  ( -332.3517673607765914, -64.61288906875131488, 4.498567634385603142 ) ) ;
#26843=ORIENTED_EDGE ( 'NONE', *, *, #7686, .F. ) ;
#26844=ADVANCED_FACE ( 'NONE', ( #40373 ), #4393, .F. ) ;
#26845=CARTESIAN_POINT ( 'NONE',  ( -305.0000000000000568, -81.78065195202965754, 43.12187378178632002 ) ) ;
#26851=PLANE ( 'NONE',  #25736 ) ;
#26858=CARTESIAN_POINT ( 'NONE',  ( -336.3521761649654422, -100.1170788342122080, 54.23253582808833073 ) ) ;
#26859=CARTESIAN_POINT ( 'NONE',  ( -339.1964088526558498, -138.3439121830091665, 58.13482838284733845 ) ) ;
#26860=VERTEX_POINT ( 'NONE', #20684 ) ;
#26861=FACE_BOUND ( 'NONE', #32167, .T. ) ;
#26862=FACE_OUTER_BOUND ( 'NONE', #35906, .T. ) ;
#26865=EDGE_LOOP ( 'NONE', ( #20519, #26654, #11026, #39760 ) ) ;
#26866=PLANE ( 'NONE',  #13058 ) ;
#26870=LINE ( 'NONE', #27128, #2907 ) ;
#26871=CARTESIAN_POINT ( 'NONE',  ( -336.3521761649654422, -133.2247606357419443, -58.25253621232173629 ) ) ;
#26875=FACE_OUTER_BOUND ( 'NONE', #49798, .T. ) ;
#26877=DIRECTION ( 'NONE',  ( -1.000000000000000000, 0.000000000000000000, -0.000000000000000000 ) ) ;
#26889=AXIS2_PLACEMENT_3D ( 'NONE', #16506, #40146, #36194 ) ;
#26890=CARTESIAN_POINT ( 'NONE',  ( -339.1964088526558498, -167.3305728129742249, 39.49849221029288060 ) ) ;
#26895=EDGE_CURVE ( 'NONE', #11938, #17341, #38459, .T. ) ;
#26897=DIRECTION ( 'NONE',  ( 0.000000000000000000, -0.5680647467311656929, -0.8229838658936495799 ) ) ;
#26903=ADVANCED_FACE ( 'NONE', ( #22443, #14822 ), #50309, .F. ) ;
#26915=AXIS2_PLACEMENT_3D ( 'NONE', #49401, #44138, #24181 ) ;
#26921=PLANE ( 'NONE',  #24895 ) ;
#26923=CARTESIAN_POINT ( 'NONE',  ( -336.3521761649654422, -172.9832938399466684, -32.17247266903247294 ) ) ;
#26924=ORIENTED_EDGE ( 'NONE', *, *, #3173, .F. ) ;
#26934=DIRECTION ( 'NONE',  ( 1.000000000000000000, -0.000000000000000000, -0.000000000000000000 ) ) ;
#26936=DIRECTION ( 'NONE',  ( 1.000000000000000000, -7.175085443855040167E-17, 4.952603889764104279E-17 ) ) ;
#26937=EDGE_CURVE ( 'NONE', #22804, #3919, #9339, .T. ) ;
#26939=CARTESIAN_POINT ( 'NONE',  ( -330.4913330509368166, -130.1153096980145563, 58.63009191191294178 ) ) ;
#26940=CARTESIAN_POINT ( 'NONE',  ( -336.3521761649654422, -179.5993808087905279, -18.46045550523168899 ) ) ;
#26941=ORIENTED_EDGE ( 'NONE', *, *, #17013, .T. ) ;
#26943=EDGE_CURVE ( 'NONE', #47521, #18519, #46299, .T. ) ;
#26945=EDGE_CURVE ( 'NONE', #21474, #20782, #30329, .T. ) ;
#26949=EDGE_CURVE ( 'NONE', #19447, #30532, #50557, .T. ) ;
#26959=CARTESIAN_POINT ( 'NONE',  ( -330.4913330509368166, -95.17484985463171654, -52.89315522109019696 ) ) ;
#26962=VERTEX_POINT ( 'NONE', #17271 ) ;
#26964=FACE_OUTER_BOUND ( 'NONE', #11544, .T. ) ;
#26966=AXIS2_PLACEMENT_3D ( 'NONE', #43959, #48699, #7708 ) ;
#26969=CARTESIAN_POINT ( 'NONE',  ( 0.000000000000000000, -84.37576316379256980, 44.16213414209452992 ) ) ;
#26970=FACE_OUTER_BOUND ( 'NONE', #14429, .T. ) ;
#26971=ORIENTED_EDGE ( 'NONE', *, *, #1293, .T. ) ;
#26972=EDGE_CURVE ( 'NONE', #38711, #50590, #21970, .T. ) ;
#26977=CARTESIAN_POINT ( 'NONE',  ( -330.4913330509368166, -178.8432607619609200, -20.45418021416661247 ) ) ;
#26979=ORIENTED_EDGE ( 'NONE', *, *, #43271, .T. ) ;
#26985=ORIENTED_EDGE ( 'NONE', *, *, #2059, .T. ) ;
#26986=FACE_OUTER_BOUND ( 'NONE', #46646, .T. ) ;
#26987=ORIENTED_EDGE ( 'NONE', *, *, #46521, .T. ) ;
#26991=DIRECTION ( 'NONE',  ( -0.000000000000000000, -0.9350162426854169428, -0.3546048870425300148 ) ) ;
#27000=FACE_OUTER_BOUND ( 'NONE', #50496, .T. ) ;
#27001=DIRECTION ( 'NONE',  ( -0.000000000000000000, 0.9709418174260519008, -0.2393156642875582940 ) ) ;
#27003=CARTESIAN_POINT ( 'NONE',  ( -332.3517673607765914, -71.64707600775140861, -30.18731974611341684 ) ) ;
#27008=ORIENTED_EDGE ( 'NONE', *, *, #41732, .F. ) ;
#27009=EDGE_CURVE ( 'NONE', #16316, #7787, #7713, .T. ) ;
#27010=DIRECTION ( 'NONE',  ( 1.000000000000000000, -0.000000000000000000, -0.000000000000000000 ) ) ;
#27018=VERTEX_POINT ( 'NONE', #24245 ) ;
#27021=CARTESIAN_POINT ( 'NONE',  ( -332.3517673607765914, -167.3116148657362032, 40.99441916720375900 ) ) ;
#27024=DIRECTION ( 'NONE',  ( 1.000000000000000000, -0.000000000000000000, -0.000000000000000000 ) ) ;
#27025=VECTOR ( 'NONE', #25741, 1000.000000000000000 ) ;
#27026=ADVANCED_FACE ( 'NONE', ( #43945 ), #11360, .T. ) ;
#27028=CARTESIAN_POINT ( 'NONE',  ( -330.4913330509368166, -172.5932850007659169, -34.49419324804648568 ) ) ;
#27029=ORIENTED_EDGE ( 'NONE', *, *, #12136, .F. ) ;
#27033=AXIS2_PLACEMENT_3D ( 'NONE', #22564, #14666, #38314 ) ;
#27037=DIRECTION ( 'NONE',  ( 0.000000000000000000, 0.000000000000000000, 1.000000000000000000 ) ) ;
#27042=CARTESIAN_POINT ( 'NONE',  ( -339.1964088526558498, -103.0458197858324496, 55.34326076196052213 ) ) ;
#27045=VERTEX_POINT ( 'NONE', #51857 ) ;
#27048=VERTEX_POINT ( 'NONE', #47653 ) ;
#27049=PLANE ( 'NONE',  #33922 ) ;
#27053=CARTESIAN_POINT ( 'NONE',  ( -336.3521761649654422, -119.0014323656137947, -58.88711093124865670 ) ) ;
#27054=ORIENTED_EDGE ( 'NONE', *, *, #4126, .T. ) ;
#27057=DIRECTION ( 'NONE',  ( 1.000000000000000000, 0.000000000000000000, 0.000000000000000000 ) ) ;
#27060=ORIENTED_EDGE ( 'NONE', *, *, #18619, .T. ) ;
#27068=VECTOR ( 'NONE', #31474, 999.9999999999998863 ) ;
#27074=FACE_OUTER_BOUND ( 'NONE', #20523, .T. ) ;
#27077=EDGE_LOOP ( 'NONE', ( #32824, #12636, #48716, #3551 ) ) ;
#27090=CARTESIAN_POINT ( 'NONE',  ( -305.0000000000000568, -84.94915232962709695, -45.97643030831888211 ) ) ;
#27094=ORIENTED_EDGE ( 'NONE', *, *, #48696, .T. ) ;
#27097=LINE ( 'NONE', #43134, #46579 ) ;
#27098=ORIENTED_EDGE ( 'NONE', *, *, #44869, .F. ) ;
#27100=PLANE ( 'NONE',  #27972 ) ;
#27102=LINE ( 'NONE', #22205, #33219 ) ;
#27104=VECTOR ( 'NONE', #3310, 1000.000000000000000 ) ;
#27107=EDGE_LOOP ( 'NONE', ( #28786, #16185, #43994, #42667 ) ) ;
#27108=AXIS2_PLACEMENT_3D ( 'NONE', #28592, #5487, #4968 ) ;
#27118=DIRECTION ( 'NONE',  ( -1.000000000000000000, 0.000000000000000000, -0.000000000000000000 ) ) ;
#27120=VERTEX_POINT ( 'NONE', #60 ) ;
#27123=DIRECTION ( 'NONE',  ( -1.000000000000000000, 0.000000000000000000, -0.000000000000000000 ) ) ;
#27125=EDGE_LOOP ( 'NONE', ( #42491, #37292, #17236, #33580 ) ) ;
#27126=AXIS2_PLACEMENT_3D ( 'NONE', #19567, #51628, #20087 ) ;
#27128=CARTESIAN_POINT ( 'NONE',  ( -305.0000000000000568, -172.5932850007659169, -34.49419324804647857 ) ) ;
#27133=LINE ( 'NONE', #43168, #21241 ) ;
#27137=CARTESIAN_POINT ( 'NONE',  ( -336.3521761649654422, -101.0520950768976149, 54.58714071513087873 ) ) ;
#27139=ORIENTED_EDGE ( 'NONE', *, *, #33069, .T. ) ;
#27140=LINE ( 'NONE', #38713, #34151 ) ;
#27141=CONICAL_SURFACE ( 'NONE', #43096, 10.00000000000000711, 0.03490658503988659789 ) ;
#27147=ORIENTED_EDGE ( 'NONE', *, *, #24585, .T. ) ;
#27149=CARTESIAN_POINT ( 'NONE',  ( -339.1964088526558498, -144.8891964568517778, 54.98865587491845730 ) ) ;
#27151=FACE_OUTER_BOUND ( 'NONE', #23983, .T. ) ;
#27154=EDGE_LOOP ( 'NONE', ( #5352, #35467, #14, #3095 ) ) ;
#27156=DIRECTION ( 'NONE',  ( -0.000000000000000000, -3.491481338843133355E-15, -1.000000000000000000 ) ) ;
#27160=FACE_OUTER_BOUND ( 'NONE', #9058, .T. ) ;
#27161=VECTOR ( 'NONE', #24115, 1000.000000000000000 ) ;
#27162=EDGE_LOOP ( 'NONE', ( #46280, #17953, #1801, #29233 ) ) ;
#27168=DIRECTION ( 'NONE',  ( -0.000000000000000000, 0.000000000000000000, -1.000000000000000000 ) ) ;
#27171=ORIENTED_EDGE ( 'NONE', *, *, #27175, .T. ) ;
#27172=DIRECTION ( 'NONE',  ( -0.000000000000000000, 0.000000000000000000, 1.000000000000000000 ) ) ;
#27175=EDGE_CURVE ( 'NONE', #36591, #33846, #8720, .T. ) ;
#27178=CARTESIAN_POINT ( 'NONE',  ( -330.4913330509368166, -162.9984922102926532, -43.83057281297441676 ) ) ;
#27183=ORIENTED_EDGE ( 'NONE', *, *, #22807, .T. ) ;
#27185=CARTESIAN_POINT ( 'NONE',  ( -336.3521761649654422, -111.9361751271348879, -57.91551518289410438 ) ) ;
#27188=DIRECTION ( 'NONE',  ( 1.000000000000000000, -0.000000000000000000, -0.000000000000000000 ) ) ;
#27189=EDGE_CURVE ( 'NONE', #8253, #18753, #9509, .T. ) ;
#27191=ORIENTED_EDGE ( 'NONE', *, *, #46257, .T. ) ;
#27195=ORIENTED_EDGE ( 'NONE', *, *, #15951, .T. ) ;
#27198=AXIS2_PLACEMENT_3D ( 'NONE', #1271, #17326, #24940 ) ;
#27206=DIRECTION ( 'NONE',  ( 0.000000000000000000, 0.000000000000000000, -1.000000000000000000 ) ) ;
#27217=FACE_OUTER_BOUND ( 'NONE', #536, .T. ) ;
#27220=DIRECTION ( 'NONE',  ( -0.000000000000000000, -0.9709418174260534551, -0.2393156642875516327 ) ) ;
#27221=ORIENTED_EDGE ( 'NONE', *, *, #49729, .F. ) ;
#27227=DIRECTION ( 'NONE',  ( -1.000000000000000000, -0.000000000000000000, 0.000000000000000000 ) ) ;
#27230=DIRECTION ( 'NONE',  ( -0.000000000000000000, -0.6631226582407989678, -0.7485107481710977506 ) ) ;
#27232=VECTOR ( 'NONE', #1274, 1000.000000000000000 ) ;
#27234=EDGE_CURVE ( 'NONE', #36520, #42349, #13197, .T. ) ;
#27235=DIRECTION ( 'NONE',  ( -1.000000000000000000, -0.000000000000000000, -0.000000000000000000 ) ) ;
#27237=EDGE_CURVE ( 'NONE', #38924, #8616, #45274, .T. ) ;
#27239=ORIENTED_EDGE ( 'NONE', *, *, #13435, .T. ) ;
#27240=FACE_OUTER_BOUND ( 'NONE', #31613, .T. ) ;
#27241=VERTEX_POINT ( 'NONE', #21608 ) ;
#27247=EDGE_CURVE ( 'NONE', #22244, #29772, #17417, .T. ) ;
#27250=FACE_OUTER_BOUND ( 'NONE', #32446, .T. ) ;
#27252=CARTESIAN_POINT ( 'NONE',  ( -330.0000000000000568, -123.5000000000000284, 31.65769145387501027 ) ) ;
#27258=ADVANCED_FACE ( 'NONE', ( #24756 ), #45519, .F. ) ;
#27260=ORIENTED_EDGE ( 'NONE', *, *, #10646, .F. ) ;
#27262=CARTESIAN_POINT ( 'NONE',  ( -336.3521761649654422, -182.3871109312487420, -4.498567634386014369 ) ) ;
#27269=LINE ( 'NONE', #19147, #29305 ) ;
#27277=ORIENTED_EDGE ( 'NONE', *, *, #11114, .F. ) ;
#27280=ORIENTED_EDGE ( 'NONE', *, *, #44218, .T. ) ;
#27288=CARTESIAN_POINT ( 'NONE',  ( -305.0000000000000568, -123.5000000000000284, -20.00000000000000355 ) ) ;
#27291=CARTESIAN_POINT ( 'NONE',  ( -305.0000000000000568, -85.72124494520284088, -46.61293454085073051 ) ) ;
#27300=DIRECTION ( 'NONE',  ( 0.000000000000000000, -0.9927088740980530845, 0.1205366802553303057 ) ) ;
#27303=CARTESIAN_POINT ( 'NONE',  ( -336.3521761649654422, -114.7679482383557144, 58.37307289257701370 ) ) ;
#27306=ADVANCED_FACE ( 'NONE', ( #37880 ), #10284, .F. ) ;
#27307=CARTESIAN_POINT ( 'NONE',  ( -330.4913330509368166, -168.0775241366795569, 40.16023333901030412 ) ) ;
#27311=CARTESIAN_POINT ( 'NONE',  ( 0.000000000000000000, -178.6659583184393796, 20.92168833551003004 ) ) ;
#27313=CARTESIAN_POINT ( 'NONE',  ( -305.0000000000000568, -181.3443148879387081, 15.93848283698911317 ) ) ;
#27315=DIRECTION ( 'NONE',  ( 0.000000000000000000, 0.3546048870425363986, 0.9350162426854146114 ) ) ;
#27321=CARTESIAN_POINT ( 'NONE',  ( -336.3521761649654422, -182.3303666475049170, -11.78931550685388707 ) ) ;
#27326=VECTOR ( 'NONE', #20517, 1000.000000000000000 ) ;
#27329=CARTESIAN_POINT ( 'NONE',  ( -339.1964088526558498, -96.06030588028407635, 53.35787839313353942 ) ) ;
#27332=VECTOR ( 'NONE', #24653, 1000.000000000000114 ) ;
#27333=VERTEX_POINT ( 'NONE', #42333 ) ;
#27336=CARTESIAN_POINT ( 'NONE',  ( -332.3517673607765914, -179.2447759217480154, -19.39547174791710660 ) ) ;
#27337=FACE_OUTER_BOUND ( 'NONE', #6650, .T. ) ;
#27338=DIRECTION ( 'NONE',  ( 0.000000000000000000, 0.000000000000000000, -1.000000000000000000 ) ) ;
#27344=ORIENTED_EDGE ( 'NONE', *, *, #6085, .T. ) ;
#27345=AXIS2_PLACEMENT_3D ( 'NONE', #42785, #41998, #30187 ) ;
#27347=LINE ( 'NONE', #31548, #28395 ) ;
#27348=VECTOR ( 'NONE', #23625, 1000.000000000000000 ) ;
#27350=CARTESIAN_POINT ( 'NONE',  ( -339.1964088526558498, -103.0458197858333165, -55.34326076196084188 ) ) ;
#27351=ORIENTED_EDGE ( 'NONE', *, *, #37166, .T. ) ;
#27353=PLANE ( 'NONE',  #5931 ) ;
#27356=ORIENTED_EDGE ( 'NONE', *, *, #19564, .F. ) ;
#27359=CARTESIAN_POINT ( 'NONE',  ( -336.3521761649654422, -142.2945752170892035, 56.98038208374156710 ) ) ;
#27360=EDGE_LOOP ( 'NONE', ( #9455, #26162, #51730, #26342 ) ) ;
#27361=DIRECTION ( 'NONE',  ( 0.000000000000000000, 0.000000000000000000, 1.000000000000000000 ) ) ;
#27363=EDGE_CURVE ( 'NONE', #7018, #232, #42851, .T. ) ;
#27364=LINE ( 'NONE', #10831, #582 ) ;
#27365=DIRECTION ( 'NONE',  ( 0.000000000000000000, -0.9927088740980526405, 0.1205366802553337890 ) ) ;
#27368=VERTEX_POINT ( 'NONE', #2911 ) ;
#27371=VERTEX_POINT ( 'NONE', #22370 ) ;
#27373=EDGE_LOOP ( 'NONE', ( #1097, #26194, #32396, #217 ) ) ;
#27375=DIRECTION ( 'NONE',  ( 0.000000000000000000, 0.000000000000000000, -1.000000000000000000 ) ) ;
#27378=LINE ( 'NONE', #14801, #26445 ) ;
#27381=ORIENTED_EDGE ( 'NONE', *, *, #50907, .T. ) ;
#27382=VECTOR ( 'NONE', #7559, 999.9999999999998863 ) ;
#27386=EDGE_CURVE ( 'NONE', #5683, #36042, #34966, .T. ) ;
#27388=CARTESIAN_POINT ( 'NONE',  ( -336.3521761649654422, -181.4155151828941825, -11.56382487286496463 ) ) ;
#27393=VECTOR ( 'NONE', #17734, 1000.000000000000000 ) ;
#27394=DIRECTION ( 'NONE',  ( 1.000000000000000000, -0.000000000000000000, -0.000000000000000000 ) ) ;
#27395=CARTESIAN_POINT ( 'NONE',  ( -339.1964088526558498, -162.9984922102920848, 43.83057281297495678 ) ) ;
#27402=AXIS2_PLACEMENT_3D ( 'NONE', #25113, #25610, #45091 ) ;
#27407=EDGE_CURVE ( 'NONE', #32388, #19412, #18437, .T. ) ;
#27412=CARTESIAN_POINT ( 'NONE',  ( -330.4913330509368166, -108.8949048983213004, -57.16590939599337418 ) ) ;
#27415=ORIENTED_EDGE ( 'NONE', *, *, #43568, .T. ) ;
#27416=ORIENTED_EDGE ( 'NONE', *, *, #4950, .F. ) ;
#27423=CARTESIAN_POINT ( 'NONE',  ( -330.4913330509368166, -131.1080185721132807, -58.50955523165751515 ) ) ;
#27425=VERTEX_POINT ( 'NONE', #3677 ) ;
#27431=EDGE_CURVE ( 'NONE', #27425, #3020, #39667, .T. ) ;
#27433=ORIENTED_EDGE ( 'NONE', *, *, #41321, .F. ) ;
#27434=VECTOR ( 'NONE', #48771, 1000.000000000000000 ) ;
#27444=CARTESIAN_POINT ( 'NONE',  ( -330.4913330509368166, -108.6560878169904640, -58.13482838284724608 ) ) ;
#27445=ORIENTED_EDGE ( 'NONE', *, *, #6916, .F. ) ;
#27453=ORIENTED_EDGE ( 'NONE', *, *, #22489, .T. ) ;
#27457=LINE ( 'NONE', #23779, #30766 ) ;
#27458=EDGE_CURVE ( 'NONE', #43120, #32812, #51523, .T. ) ;
#27461=ORIENTED_EDGE ( 'NONE', *, *, #15630, .T. ) ;
#27465=CARTESIAN_POINT ( 'NONE',  ( -330.4913330509368166, -79.66942718702547666, -39.49849221029252533 ) ) ;
#27467=VECTOR ( 'NONE', #24699, 1000.000000000000000 ) ;
#27470=CARTESIAN_POINT ( 'NONE',  ( -336.3521761649653854, -66.84097189748108292, 19.74220186498881091 ) ) ;
#27475=FACE_OUTER_BOUND ( 'NONE', #11799, .T. ) ;
#27479=EDGE_CURVE ( 'NONE', #41341, #7980, #26192, .T. ) ;
#27481=VECTOR ( 'NONE', #17895, 1000.000000000000000 ) ;
#27482=FACE_OUTER_BOUND ( 'NONE', #43235, .T. ) ;
#27486=ORIENTED_EDGE ( 'NONE', *, *, #13077, .T. ) ;
#27490=CARTESIAN_POINT ( 'NONE',  ( -332.3517673607765914, -164.4944191672036311, -43.81161486573635244 ) ) ;
#27497=ORIENTED_EDGE ( 'NONE', *, *, #45971, .F. ) ;
#27498=CARTESIAN_POINT ( 'NONE',  ( -332.3517673607765914, -170.5607375887735770, 35.68215131113770155 ) ) ;
#27505=FACE_OUTER_BOUND ( 'NONE', #11983, .T. ) ;
#27513=VERTEX_POINT ( 'NONE', #15263 ) ;
#27515=AXIS2_PLACEMENT_3D ( 'NONE', #29020, #1439, #41375 ) ;
#27522=LINE ( 'NONE', #40365, #27161 ) ;
#27523=PLANE ( 'NONE',  #18996 ) ;
#27525=LINE ( 'NONE', #14949, #37460 ) ;
#27530=PLANE ( 'NONE',  #18696 ) ;
#27531=ORIENTED_EDGE ( 'NONE', *, *, #48642, .F. ) ;
#27534=AXIS2_PLACEMENT_3D ( 'NONE', #22796, #38809, #51442 ) ;
#27539=ORIENTED_EDGE ( 'NONE', *, *, #32224, .T. ) ;
#27542=ADVANCED_FACE ( 'NONE', ( #27074 ), #36011, .F. ) ;
#27545=EDGE_LOOP ( 'NONE', ( #39238, #376, #8516, #49614 ) ) ;
#27546=ADVANCED_FACE ( 'NONE', ( #49142 ), #20485, .T. ) ;
#27556=CARTESIAN_POINT ( 'NONE',  ( -336.3521761649654422, -72.01665693856799066, -28.86398714850468039 ) ) ;
#27559=LINE ( 'NONE', #43590, #42648 ) ;
#27561=EDGE_CURVE ( 'NONE', #1527, #51496, #17354, .T. ) ;
#27569=PLANE ( 'NONE',  #30789 ) ;
#27579=LINE ( 'NONE', #43608, #18805 ) ;
#27580=CARTESIAN_POINT ( 'NONE',  ( -339.1964088526558498, -157.4273119900845757, 48.27201571436049932 ) ) ;
#27588=CARTESIAN_POINT ( 'NONE',  ( -332.3517673607765914, -123.5000000000000284, 0.000000000000000000 ) ) ;
#27592=CARTESIAN_POINT ( 'NONE',  ( 0.000000000000000000, -109.3803758070342838, -57.28556722813713975 ) ) ;
#27595=CARTESIAN_POINT ( 'NONE',  ( 0.000000000000000000, -96.08133284941705199, 52.24190551353909484 ) ) ;
#27607=EDGE_CURVE ( 'NONE', #19447, #45420, #29153, .T. ) ;
#27610=EDGE_CURVE ( 'NONE', #47197, #51691, #5259, .T. ) ;
#27613=VECTOR ( 'NONE', #22580, 1000.000000000000000 ) ;
#27617=CARTESIAN_POINT ( 'NONE',  ( -336.3521761649654422, -181.4155151828941825, -11.56382487286496463 ) ) ;
#27619=CARTESIAN_POINT ( 'NONE',  ( -339.1964088526558498, -182.1300919119129560, -6.615309698014600670 ) ) ;
#27620=CARTESIAN_POINT ( 'NONE',  ( -336.3521761649654422, -106.8245764869328980, 56.65561927337994064 ) ) ;
#27621=VECTOR ( 'NONE', #8768, 1000.000000000000000 ) ;
#27623=DIRECTION ( 'NONE',  ( 1.000000000000000000, 7.175085443855077145E-17, -4.952603889764050661E-17 ) ) ;
#27624=VERTEX_POINT ( 'NONE', #32834 ) ;
#27626=FACE_OUTER_BOUND ( 'NONE', #16014, .T. ) ;
#27628=LINE ( 'NONE', #43658, #50746 ) ;
#27633=CARTESIAN_POINT ( 'NONE',  ( 0.000000000000000000, -162.6242368362065918, 44.16213414209531862 ) ) ;
#27634=DIRECTION ( 'NONE',  ( 0.000000000000000000, 0.000000000000000000, -1.000000000000000000 ) ) ;
#27635=DIRECTION ( 'NONE',  ( 1.043714542225393539E-14, 0.4647231720437573488, -0.8854560256532157947 ) ) ;
#27637=ADVANCED_FACE ( 'NONE', ( #21278 ), #37296, .F. ) ;
#27638=VECTOR ( 'NONE', #26144, 1000.000000000000000 ) ;
#27644=DIRECTION ( 'NONE',  ( -1.000000000000000000, -0.000000000000000000, 0.000000000000000000 ) ) ;
#27645=PLANE ( 'NONE',  #33289 ) ;
#27648=FACE_OUTER_BOUND ( 'NONE', #12175, .T. ) ;
#27649=CARTESIAN_POINT ( 'NONE',  ( -339.1964088526558498, -178.4886558749180949, 21.38919645685277970 ) ) ;
#27650=ORIENTED_EDGE ( 'NONE', *, *, #36252, .F. ) ;
#27651=FACE_OUTER_BOUND ( 'NONE', #14969, .T. ) ;
#27660=DIRECTION ( 'NONE',  ( 0.000000000000000000, 0.000000000000000000, 1.000000000000000000 ) ) ;
#27661=CARTESIAN_POINT ( 'NONE',  ( 0.000000000000000000, -178.6659583184396354, -20.92168833550928042 ) ) ;
#27668=PLANE ( 'NONE',  #26609 ) ;
#27671=ORIENTED_EDGE ( 'NONE', *, *, #39408, .T. ) ;
#27674=ORIENTED_EDGE ( 'NONE', *, *, #10394, .T. ) ;
#27676=LINE ( 'NONE', #48175, #46843 ) ;
#27678=DIRECTION ( 'NONE',  ( 1.000000000000000000, 0.000000000000000000, 0.000000000000000000 ) ) ;
#27679=ORIENTED_EDGE ( 'NONE', *, *, #12917, .T. ) ;
#27681=ORIENTED_EDGE ( 'NONE', *, *, #40134, .F. ) ;
#27684=EDGE_CURVE ( 'NONE', #16500, #4879, #41773, .T. ) ;
#27685=DIRECTION ( 'NONE',  ( 0.000000000000000000, 0.000000000000000000, -1.000000000000000000 ) ) ;
#27690=DIRECTION ( 'NONE',  ( 0.000000000000000000, -0.6631226582407885317, 0.7485107481711069655 ) ) ;
#27702=DIRECTION ( 'NONE',  ( 1.000000000000000000, -0.000000000000000000, -0.000000000000000000 ) ) ;
#27709=LINE ( 'NONE', #3292, #44137 ) ;
#27713=ADVANCED_FACE ( 'NONE', ( #26765 ), #14682, .F. ) ;
#27715=CARTESIAN_POINT ( 'NONE',  ( -339.1964088526558498, -102.1108035431470427, 54.98865587491797413 ) ) ;
#27716=ORIENTED_EDGE ( 'NONE', *, *, #32043, .F. ) ;
#27718=VECTOR ( 'NONE', #19154, 1000.000000000000000 ) ;
#27720=CARTESIAN_POINT ( 'NONE',  ( -332.3517673607765914, -121.8677111499054320, 59.00000000000001421 ) ) ;
#27721=ORIENTED_EDGE ( 'NONE', *, *, #14816, .F. ) ;
#27726=EDGE_CURVE ( 'NONE', #13360, #29379, #45992, .T. ) ;
#27741=LINE ( 'NONE', #31693, #5865 ) ;
#27743=CARTESIAN_POINT ( 'NONE',  ( -336.3521761649653854, -169.4764303083190384, -38.55084767037274673 ) ) ;
#27744=CARTESIAN_POINT ( 'NONE',  ( -332.3517673607765914, -164.5945333327934463, -42.41660376256285048 ) ) ;
#27746=VERTEX_POINT ( 'NONE', #22302 ) ;
#27751=EDGE_LOOP ( 'NONE', ( #17720, #5682, #6644, #17821 ) ) ;
#27752=VECTOR ( 'NONE', #44305, 1000.000000000000000 ) ;
#27756=CARTESIAN_POINT ( 'NONE',  ( -339.1964088526558498, -157.4273119900853146, -48.27201571435997352 ) ) ;
#27757=ORIENTED_EDGE ( 'NONE', *, *, #39317, .F. ) ;
#27758=DIRECTION ( 'NONE',  ( -0.000000000000000000, 0.9927088740980538617, -0.1205366802553232974 ) ) ;
#27759=ORIENTED_EDGE ( 'NONE', *, *, #6337, .F. ) ;
#27767=DIRECTION ( 'NONE',  ( -1.000000000000000000, 0.000000000000000000, -0.000000000000000000 ) ) ;
#27768=ORIENTED_EDGE ( 'NONE', *, *, #32716, .T. ) ;
#27769=CARTESIAN_POINT ( 'NONE',  ( -339.1964088526558498, -79.66942718702553350, -39.49849221029258928 ) ) ;
#27774=VERTEX_POINT ( 'NONE', #18380 ) ;
#27778=DIRECTION ( 'NONE',  ( -0.000000000000000000, -0.8229838658936516893, 0.5680647467311626952 ) ) ;
#27779=EDGE_CURVE ( 'NONE', #32119, #30672, #42013, .T. ) ;
#27784=ADVANCED_FACE ( 'NONE', ( #13647 ), #26498, .F. ) ;
#27788=DIRECTION ( 'NONE',  ( -0.000000000000000000, 0.000000000000000000, 1.000000000000000000 ) ) ;
#27791=ORIENTED_EDGE ( 'NONE', *, *, #20480, .F. ) ;
#27793=ORIENTED_EDGE ( 'NONE', *, *, #15003, .T. ) ;
#27794=DIRECTION ( 'NONE',  ( 0.000000000000000000, 0.000000000000000000, 1.000000000000000000 ) ) ;
#27801=EDGE_LOOP ( 'NONE', ( #40385, #34229, #17759, #13049 ) ) ;
#27802=CARTESIAN_POINT ( 'NONE',  ( -336.3521761649653854, -107.5615171630107056, 57.84431488793861575 ) ) ;
#27813=PLANE ( 'NONE',  #35870 ) ;
#27817=ORIENTED_EDGE ( 'NONE', *, *, #4791, .F. ) ;
#27820=AXIS2_PLACEMENT_3D ( 'NONE', #13861, #26448, #18576 ) ;
#27832=CARTESIAN_POINT ( 'NONE',  ( -330.4913330509368166, -64.99044476834247064, -7.608018572113060429 ) ) ;
#27837=DIRECTION ( 'NONE',  ( 0.000000000000000000, 0.000000000000000000, 1.000000000000000000 ) ) ;
#27843=VERTEX_POINT ( 'NONE', #41041 ) ;
#27844=EDGE_CURVE ( 'NONE', #34734, #17876, #5056, .T. ) ;
#27846=CARTESIAN_POINT ( 'NONE',  ( -336.3521761649654422, -161.4024510877913485, 45.24454186338643780 ) ) ;
#27848=DIRECTION ( 'NONE',  ( -0.000000000000000000, 0.5680647467311540355, -0.8229838658936575735 ) ) ;
#27855=ORIENTED_EDGE ( 'NONE', *, *, #38181, .F. ) ;
#27856=VECTOR ( 'NONE', #29134, 1000.000000000000114 ) ;
#27857=VERTEX_POINT ( 'NONE', #17143 ) ;
#27862=ADVANCED_FACE ( 'NONE', ( #41831 ), #579, .T. ) ;
#27863=DIRECTION ( 'NONE',  ( 1.000000000000000000, 0.000000000000000000, 0.000000000000000000 ) ) ;
#27871=VECTOR ( 'NONE', #25453, 1000.000000000000000 ) ;
#27872=VERTEX_POINT ( 'NONE', #13455 ) ;
#27875=CARTESIAN_POINT ( 'NONE',  ( -339.1964088526558498, -73.83865025250274527, 33.67120938215247605 ) ) ;
#27877=EDGE_LOOP ( 'NONE', ( #12189, #20014, #16719, #5178 ) ) ;
#27880=DIRECTION ( 'NONE',  ( 0.000000000000000000, -6.753856733136369375E-14, -1.000000000000000000 ) ) ;
#27884=DIRECTION ( 'NONE',  ( 0.000000000000000000, 1.063963731932441632E-14, -1.000000000000000000 ) ) ;
#27886=ADVANCED_FACE ( 'NONE', ( #28682 ), #37359, .F. ) ;
#27887=ADVANCED_FACE ( 'NONE', ( #9510 ), #9258, .F. ) ;
#27888=EDGE_CURVE ( 'NONE', #29772, #8372, #49479, .T. ) ;
#27889=EDGE_LOOP ( 'NONE', ( #50913, #8122, #44021, #18148 ) ) ;
#27893=LINE ( 'NONE', #23956, #50814 ) ;
#27898=ORIENTED_EDGE ( 'NONE', *, *, #36803, .T. ) ;
#27899=AXIS2_PLACEMENT_3D ( 'NONE', #34056, #9625, #38247 ) ;
#27901=CARTESIAN_POINT ( 'NONE',  ( -305.0000000000000568, -173.1613497474968710, -33.67120938215310844 ) ) ;
#27911=DIRECTION ( 'NONE',  ( 0.000000000000000000, 2.567390744445674500E-14, 1.000000000000000000 ) ) ;
#27914=EDGE_LOOP ( 'NONE', ( #51987, #40364, #5723, #34361 ) ) ;
#27919=EDGE_CURVE ( 'NONE', #51592, #50821, #11046, .T. ) ;
#27920=CIRCLE ( 'NONE', #43008, 60.00000000000000000 ) ;
#27922=ORIENTED_EDGE ( 'NONE', *, *, #23139, .F. ) ;
#27931=VECTOR ( 'NONE', #26238, 1000.000000000000000 ) ;
#27932=ORIENTED_EDGE ( 'NONE', *, *, #1208, .T. ) ;
#27935=LINE ( 'NONE', #43965, #15721 ) ;
#27937=LINE ( 'NONE', #15611, #1412 ) ;
#27939=PLANE ( 'NONE',  #42159 ) ;
#27940=DIRECTION ( 'NONE',  ( 0.000000000000000000, 0.7485107481710999711, -0.6631226582407964143 ) ) ;
#27947=ORIENTED_EDGE ( 'NONE', *, *, #51670, .F. ) ;
#27948=ORIENTED_EDGE ( 'NONE', *, *, #1981, .F. ) ;
#27953=DIRECTION ( 'NONE',  ( 0.000000000000000000, -0.1205366802553303057, -0.9927088740980530845 ) ) ;
#27962=EDGE_CURVE ( 'NONE', #37621, #17577, #33784, .T. ) ;
#27966=DIRECTION ( 'NONE',  ( -1.000000000000000000, 0.000000000000000000, 0.000000000000000000 ) ) ;
#27972=AXIS2_PLACEMENT_3D ( 'NONE', #31836, #43911, #23940 ) ;
#27977=ORIENTED_EDGE ( 'NONE', *, *, #51654, .F. ) ;
#27979=PLANE ( 'NONE',  #43650 ) ;
#27982=ORIENTED_EDGE ( 'NONE', *, *, #11177, .F. ) ;
#27988=DIRECTION ( 'NONE',  ( -1.000000000000000000, -0.000000000000000000, 0.000000000000000000 ) ) ;
#27993=DIRECTION ( 'NONE',  ( -0.000000000000000000, -0.5680647467311485954, 0.8229838658936613482 ) ) ;
#27996=VERTEX_POINT ( 'NONE', #30770 ) ;
#27999=FACE_OUTER_BOUND ( 'NONE', #48328, .T. ) ;
#28000=PLANE ( 'NONE',  #25169 ) ;
#28002=FACE_BOUND ( 'NONE', #10911, .T. ) ;
#28003=LINE ( 'NONE', #15684, #14628 ) ;
#28004=VERTEX_POINT ( 'NONE', #6861 ) ;
#28005=CARTESIAN_POINT ( 'NONE',  ( -339.1964088526558498, -64.99044476834248485, -7.608018572113150135 ) ) ;
#28006=ORIENTED_EDGE ( 'NONE', *, *, #4476, .T. ) ;
#28014=LINE ( 'NONE', #12515, #36009 ) ;
#28016=CARTESIAN_POINT ( 'NONE',  ( -332.3517673607765914, -120.8677111499054320, 59.00000000000000000 ) ) ;
#28019=DIRECTION ( 'NONE',  ( -0.000000000000000000, -0.9927088740980530845, 0.1205366802553303057 ) ) ;
#28025=CARTESIAN_POINT ( 'NONE',  ( -336.3521761649654422, -98.41210887299327226, -53.46519113769058151 ) ) ;
#28027=ORIENTED_EDGE ( 'NONE', *, *, #23615, .F. ) ;
#28028=CARTESIAN_POINT ( 'NONE',  ( -336.3521761649654422, -111.7106844931459619, -58.83036664750484590 ) ) ;
#28029=CARTESIAN_POINT ( 'NONE',  ( -332.3517673607765914, -158.3591674452439122, -47.62880233550485087 ) ) ;
#28045=FACE_OUTER_BOUND ( 'NONE', #42049, .T. ) ;
#28046=EDGE_LOOP ( 'NONE', ( #46619, #3960, #5142, #30011 ) ) ;
#28054=AXIS2_PLACEMENT_3D ( 'NONE', #17976, #34756, #2192 ) ;
#28055=EDGE_CURVE ( 'NONE', #15026, #24837, #24190, .T. ) ;
#28058=FACE_OUTER_BOUND ( 'NONE', #10183, .T. ) ;
#28060=ORIENTED_EDGE ( 'NONE', *, *, #22399, .T. ) ;
#28063=VERTEX_POINT ( 'NONE', #19980 ) ;
#28067=CARTESIAN_POINT ( 'NONE',  ( -336.3521761649654422, -64.61288906875131488, 4.498567634385603142 ) ) ;
#28071=VECTOR ( 'NONE', #2159, 1000.000000000000000 ) ;
#28072=VERTEX_POINT ( 'NONE', #47848 ) ;
#28073=EDGE_CURVE ( 'NONE', #7018, #19848, #43886, .T. ) ;
#28077=CARTESIAN_POINT ( 'NONE',  ( -336.3521761649654422, -125.1322888500942270, -59.00000000000002132 ) ) ;
#28078=CARTESIAN_POINT ( 'NONE',  ( -332.3517673607765914, -100.1170788342122080, 54.23253582808833073 ) ) ;
#28079=FACE_OUTER_BOUND ( 'NONE', #13794, .T. ) ;
#28081=CARTESIAN_POINT ( 'NONE',  ( -336.3521761649654422, -127.9985676343858501, 58.88711093124869222 ) ) ;
#28082=ORIENTED_EDGE ( 'NONE', *, *, #35915, .F. ) ;
#28091=CIRCLE ( 'NONE', #18059, 60.00000000000000000 ) ;
#28096=ORIENTED_EDGE ( 'NONE', *, *, #31929, .T. ) ;
#28099=( GEOMETRIC_REPRESENTATION_CONTEXT ( 3 ) GLOBAL_UNCERTAINTY_ASSIGNED_CONTEXT ( ( #21695 ) ) GLOBAL_UNIT_ASSIGNED_CONTEXT ( ( #7587, #3638, #32798 ) ) REPRESENTATION_CONTEXT ( 'NONE', 'WORKASPACE' ) );
#28103=ORIENTED_EDGE ( 'NONE', *, *, #7353, .F. ) ;
#28104=VECTOR ( 'NONE', #23871, 999.9999999999998863 ) ;
#28105=CARTESIAN_POINT ( 'NONE',  ( -332.3517673607765914, -123.5000000000000284, 0.000000000000000000 ) ) ;
#28112=EDGE_CURVE ( 'NONE', #13761, #38315, #17033, .T. ) ;
#28116=FACE_OUTER_BOUND ( 'NONE', #9465, .T. ) ;
#28122=VECTOR ( 'NONE', #46855, 1000.000000000000000 ) ;
#28123=ORIENTED_EDGE ( 'NONE', *, *, #36259, .F. ) ;
#28124=DIRECTION ( 'NONE',  ( 0.000000000000000000, -0.4647231720437604574, 0.8854560256532141294 ) ) ;
#28129=DIRECTION ( 'NONE',  ( -0.000000000000000000, 0.2393156642875685636, 0.9709418174260492362 ) ) ;
#28130=DIRECTION ( 'NONE',  ( 1.000000000000000000, -0.000000000000000000, 0.000000000000000000 ) ) ;
#28140=VECTOR ( 'NONE', #50145, 1000.000000000000000 ) ;
#28141=LINE ( 'NONE', #8441, #21615 ) ;
#28143=VECTOR ( 'NONE', #14192, 1000.000000000000000 ) ;
#28149=DIRECTION ( 'NONE',  ( 0.000000000000000000, 0.000000000000000000, -1.000000000000000000 ) ) ;
#28150=AXIS2_PLACEMENT_3D ( 'NONE', #43474, #31370, #40023 ) ;
#28156=CARTESIAN_POINT ( 'NONE',  ( -332.3517673607765914, -123.5000000000000284, 0.000000000000000000 ) ) ;
#28157=CARTESIAN_POINT ( 'NONE',  ( -332.3517673607765914, -181.8730728925770563, 8.732051761644092025 ) ) ;
#28162=LINE ( 'NONE', #20288, #26413 ) ;
#28169=EDGE_CURVE ( 'NONE', #16821, #37730, #47594, .T. ) ;
#28173=AXIS2_PLACEMENT_3D ( 'NONE', #13943, #45744, #9483 ) ;
#28174=VERTEX_POINT ( 'NONE', #7632 ) ;
#28175=CARTESIAN_POINT ( 'NONE',  ( 0.000000000000000000, -180.7855672281372108, -14.11962419296555105 ) ) ;
#28183=VERTEX_POINT ( 'NONE', #1033 ) ;
#28189=PLANE ( 'NONE',  #51804 ) ;
#28192=DIRECTION ( 'NONE',  ( 0.000000000000000000, 0.000000000000000000, 1.000000000000000000 ) ) ;
#28195=DIRECTION ( 'NONE',  ( -0.000000000000000000, -0.6631226582407885317, 0.7485107481711069655 ) ) ;
#28196=ADVANCED_FACE ( 'NONE', ( #5260 ), #8410, .F. ) ;
#28198=LINE ( 'NONE', #3777, #12286 ) ;
#28199=ADVANCED_FACE ( 'NONE', ( #25476 ), #1297, .T. ) ;
#28202=VERTEX_POINT ( 'NONE', #17610 ) ;
#28203=LINE ( 'NONE', #43985, #16418 ) ;
#28206=FACE_OUTER_BOUND ( 'NONE', #39337, .T. ) ;
#28210=AXIS2_PLACEMENT_3D ( 'NONE', #51002, #46285, #14731 ) ;
#28213=ORIENTED_EDGE ( 'NONE', *, *, #17974, .F. ) ;
#28214=DIRECTION ( 'NONE',  ( 1.000000000000000000, 8.718379230999705894E-17, -3.044005838999302267E-31 ) ) ;
#28215=EDGE_CURVE ( 'NONE', #42588, #38711, #41492, .T. ) ;
#28218=ORIENTED_EDGE ( 'NONE', *, *, #5028, .T. ) ;
#28227=PLANE ( 'NONE',  #15479 ) ;
#28228=DIRECTION ( 'NONE',  ( 1.000000000000000000, 0.000000000000000000, 0.000000000000000000 ) ) ;
#28229=VECTOR ( 'NONE', #45494, 1000.000000000000114 ) ;
#28233=CARTESIAN_POINT ( 'NONE',  ( -339.1964088526558498, -182.1300919119129560, -6.615309698014600670 ) ) ;
#28236=AXIS2_PLACEMENT_3D ( 'NONE', #29687, #9470, #1588 ) ;
#28238=DIRECTION ( 'NONE',  ( 0.000000000000000000, -0.9927088740980530845, 0.1205366802553303196 ) ) ;
#28240=ORIENTED_EDGE ( 'NONE', *, *, #21660, .T. ) ;
#28243=AXIS2_PLACEMENT_3D ( 'NONE', #41679, #5705, #38249 ) ;
#28245=EDGE_LOOP ( 'NONE', ( #8145, #33379, #25426, #51128 ) ) ;
#28246=CARTESIAN_POINT ( 'NONE',  ( -339.1964088526558498, -96.52406086224443982, -52.47426709956138069 ) ) ;
#28247=DIRECTION ( 'NONE',  ( 0.000000000000000000, 1.882753212593494549E-13, -1.000000000000000000 ) ) ;
#28251=CIRCLE ( 'NONE', #40813, 60.00000000000000000 ) ;
#28252=EDGE_CURVE ( 'NONE', #49023, #32161, #27920, .T. ) ;
#28257=VERTEX_POINT ( 'NONE', #33370 ) ;
#28258=EDGE_CURVE ( 'NONE', #21618, #24982, #785, .T. ) ;
#28259=ORIENTED_EDGE ( 'NONE', *, *, #40082, .T. ) ;
#28267=FACE_BOUND ( 'NONE', #33195, .T. ) ;
#28268=VECTOR ( 'NONE', #1929, 1000.000000000000000 ) ;
#28269=CARTESIAN_POINT ( 'NONE',  ( -330.4913330509368166, -176.3931552210903249, -28.32515014536811293 ) ) ;
#28272=ORIENTED_EDGE ( 'NONE', *, *, #34965, .T. ) ;
#28273=CARTESIAN_POINT ( 'NONE',  ( -339.1964088526558498, -175.9742670995615015, -26.97593913775538965 ) ) ;
#28274=ORIENTED_EDGE ( 'NONE', *, *, #50094, .F. ) ;
#28280=PLANE ( 'NONE',  #14191 ) ;
#28288=VECTOR ( 'NONE', #30500, 1000.000000000000227 ) ;
#28289=DIRECTION ( 'NONE',  ( 0.000000000000000000, -2.659909329831104317E-14, -1.000000000000000000 ) ) ;
#28299=CIRCLE ( 'NONE', #40902, 60.00000000000000000 ) ;
#28303=DIRECTION ( 'NONE',  ( 0.000000000000000000, 0.5680647467311540355, -0.8229838658936575735 ) ) ;
#28307=AXIS2_PLACEMENT_3D ( 'NONE', #28694, #40263, #8734 ) ;
#28311=CARTESIAN_POINT ( 'NONE',  ( -339.1964088526558498, -123.5000000000000284, 0.000000000000000000 ) ) ;
#28312=CARTESIAN_POINT ( 'NONE',  ( -339.1964088526558498, -162.9984922102927385, -43.83057281297435992 ) ) ;
#28314=EDGE_CURVE ( 'NONE', #1525, #10115, #4596, .T. ) ;
#28316=ORIENTED_EDGE ( 'NONE', *, *, #51366, .F. ) ;
#28328=PLANE ( 'NONE',  #14697 ) ;
#28329=ORIENTED_EDGE ( 'NONE', *, *, #9915, .T. ) ;
#28332=EDGE_CURVE ( 'NONE', #6252, #5943, #5129, .T. ) ;
#28340=FACE_OUTER_BOUND ( 'NONE', #10258, .T. ) ;
#28342=ORIENTED_EDGE ( 'NONE', *, *, #51775, .T. ) ;
#28343=ADVANCED_FACE ( 'NONE', ( #30069 ), #50054, .F. ) ;
#28348=FACE_OUTER_BOUND ( 'NONE', #49062, .T. ) ;
#28352=ORIENTED_EDGE ( 'NONE', *, *, #51349, .T. ) ;
#28357=DIRECTION ( 'NONE',  ( -0.000000000000000000, 0.5680647467311656929, 0.8229838658936495799 ) ) ;
#28366=ORIENTED_EDGE ( 'NONE', *, *, #19145, .T. ) ;
#28369=DIRECTION ( 'NONE',  ( -0.000000000000000000, 0.4647231720437573488, -0.8854560256532157947 ) ) ;
#28373=ORIENTED_EDGE ( 'NONE', *, *, #21961, .F. ) ;
#28374=EDGE_CURVE ( 'NONE', #8829, #18239, #21144, .T. ) ;
#28375=EDGE_CURVE ( 'NONE', #45414, #7213, #41116, .T. ) ;
#28379=ORIENTED_EDGE ( 'NONE', *, *, #3102, .F. ) ;
#28380=EDGE_CURVE ( 'NONE', #15465, #50694, #33505, .T. ) ;
#28386=LINE ( 'NONE', #8424, #4005 ) ;
#28391=CARTESIAN_POINT ( 'NONE',  ( -330.4913330509368166, -137.3729703655840524, -58.37414404713467064 ) ) ;
#28394=CARTESIAN_POINT ( 'NONE',  ( -339.1964088526558498, -108.8949048983204051, 57.16590939599314680 ) ) ;
#28395=VECTOR ( 'NONE', #40210, 1000.000000000000000 ) ;
#28403=CARTESIAN_POINT ( 'NONE',  ( -305.0000000000000568, -63.55776901541228341, -2.632288850093980503 ) ) ;
#28405=( NAMED_UNIT ( * ) SI_UNIT ( $, .STERADIAN. ) SOLID_ANGLE_UNIT ( ) );
#28406=ORIENTED_EDGE ( 'NONE', *, *, #8005, .T. ) ;
#28407=CARTESIAN_POINT ( 'NONE',  ( -336.3521761649654422, -106.8245764869328980, 56.65561927337994064 ) ) ;
#28413=ORIENTED_EDGE ( 'NONE', *, *, #48297, .T. ) ;
#28419=ADVANCED_FACE ( 'NONE', ( #49275 ), #13268, .T. ) ;
#28425=DIRECTION ( 'NONE',  ( 1.000000000000000000, -0.000000000000000000, -0.000000000000000000 ) ) ;
#28428=ORIENTED_EDGE ( 'NONE', *, *, #29400, .T. ) ;
#28432=ADVANCED_FACE ( 'NONE', ( #9842 ), #29015, .F. ) ;
#28442=CARTESIAN_POINT ( 'NONE',  ( -339.1964088526558498, -89.82879061784706209, -49.66134974749692788 ) ) ;
#28446=VECTOR ( 'NONE', #46531, 1000.000000000000000 ) ;
#28448=FACE_OUTER_BOUND ( 'NONE', #42819, .T. ) ;
#28451=CARTESIAN_POINT ( 'NONE',  ( -339.1964088526558498, -167.9936954712156592, -38.74998146212110584 ) ) ;
#28452=DIRECTION ( 'NONE',  ( 1.000000000000000000, 0.000000000000000000, 0.000000000000000000 ) ) ;
#28454=LINE ( 'NONE', #24004, #338 ) ;
#28456=FACE_OUTER_BOUND ( 'NONE', #45015, .T. ) ;
#28458=ORIENTED_EDGE ( 'NONE', *, *, #37226, .F. ) ;
#28465=AXIS2_PLACEMENT_3D ( 'NONE', #41963, #38017, #2549 ) ;
#28466=DIRECTION ( 'NONE',  ( 1.000000000000000000, -0.000000000000000000, -0.000000000000000000 ) ) ;
#28470=VERTEX_POINT ( 'NONE', #21675 ) ;
#28476=CARTESIAN_POINT ( 'NONE',  ( -339.1964088526558498, -95.63860483659122735, -52.00954392751761191 ) ) ;
#28480=ADVANCED_FACE ( 'NONE', ( #5911 ), #37949, .T. ) ;
#28486=VERTEX_POINT ( 'NONE', #2210 ) ;
#28492=ADVANCED_FACE ( 'NONE', ( #30569 ), #18757, .F. ) ;
#28498=DIRECTION ( 'NONE',  ( -0.000000000000000000, 0.000000000000000000, 1.000000000000000000 ) ) ;
#28505=DIRECTION ( 'NONE',  ( 0.000000000000000000, 8.349802331035031902E-14, 1.000000000000000000 ) ) ;
#28506=EDGE_CURVE ( 'NONE', #21379, #32832, #2475, .T. ) ;
#28507=DIRECTION ( 'NONE',  ( 0.000000000000000000, 0.4647231720437631775, -0.8854560256532126861 ) ) ;
#28510=ORIENTED_EDGE ( 'NONE', *, *, #13722, .T. ) ;
#28511=EDGE_LOOP ( 'NONE', ( #39494, #50327, #50463, #47465 ) ) ;
#28513=DIRECTION ( 'NONE',  ( 1.000000000000000000, -0.000000000000000000, -0.000000000000000000 ) ) ;
#28515=FACE_BOUND ( 'NONE', #5221, .T. ) ;
#28529=ORIENTED_EDGE ( 'NONE', *, *, #3504, .F. ) ;
#28530=PLANE ( 'NONE',  #11597 ) ;
#28533=ORIENTED_EDGE ( 'NONE', *, *, #11280, .T. ) ;
#28536=CARTESIAN_POINT ( 'NONE',  ( -339.1964088526558498, -71.49045607248255862, -27.86139516340906397 ) ) ;
#28540=ADVANCED_FACE ( 'NONE', ( #42408 ), #14565, .F. ) ;
#28542=DIRECTION ( 'NONE',  ( -1.000000000000000000, -0.000000000000000000, -0.000000000000000000 ) ) ;
#28544=EDGE_CURVE ( 'NONE', #47197, #32221, #2719, .T. ) ;
#28547=CARTESIAN_POINT ( 'NONE',  ( -330.4913330509368166, -84.00150778970706256, 43.83057281297416097 ) ) ;
#28554=VERTEX_POINT ( 'NONE', #31871 ) ;
#28559=VERTEX_POINT ( 'NONE', #3745 ) ;
#28564=EDGE_CURVE ( 'NONE', #21974, #17216, #15376, .T. ) ;
#28565=CARTESIAN_POINT ( 'NONE',  ( -339.1964088526558498, -109.8658467157473666, -57.40522506028092664 ) ) ;
#28576=DIRECTION ( 'NONE',  ( -1.000000000000000000, 0.000000000000000000, 0.000000000000000000 ) ) ;
#28580=DIRECTION ( 'NONE',  ( 1.000000000000000000, -0.000000000000000000, 0.000000000000000000 ) ) ;
#28581=DIRECTION ( 'NONE',  ( -1.000000000000000000, -0.000000000000000000, 0.000000000000000000 ) ) ;
#28584=DIRECTION ( 'NONE',  ( 0.000000000000000000, 0.000000000000000000, -1.000000000000000000 ) ) ;
#28585=EDGE_LOOP ( 'NONE', ( #12720, #5653 ) ) ;
#28586=EDGE_LOOP ( 'NONE', ( #42538, #47090, #30618, #10906 ) ) ;
#28589=DIRECTION ( 'NONE',  ( -1.000000000000000000, -0.000000000000000000, -0.000000000000000000 ) ) ;
#28591=ORIENTED_EDGE ( 'NONE', *, *, #50402, .T. ) ;
#28592=CARTESIAN_POINT ( 'NONE',  ( -339.1964088526558498, -137.1341532842523065, 57.40522506028101901 ) ) ;
#28600=CARTESIAN_POINT ( 'NONE',  ( 0.000000000000000000, -74.94395191227387443, 33.51582005713760282 ) ) ;
#28601=DIRECTION ( 'NONE',  ( -0.000000000000000000, -0.9927088740980548609, -0.1205366802553164696 ) ) ;
#28604=FACE_OUTER_BOUND ( 'NONE', #45722, .T. ) ;
#28616=CARTESIAN_POINT ( 'NONE',  ( 0.000000000000000000, -116.3883358649361526, -58.56982357178523557 ) ) ;
#28619=ORIENTED_EDGE ( 'NONE', *, *, #22461, .F. ) ;
#28626=CARTESIAN_POINT ( 'NONE',  ( -332.3517673607765914, -76.43926241122620979, -35.68215131113738181 ) ) ;
#28629=CARTESIAN_POINT ( 'NONE',  ( -332.3517673607765914, -123.5000000000000284, 0.000000000000000000 ) ) ;
#28632=EDGE_CURVE ( 'NONE', #19724, #13689, #16365, .T. ) ;
#28636=VERTEX_POINT ( 'NONE', #66 ) ;
#28640=DIRECTION ( 'NONE',  ( 0.000000000000000000, 0.000000000000000000, -1.000000000000000000 ) ) ;
#28641=CARTESIAN_POINT ( 'NONE',  ( -336.3521761649654422, -81.08339623743702873, -41.09453333279329712 ) ) ;
#28643=EDGE_LOOP ( 'NONE', ( #50554, #30071, #19512, #40111 ) ) ;
#28647=PLANE ( 'NONE',  #47397 ) ;
#28650=DIRECTION ( 'NONE',  ( -0.000000000000000000, -0.1205366802553130001, 0.9927088740980551940 ) ) ;
#28651=CARTESIAN_POINT ( 'NONE',  ( -332.3517673607765914, -174.3267994849386184, -31.88473700876087591 ) ) ;
#28656=DIRECTION ( 'NONE',  ( -0.000000000000000000, -0.3546048870425267951, 0.9350162426854181641 ) ) ;
#28658=CARTESIAN_POINT ( 'NONE',  ( -332.3517673607765914, -179.2447759217480154, -19.39547174791710660 ) ) ;
#28661=CARTESIAN_POINT ( 'NONE',  ( -336.3521761649654422, -86.34605966037949543, -45.90766452162698386 ) ) ;
#28666=VECTOR ( 'NONE', #47180, 1000.000000000000000 ) ;
#28670=ORIENTED_EDGE ( 'NONE', *, *, #43323, .F. ) ;
#28673=LINE ( 'NONE', #29212, #40294 ) ;
#28682=FACE_OUTER_BOUND ( 'NONE', #19693, .T. ) ;
#28685=ORIENTED_EDGE ( 'NONE', *, *, #26594, .T. ) ;
#28688=VERTEX_POINT ( 'NONE', #7942 ) ;
#28689=ORIENTED_EDGE ( 'NONE', *, *, #8774, .F. ) ;
#28692=AXIS2_PLACEMENT_3D ( 'NONE', #20012, #48664, #16079 ) ;
#28694=CARTESIAN_POINT ( 'NONE',  ( -332.3517673607765914, -64.50000000000000000, -2.632288850093980503 ) ) ;
#28696=ORIENTED_EDGE ( 'NONE', *, *, #31097, .F. ) ;
#28698=FACE_OUTER_BOUND ( 'NONE', #17295, .T. ) ;
#28704=ORIENTED_EDGE ( 'NONE', *, *, #18240, .F. ) ;
#28707=EDGE_CURVE ( 'NONE', #11608, #28063, #44742, .T. ) ;
#28710=DIRECTION ( 'NONE',  ( -1.000000000000000000, 0.000000000000000000, 0.000000000000000000 ) ) ;
#28711=VECTOR ( 'NONE', #256, 1000.000000000000000 ) ;
#28712=AXIS2_PLACEMENT_3D ( 'NONE', #45627, #41924, #37726 ) ;
#28714=ORIENTED_EDGE ( 'NONE', *, *, #45833, .T. ) ;
#28719=DIRECTION ( 'NONE',  ( -8.718379230999708359E-17, 0.6631226582407965253, 0.7485107481711000821 ) ) ;
#28720=ORIENTED_EDGE ( 'NONE', *, *, #13147, .F. ) ;
#28723=ORIENTED_EDGE ( 'NONE', *, *, #12545, .T. ) ;
#28727=CARTESIAN_POINT ( 'NONE',  ( -332.3517673607765914, -78.25545813661345562, 37.90245108779119931 ) ) ;
#28731=ADVANCED_FACE ( 'NONE', ( #45014 ), #37364, .F. ) ;
#28735=DIRECTION ( 'NONE',  ( 0.000000000000000000, -0.2393156642875482465, 0.9709418174260544543 ) ) ;
#28737=DIRECTION ( 'NONE',  ( -0.000000000000000000, -0.8229838658936575735, -0.5680647467311540355 ) ) ;
#28743=EDGE_LOOP ( 'NONE', ( #20265, #32070, #9349, #42815 ) ) ;
#28744=ADVANCED_FACE ( 'NONE', ( #32895 ), #13980, .T. ) ;
#28748=VERTEX_POINT ( 'NONE', #9006 ) ;
#28755=CARTESIAN_POINT ( 'NONE',  ( -332.3517673607765914, -123.5000000000000284, 0.000000000000000000 ) ) ;
#28764=EDGE_LOOP ( 'NONE', ( #1373, #21762, #43250, #36370 ) ) ;
#28765=DIRECTION ( 'NONE',  ( -1.000000000000000000, 0.000000000000000000, -0.000000000000000000 ) ) ;
#28768=FACE_BOUND ( 'NONE', #16054, .T. ) ;
#28772=EDGE_CURVE ( 'NONE', #45713, #14384, #17679, .T. ) ;
#28779=CARTESIAN_POINT ( 'NONE',  ( -330.4913330509368166, -123.9999999999993605, 59.99791663049644086 ) ) ;
#28780=CARTESIAN_POINT ( 'NONE',  ( -339.1964088526558498, -138.3439121830101328, -58.13482838284710397 ) ) ;
#28784=DIRECTION ( 'NONE',  ( -0.000000000000000000, -0.1205366802553130001, 0.9927088740980551940 ) ) ;
#28786=ORIENTED_EDGE ( 'NONE', *, *, #31346, .T. ) ;
#28796=CARTESIAN_POINT ( 'NONE',  ( -332.3517673607765914, -166.6218737817864621, 41.71934804797023588 ) ) ;
#28810=VECTOR ( 'NONE', #32565, 999.9999999999998863 ) ;
#28811=PLANE ( 'NONE',  #47934 ) ;
#28815=AXIS2_PLACEMENT_3D ( 'NONE', #5244, #1276, #25206 ) ;
#28816=CARTESIAN_POINT ( 'NONE',  ( -330.4913330509368166, -151.3613951634091848, -52.00954392751743427 ) ) ;
#28817=LINE ( 'NONE', #44866, #34347 ) ;
#28819=ORIENTED_EDGE ( 'NONE', *, *, #48348, .F. ) ;
#28820=DIRECTION ( 'NONE',  ( -0.000000000000000000, -0.9709418174260534551, -0.2393156642875516327 ) ) ;
#28821=VECTOR ( 'NONE', #51551, 1000.000000000000000 ) ;
#28822=ORIENTED_EDGE ( 'NONE', *, *, #17935, .T. ) ;
#28824=EDGE_CURVE ( 'NONE', #4373, #30471, #4809, .T. ) ;
#28825=DIRECTION ( 'NONE',  ( -0.000000000000000000, -0.8854560256532062468, 0.4647231720437755564 ) ) ;
#28845=ORIENTED_EDGE ( 'NONE', *, *, #1920, .F. ) ;
#28846=CARTESIAN_POINT ( 'NONE',  ( -339.1964088526558498, -70.60684477890995936, -28.32515014536858189 ) ) ;
#28853=CARTESIAN_POINT ( 'NONE',  ( -339.1964088526558498, -157.1712093821526821, 49.66134974749714104 ) ) ;
#28855=AXIS2_PLACEMENT_3D ( 'NONE', #2331, #3089, #18360 ) ;
#28859=CARTESIAN_POINT ( 'NONE',  ( -339.1964088526558498, -122.9999999999993747, 59.00000000000002132 ) ) ;
#28864=CARTESIAN_POINT ( 'NONE',  ( -332.3517673607765914, -166.5797264208035244, 40.34602258462248159 ) ) ;
#28869=LINE ( 'NONE', #44917, #304 ) ;
#28870=CARTESIAN_POINT ( 'NONE',  ( -330.4913330509368166, -70.14212160686581399, 27.43969411971463046 ) ) ;
#28873=ORIENTED_EDGE ( 'NONE', *, *, #20480, .T. ) ;
#28874=VERTEX_POINT ( 'NONE', #34211 ) ;
#28881=EDGE_CURVE ( 'NONE', #47910, #36663, #30776, .T. ) ;
#28882=CARTESIAN_POINT ( 'NONE',  ( -339.1964088526558498, -156.6043281241909426, 48.84008046109164525 ) ) ;
#28886=VECTOR ( 'NONE', #1904, 1000.000000000000000 ) ;
#28892=CIRCLE ( 'NONE', #43155, 60.00000000000000000 ) ;
#28895=PLANE ( 'NONE',  #20844 ) ;
#28896=EDGE_LOOP ( 'NONE', ( #11464, #36176, #12456, #40025 ) ) ;
#28906=CARTESIAN_POINT ( 'NONE',  ( -336.3521761649654422, -171.1288023355047585, 34.85916744524404720 ) ) ;
#28909=VERTEX_POINT ( 'NONE', #10805 ) ;
#28911=CARTESIAN_POINT ( 'NONE',  ( -305.0000000000000568, -65.65568511206123503, -15.93848283698870105 ) ) ;
#28912=ORIENTED_EDGE ( 'NONE', *, *, #17504, .F. ) ;
#28920=EDGE_CURVE ( 'NONE', #43333, #11713, #10293, .T. ) ;
#28923=PLANE ( 'NONE',  #19865 ) ;
#28937=LINE ( 'NONE', #8987, #25211 ) ;
#28938=FACE_OUTER_BOUND ( 'NONE', #50167, .T. ) ;
#28945=ORIENTED_EDGE ( 'NONE', *, *, #32358, .T. ) ;
#28951=EDGE_LOOP ( 'NONE', ( #39331, #29716, #7168, #14749 ) ) ;
#28953=AXIS2_PLACEMENT_3D ( 'NONE', #11263, #11536, #11782 ) ;
#28954=VECTOR ( 'NONE', #34378, 1000.000000000000000 ) ;
#28961=DIRECTION ( 'NONE',  ( -0.000000000000000000, -0.5680647467311569221, -0.8229838658936556861 ) ) ;
#28963=EDGE_LOOP ( 'NONE', ( #14064, #17124, #10432, #14577 ) ) ;
#28964=AXIS2_PLACEMENT_3D ( 'NONE', #36999, #995, #49098 ) ;
#28969=ORIENTED_EDGE ( 'NONE', *, *, #11177, .T. ) ;
#28970=DIRECTION ( 'NONE',  ( 0.000000000000000000, 0.000000000000000000, 1.000000000000000000 ) ) ;
#28976=CARTESIAN_POINT ( 'NONE',  ( -336.3521761649654422, -181.8730728925770563, 8.732051761644092025 ) ) ;
#28977=DIRECTION ( 'NONE',  ( 0.000000000000000000, 0.000000000000000000, 1.000000000000000000 ) ) ;
#28982=ORIENTED_EDGE ( 'NONE', *, *, #32378, .T. ) ;
#28984=DIRECTION ( 'NONE',  ( -1.000000000000000000, 0.000000000000000000, 0.000000000000000000 ) ) ;
#28986=DIRECTION ( 'NONE',  ( -1.000000000000000000, -0.000000000000000000, -0.000000000000000000 ) ) ;
#28987=EDGE_LOOP ( 'NONE', ( #38028, #40851, #33052, #30495 ) ) ;
#28991=DIRECTION ( 'NONE',  ( 1.000000000000000000, 0.000000000000000000, -0.000000000000000000 ) ) ;
#28997=CARTESIAN_POINT ( 'NONE',  ( -170.0000000000000284, -123.5000000000000284, 0.000000000000000000 ) ) ;
#29000=VERTEX_POINT ( 'NONE', #37284 ) ;
#29004=ADVANCED_FACE ( 'NONE', ( #49125 ), #45444, .F. ) ;
#29005=VECTOR ( 'NONE', #4763, 1000.000000000000000 ) ;
#29006=CARTESIAN_POINT ( 'NONE',  ( -336.3521761649654422, -82.40546666720629787, 42.41660376256258047 ) ) ;
#29009=AXIS2_PLACEMENT_3D ( 'NONE', #35087, #11158, #6724 ) ;
#29010=EDGE_LOOP ( 'NONE', ( #3091, #12976, #14985, #37196 ) ) ;
#29012=AXIS2_PLACEMENT_3D ( 'NONE', #51827, #36, #27880 ) ;
#29013=EDGE_CURVE ( 'NONE', #11736, #16530, #22123, .T. ) ;
#29014=VECTOR ( 'NONE', #42942, 1000.000000000000000 ) ;
#29015=PLANE ( 'NONE',  #12011 ) ;
#29017=ORIENTED_EDGE ( 'NONE', *, *, #25379, .T. ) ;
#29020=CARTESIAN_POINT ( 'NONE',  ( -339.1964088526558498, -123.5000000000000284, 0.000000000000000000 ) ) ;
#29022=EDGE_CURVE ( 'NONE', #45092, #26309, #14165, .T. ) ;
#29025=ORIENTED_EDGE ( 'NONE', *, *, #49646, .T. ) ;
#29029=PLANE ( 'NONE',  #36941 ) ;
#29031=AXIS2_PLACEMENT_3D ( 'NONE', #11801, #3941, #43368 ) ;
#29035=CARTESIAN_POINT ( 'NONE',  ( -330.4913330509368166, -173.1613497474965300, 33.67120938215357029 ) ) ;
#29050=DIRECTION ( 'NONE',  ( -0.000000000000000000, -0.9350162426854169428, -0.3546048870425300148 ) ) ;
#29051=VERTEX_POINT ( 'NONE', #13630 ) ;
#29052=DIRECTION ( 'NONE',  ( 1.000000000000000000, -0.000000000000000000, 0.000000000000000000 ) ) ;
#29053=VECTOR ( 'NONE', #38010, 1000.000000000000000 ) ;
#29061=DIRECTION ( 'NONE',  ( 1.000000000000000000, -0.000000000000000000, -0.000000000000000000 ) ) ;
#29065=PLANE ( 'NONE',  #4742 ) ;
#29066=PLANE ( 'NONE',  #1815 ) ;
#29071=LINE ( 'NONE', #25918, #34000 ) ;
#29074=DIRECTION ( 'NONE',  ( 0.000000000000000000, 0.000000000000000000, -1.000000000000000000 ) ) ;
#29077=EDGE_CURVE ( 'NONE', #47681, #38828, #34119, .T. ) ;
#29089=CARTESIAN_POINT ( 'NONE',  ( -332.3517673607765914, -128.1121410293017391, 59.82247199109905011 ) ) ;
#29097=VERTEX_POINT ( 'NONE', #13110 ) ;
#29103=DIRECTION ( 'NONE',  ( 0.000000000000000000, 0.000000000000000000, -1.000000000000000000 ) ) ;
#29104=CARTESIAN_POINT ( 'NONE',  ( -336.3521761649654422, -165.9166037625627439, 41.09453333279358134 ) ) ;
#29109=CIRCLE ( 'NONE', #24922, 60.00000000000000000 ) ;
#29114=DIRECTION ( 'NONE',  ( -1.000000000000000000, -0.000000000000000000, -0.000000000000000000 ) ) ;
#29116=AXIS2_PLACEMENT_3D ( 'NONE', #24494, #20553, #32377 ) ;
#29117=LINE ( 'NONE', #25191, #26332 ) ;
#29120=CARTESIAN_POINT ( 'NONE',  ( -305.0000000000000568, -131.2283041299240836, 59.50019592636143528 ) ) ;
#29121=VERTEX_POINT ( 'NONE', #29133 ) ;
#29123=CARTESIAN_POINT ( 'NONE',  ( -332.3517673607765914, -182.5000000000000568, 1.632288850093980725 ) ) ;
#29125=DIRECTION ( 'NONE',  ( -1.000000000000000000, 0.000000000000000000, -0.000000000000000000 ) ) ;
#29126=AXIS2_PLACEMENT_3D ( 'NONE', #29242, #20572, #36606 ) ;
#29127=CARTESIAN_POINT ( 'NONE',  ( -336.3521761649654422, -70.03480886230919111, 25.08789112700620194 ) ) ;
#29128=CARTESIAN_POINT ( 'NONE',  ( -365.0000000000001137, -168.5000000000000284, 5.000000000000001776 ) ) ;
#29133=CARTESIAN_POINT ( 'NONE',  ( -336.3521761649654422, -149.0257676989619142, 54.29949524055110999 ) ) ;
#29134=DIRECTION ( 'NONE',  ( 0.000000000000000000, -0.3546048870425426158, -0.9350162426854120579 ) ) ;
#29136=CARTESIAN_POINT ( 'NONE',  ( 0.000000000000000000, -109.3803758070342838, -57.28556722813713975 ) ) ;
#29141=EDGE_CURVE ( 'NONE', #40004, #12706, #33030, .T. ) ;
#29147=DIRECTION ( 'NONE',  ( -1.000000000000000000, 0.000000000000000000, 0.000000000000000000 ) ) ;
#29151=AXIS2_PLACEMENT_3D ( 'NONE', #41802, #46019, #10010 ) ;
#29153=LINE ( 'NONE', #36791, #1864 ) ;
#29155=CARTESIAN_POINT ( 'NONE',  ( -339.1964088526558498, -64.99044476834248485, -7.608018572113150135 ) ) ;
#29156=ADVANCED_FACE ( 'NONE', ( #34875 ), #26745, .T. ) ;
#29164=ORIENTED_EDGE ( 'NONE', *, *, #24352, .F. ) ;
#29171=VECTOR ( 'NONE', #48538, 1000.000000000000000 ) ;
#29174=VECTOR ( 'NONE', #32850, 1000.000000000000000 ) ;
#29177=PLANE ( 'NONE',  #46823 ) ;
#29178=DIRECTION ( 'NONE',  ( 1.000000000000000000, -0.000000000000000000, -0.000000000000000000 ) ) ;
#29180=FACE_OUTER_BOUND ( 'NONE', #51226, .T. ) ;
#29181=ORIENTED_EDGE ( 'NONE', *, *, #26313, .F. ) ;
#29185=PLANE ( 'NONE',  #37588 ) ;
#29186=LINE ( 'NONE', #45241, #51811 ) ;
#29187=DIRECTION ( 'NONE',  ( 0.000000000000000000, 0.000000000000000000, -1.000000000000000000 ) ) ;
#29196=EDGE_LOOP ( 'NONE', ( #9431, #276, #7457, #5342 ) ) ;
#29199=CARTESIAN_POINT ( 'NONE',  ( -332.3517673607765914, -127.9985676343858501, 58.88711093124869222 ) ) ;
#29202=ORIENTED_EDGE ( 'NONE', *, *, #44218, .F. ) ;
#29208=VECTOR ( 'NONE', #6040, 1000.000000000000000 ) ;
#29212=CARTESIAN_POINT ( 'NONE',  ( -305.0000000000000568, -178.6135371030394481, 23.71704087764532076 ) ) ;
#29214=EDGE_CURVE ( 'NONE', #48223, #42957, #31457, .T. ) ;
#29215=ADVANCED_FACE ( 'NONE', ( #39077 ), #38313, .F. ) ;
#29217=CARTESIAN_POINT ( 'NONE',  ( -339.1964088526558498, -66.33409060400673241, -14.60509510167901404 ) ) ;
#29219=CARTESIAN_POINT ( 'NONE',  ( -332.3517673607765914, -135.0638248728647852, 57.91551518289418254 ) ) ;
#29222=EDGE_LOOP ( 'NONE', ( #13975, #46028, #16282, #19569 ) ) ;
#29231=EDGE_CURVE ( 'NONE', #8999, #48057, #2577, .T. ) ;
#29232=AXIS2_PLACEMENT_3D ( 'NONE', #46319, #14776, #23171 ) ;
#29233=ORIENTED_EDGE ( 'NONE', *, *, #23469, .F. ) ;
#29235=VECTOR ( 'NONE', #42866, 1000.000000000000000 ) ;
#29242=CARTESIAN_POINT ( 'NONE',  ( -365.0000000000001137, -78.50000000000002842, 0.000000000000000000 ) ) ;
#29243=VERTEX_POINT ( 'NONE', #28025 ) ;
#29249=LINE ( 'NONE', #9288, #34061 ) ;
#29251=CIRCLE ( 'NONE', #19161, 60.00000000000000000 ) ;
#29252=ORIENTED_EDGE ( 'NONE', *, *, #47746, .F. ) ;
#29254=CARTESIAN_POINT ( 'NONE',  ( -339.1964088526558498, -103.0458197858333165, -55.34326076196084188 ) ) ;
#29256=ORIENTED_EDGE ( 'NONE', *, *, #13391, .F. ) ;
#29257=DIRECTION ( 'NONE',  ( 0.000000000000000000, -0.9927088740980530845, 0.1205366802553303057 ) ) ;
#29259=ORIENTED_EDGE ( 'NONE', *, *, #9969, .F. ) ;
#29260=FACE_BOUND ( 'NONE', #40196, .T. ) ;
#29262=EDGE_LOOP ( 'NONE', ( #42429, #4946, #9273, #14836 ) ) ;
#29265=PRODUCT_DEFINITION_FORMATION_WITH_SPECIFIED_SOURCE ( 'ANY', '', #41948, .NOT_KNOWN. ) ;
#29267=CARTESIAN_POINT ( 'NONE',  ( -330.4913330509368166, -150.4759391377560576, -52.47426709956116042 ) ) ;
#29269=LINE ( 'NONE', #1140, #41279 ) ;
#29272=CARTESIAN_POINT ( 'NONE',  ( -330.4913330509368166, -64.86990808808705822, 6.615309698014281814 ) ) ;
#29275=EDGE_CURVE ( 'NONE', #47980, #12857, #25527, .T. ) ;
#29278=ORIENTED_EDGE ( 'NONE', *, *, #39450, .T. ) ;
#29282=AXIS2_PLACEMENT_3D ( 'NONE', #32786, #16780, #52004 ) ;
#29286=ORIENTED_EDGE ( 'NONE', *, *, #36352, .F. ) ;
#29289=CARTESIAN_POINT ( 'NONE',  ( -339.1964088526558498, -122.9999999999993747, 59.00000000000002132 ) ) ;
#29300=VERTEX_POINT ( 'NONE', #35927 ) ;
#29302=ORIENTED_EDGE ( 'NONE', *, *, #42577, .F. ) ;
#29303=FACE_OUTER_BOUND ( 'NONE', #18857, .T. ) ;
#29305=VECTOR ( 'NONE', #3366, 1000.000000000000000 ) ;
#29308=ORIENTED_EDGE ( 'NONE', *, *, #44672, .F. ) ;
#29309=AXIS2_PLACEMENT_3D ( 'NONE', #47740, #46966, #146 ) ;
#29311=DIRECTION ( 'NONE',  ( 0.000000000000000000, -0.9709418174260502354, 0.2393156642875652051 ) ) ;
#29312=ORIENTED_EDGE ( 'NONE', *, *, #26296, .T. ) ;
#29316=CARTESIAN_POINT ( 'NONE',  ( -336.3521761649654422, -128.9912765084839066, 58.76657425099337928 ) ) ;
#29325=LINE ( 'NONE', #45119, #50596 ) ;
#29335=LINE ( 'NONE', #17781, #48379 ) ;
#29343=DIRECTION ( 'NONE',  ( 0.000000000000000000, 0.000000000000000000, 1.000000000000000000 ) ) ;
#29345=CARTESIAN_POINT ( 'NONE',  ( -339.1964088526558498, -123.5000000000000284, 0.000000000000000000 ) ) ;
#29346=PLANE ( 'NONE',  #3289 ) ;
#29347=DIRECTION ( 'NONE',  ( 0.000000000000000000, -0.5680647467311596976, -0.8229838658936536877 ) ) ;
#29348=VERTEX_POINT ( 'NONE', #20405 ) ;
#29350=DIRECTION ( 'NONE',  ( 0.000000000000000000, 0.000000000000000000, 1.000000000000000000 ) ) ;
#29351=ORIENTED_EDGE ( 'NONE', *, *, #44543, .T. ) ;
#29354=AXIS2_PLACEMENT_3D ( 'NONE', #31083, #43171, #30563 ) ;
#29364=CARTESIAN_POINT ( 'NONE',  ( -305.0000000000000568, -69.63373947859463442, 26.42775013958025454 ) ) ;
#29365=ORIENTED_EDGE ( 'NONE', *, *, #43632, .T. ) ;
#29371=ORIENTED_EDGE ( 'NONE', *, *, #5757, .F. ) ;
#29378=DIRECTION ( 'NONE',  ( -0.000000000000000000, 0.9927088740980538617, -0.1205366802553232974 ) ) ;
#29379=VERTEX_POINT ( 'NONE', #31973 ) ;
#29382=DIRECTION ( 'NONE',  ( -0.000000000000000000, -0.9927088740980530845, 0.1205366802553303057 ) ) ;
#29384=DIRECTION ( 'NONE',  ( -0.000000000000000000, 0.1205366802553095168, -0.9927088740980556381 ) ) ;
#29386=EDGE_LOOP ( 'NONE', ( #17315, #38551, #27716, #50649 ) ) ;
#29389=DIRECTION ( 'NONE',  ( 0.000000000000000000, 0.7485107481711024136, 0.6631226582407937498 ) ) ;
#29396=VECTOR ( 'NONE', #37870, 1000.000000000000000 ) ;
#29397=LINE ( 'NONE', #42001, #13989 ) ;
#29398=EDGE_LOOP ( 'NONE', ( #27539, #47957, #9061, #35822 ) ) ;
#29400=EDGE_CURVE ( 'NONE', #51691, #6345, #51531, .T. ) ;
#29404=ORIENTED_EDGE ( 'NONE', *, *, #41009, .F. ) ;
#29410=CARTESIAN_POINT ( 'NONE',  ( -305.0000000000000568, -102.6919536717973926, 56.27632902032055284 ) ) ;
#29428=CARTESIAN_POINT ( 'NONE',  ( -305.0000000000000568, -171.9335100611925213, 35.41461708323791413 ) ) ;
#29430=CARTESIAN_POINT ( 'NONE',  ( -339.1964088526558498, -64.50000000000000000, -0.5000000000000457412 ) ) ;
#29431=VERTEX_POINT ( 'NONE', #44848 ) ;
#29433=VERTEX_POINT ( 'NONE', #1206 ) ;
#29434=EDGE_CURVE ( 'NONE', #13843, #21465, #45126, .T. ) ;
#29439=DIRECTION ( 'NONE',  ( 1.000000000000000000, -5.781354811211787559E-17, 6.525800561035047192E-17 ) ) ;
#29440=ORIENTED_EDGE ( 'NONE', *, *, #4843, .F. ) ;
#29441=ORIENTED_EDGE ( 'NONE', *, *, #10578, .F. ) ;
#29442=DIRECTION ( 'NONE',  ( -0.000000000000000000, -0.8854560256532126861, -0.4647231720437631775 ) ) ;
#29445=VECTOR ( 'NONE', #40586, 1000.000000000000000 ) ;
#29449=CARTESIAN_POINT ( 'NONE',  ( -339.1964088526558498, -150.4759391377552618, 52.47426709956155122 ) ) ;
#29453=DIRECTION ( 'NONE',  ( 1.000000000000000000, -0.000000000000000000, -0.000000000000000000 ) ) ;
#29462=EDGE_CURVE ( 'NONE', #30840, #32017, #9891, .T. ) ;
#29463=CARTESIAN_POINT ( 'NONE',  ( -339.1964088526558498, -138.1050951016783301, 57.16590939599346655 ) ) ;
#29467=CARTESIAN_POINT ( 'NONE',  ( -305.0000000000000568, -123.5000000000000284, -20.00000000000000355 ) ) ;
#29468=CARTESIAN_POINT ( 'NONE',  ( -305.0000000000000568, -145.2430625708873322, -55.92172413327827485 ) ) ;
#29470=ORIENTED_EDGE ( 'NONE', *, *, #18593, .T. ) ;
#29473=ADVANCED_FACE ( 'NONE', ( #37478 ), #37737, .F. ) ;
#29479=ORIENTED_EDGE ( 'NONE', *, *, #45659, .T. ) ;
#29485=CARTESIAN_POINT ( 'NONE',  ( -330.4913330509368166, -167.9936954712156023, -38.74998146212117689 ) ) ;
#29490=CARTESIAN_POINT ( 'NONE',  ( -332.3517673607765914, -173.7880015656344312, -32.72792230702632565 ) ) ;
#29491=VECTOR ( 'NONE', #23782, 1000.000000000000000 ) ;
#29495=EDGE_CURVE ( 'NONE', #37735, #11736, #13563, .T. ) ;
#29500=CARTESIAN_POINT ( 'NONE',  ( -336.3521761649654422, -118.8878589706978772, -59.82247199109903590 ) ) ;
#29505=CARTESIAN_POINT ( 'NONE',  ( -339.1964088526558498, -151.3613951634092700, -52.00954392751739164 ) ) ;
#29509=CARTESIAN_POINT ( 'NONE',  ( -330.4913330509368166, -109.6270296344155923, 58.37414404713457117 ) ) ;
#29514=CARTESIAN_POINT ( 'NONE',  ( -330.4913330509368166, -162.9984922102920848, 43.83057281297495678 ) ) ;
#29519=DIRECTION ( 'NONE',  ( 0.000000000000000000, -1.191176786837407622E-13, -1.000000000000000000 ) ) ;
#29521=DIRECTION ( 'NONE',  ( -0.000000000000000000, -0.6631226582407885317, 0.7485107481711069655 ) ) ;
#29524=DIRECTION ( 'NONE',  ( 1.000000000000000000, -0.000000000000000000, -0.000000000000000000 ) ) ;
#29527=DIRECTION ( 'NONE',  ( -1.000000000000000000, 0.000000000000000000, -0.000000000000000000 ) ) ;
#29535=ORIENTED_EDGE ( 'NONE', *, *, #13002, .F. ) ;
#29537=ORIENTED_EDGE ( 'NONE', *, *, #32495, .F. ) ;
#29538=CARTESIAN_POINT ( 'NONE',  ( -332.3517673607765914, -148.5878911270064009, 53.46519113769075204 ) ) ;
#29541=VECTOR ( 'NONE', #37817, 1000.000000000000114 ) ;
#29542=EDGE_CURVE ( 'NONE', #8048, #9084, #36432, .T. ) ;
#29544=EDGE_LOOP ( 'NONE', ( #48701, #7869, #21701, #13825 ) ) ;
#29547=CARTESIAN_POINT ( 'NONE',  ( -332.3517673607765914, -119.0014323656137947, -58.88711093124865670 ) ) ;
#29552=CIRCLE ( 'NONE', #6865, 60.00000000000000000 ) ;
#29554=ORIENTED_EDGE ( 'NONE', *, *, #857, .F. ) ;
#29555=PLANE ( 'NONE',  #40863 ) ;
#29557=CIRCLE ( 'NONE', #32063, 60.00000000000000000 ) ;
#29562=EDGE_CURVE ( 'NONE', #30970, #43162, #46937, .T. ) ;
#29565=ADVANCED_FACE ( 'NONE', ( #38516 ), #2514, .F. ) ;
#29567=CARTESIAN_POINT ( 'NONE',  ( -339.1964088526558498, -180.9052250602807703, 13.63415328425337236 ) ) ;
#29570=CARTESIAN_POINT ( 'NONE',  ( -336.3521761649654422, -87.81784868886214213, 47.06073758877343494 ) ) ;
#29571=DIRECTION ( 'NONE',  ( 1.000000000000000000, -0.000000000000000000, 0.000000000000000000 ) ) ;
#29578=VECTOR ( 'NONE', #11578, 1000.000000000000000 ) ;
#29579=EDGE_LOOP ( 'NONE', ( #16683, #46825, #45632, #46053 ) ) ;
#29580=DIRECTION ( 'NONE',  ( 1.000000000000000000, -0.000000000000000000, -0.000000000000000000 ) ) ;
#29585=DIRECTION ( 'NONE',  ( -0.000000000000000000, 0.3546048870425463906, 0.9350162426854107256 ) ) ;
#29597=ORIENTED_EDGE ( 'NONE', *, *, #43632, .F. ) ;
#29602=DIRECTION ( 'NONE',  ( 0.000000000000000000, 0.000000000000000000, -1.000000000000000000 ) ) ;
#29605=ORIENTED_EDGE ( 'NONE', *, *, #42175, .F. ) ;
#29608=ORIENTED_EDGE ( 'NONE', *, *, #18134, .F. ) ;
#29611=EDGE_LOOP ( 'NONE', ( #51410, #32223, #39278, #10441 ) ) ;
#29621=AXIS2_PLACEMENT_3D ( 'NONE', #1498, #36980, #49854 ) ;
#29622=FACE_OUTER_BOUND ( 'NONE', #43330, .T. ) ;
#29626=VERTEX_POINT ( 'NONE', #3293 ) ;
#29630=LINE ( 'NONE', #31, #40033 ) ;
#29632=ORIENTED_EDGE ( 'NONE', *, *, #50577, .F. ) ;
#29633=CARTESIAN_POINT ( 'NONE',  ( -339.1964088526558498, -157.9941932480470541, -49.09328500076547641 ) ) ;
#29643=DIRECTION ( 'NONE',  ( 0.000000000000000000, 0.000000000000000000, 1.000000000000000000 ) ) ;
#29648=LINE ( 'NONE', #28864, #36459 ) ;
#29662=VERTEX_POINT ( 'NONE', #15643 ) ;
#29668=ADVANCED_FACE ( 'NONE', ( #11933 ), #8002, .F. ) ;
#29672=CARTESIAN_POINT ( 'NONE',  ( -332.3517673607765914, -76.43926241122620979, -35.68215131113738181 ) ) ;
#29673=DIRECTION ( 'NONE',  ( 0.000000000000000000, 0.9927088740980556381, 0.1205366802553095307 ) ) ;
#29674=ORIENTED_EDGE ( 'NONE', *, *, #16274, .F. ) ;
#29676=ADVANCED_FACE ( 'NONE', ( #11418 ), #47708, .F. ) ;
#29677=ORIENTED_EDGE ( 'NONE', *, *, #26302, .T. ) ;
#29678=CARTESIAN_POINT ( 'NONE',  ( -332.3517673607765914, -181.4155151828941825, -11.56382487286496463 ) ) ;
#29681=CIRCLE ( 'NONE', #1999, 5.000000000000001776 ) ;
#29685=VECTOR ( 'NONE', #17334, 1000.000000000000000 ) ;
#29686=DIRECTION ( 'NONE',  ( 0.000000000000000000, 0.2393156642875582940, 0.9709418174260519008 ) ) ;
#29687=CARTESIAN_POINT ( 'NONE',  ( -339.1964088526558498, -162.2499814621209850, 44.49369547121574442 ) ) ;
#29688=ORIENTED_EDGE ( 'NONE', *, *, #5565, .T. ) ;
#29689=CARTESIAN_POINT ( 'NONE',  ( -330.4913330509368166, -65.12585595286530804, -13.87297036558381080 ) ) ;
#29693=DIRECTION ( 'NONE',  ( -0.000000000000000000, 1.000000000000000000, -0.000000000000000000 ) ) ;
#29697=CARTESIAN_POINT ( 'NONE',  ( -330.4913330509368166, -73.83865025250327108, -33.67120938215323633 ) ) ;
#29698=DIRECTION ( 'NONE',  ( 1.000000000000000000, -3.091579882402533631E-17, 8.151826190875940963E-17 ) ) ;
#29699=PLANE ( 'NONE',  #28173 ) ;
#29706=ORIENTED_EDGE ( 'NONE', *, *, #22028, .T. ) ;
#29709=CARTESIAN_POINT ( 'NONE',  ( -330.4913330509368166, -74.40671499923389831, 34.49419324804615172 ) ) ;
#29716=ORIENTED_EDGE ( 'NONE', *, *, #22387, .F. ) ;
#29717=CARTESIAN_POINT ( 'NONE',  ( -336.3521761649654422, -72.67320051506121104, 31.88473700876054551 ) ) ;
#29718=DIRECTION ( 'NONE',  ( 1.000000000000000000, -2.086444717177429095E-17, 8.465038975556428342E-17 ) ) ;
#29720=AXIS2_PLACEMENT_3D ( 'NONE', #16809, #9683, #29643 ) ;
#29722=LINE ( 'NONE', #49472, #35828 ) ;
#29724=PLANE ( 'NONE',  #24603 ) ;
#29727=CARTESIAN_POINT ( 'NONE',  ( -339.1964088526558498, -95.63860483659040312, 52.00954392751717847 ) ) ;
#29737=ORIENTED_EDGE ( 'NONE', *, *, #19856, .T. ) ;
#29738=ORIENTED_EDGE ( 'NONE', *, *, #14812, .T. ) ;
#29739=CARTESIAN_POINT ( 'NONE',  ( -365.0000000000001137, -168.5000000000000284, 0.000000000000000000 ) ) ;
#29741=CARTESIAN_POINT ( 'NONE',  ( -336.3521761649653854, -121.8677111499054320, 59.97779283292990016 ) ) ;
#29748=ADVANCED_FACE ( 'NONE', ( #24547 ), #16158, .F. ) ;
#29751=EDGE_LOOP ( 'NONE', ( #27094, #19126, #29259, #14340 ) ) ;
#29752=DIRECTION ( 'NONE',  ( -1.000000000000000000, -0.000000000000000000, -0.000000000000000000 ) ) ;
#29753=ADVANCED_FACE ( 'NONE', ( #12194 ), #28227, .F. ) ;
#29758=CARTESIAN_POINT ( 'NONE',  ( -339.1964088526558498, -102.1108035431478811, -54.98865587491830809 ) ) ;
#29767=DIRECTION ( 'NONE',  ( 1.000000000000000000, 4.051632851310648003E-17, -7.719741424018512503E-17 ) ) ;
#29772=VERTEX_POINT ( 'NONE', #365 ) ;
#29779=PLANE ( 'NONE',  #39166 ) ;
#29786=DIRECTION ( 'NONE',  ( 1.043714542225393381E-14, -0.8229838658936536877, 0.5680647467311596976 ) ) ;
#29787=DIRECTION ( 'NONE',  ( -0.000000000000000000, 0.5680647467311540355, -0.8229838658936575735 ) ) ;
#29788=ORIENTED_EDGE ( 'NONE', *, *, #37215, .T. ) ;
#29790=VECTOR ( 'NONE', #4379, 1000.000000000000000 ) ;
#29793=EDGE_CURVE ( 'NONE', #24508, #1071, #13252, .T. ) ;
#29796=EDGE_CURVE ( 'NONE', #23872, #16769, #28892, .T. ) ;
#29800=EDGE_CURVE ( 'NONE', #28470, #39299, #44790, .T. ) ;
#29801=AXIS2_PLACEMENT_3D ( 'NONE', #17306, #5219, #33051 ) ;
#29805=CIRCLE ( 'NONE', #15561, 60.00000000000000000 ) ;
#29821=EDGE_CURVE ( 'NONE', #31094, #10455, #17471, .T. ) ;
#29824=CARTESIAN_POINT ( 'NONE',  ( -332.3517673607765914, -97.07224986041923387, -53.86626052140510978 ) ) ;
#29826=ORIENTED_EDGE ( 'NONE', *, *, #38181, .T. ) ;
#29827=VECTOR ( 'NONE', #18222, 1000.000000000000000 ) ;
#29828=LINE ( 'NONE', #32987, #9062 ) ;
#29829=LINE ( 'NONE', #5938, #32543 ) ;
#29833=DIRECTION ( 'NONE',  ( 0.000000000000000000, -0.7485107481710977506, 0.6631226582407989678 ) ) ;
#29836=ORIENTED_EDGE ( 'NONE', *, *, #8922, .F. ) ;
#29838=VERTEX_POINT ( 'NONE', #20605 ) ;
#29843=AXIS2_PLACEMENT_3D ( 'NONE', #1578, #32842, #48896 ) ;
#29851=CARTESIAN_POINT ( 'NONE',  ( -305.0000000000000568, -133.3383340306578759, -59.18789727217212970 ) ) ;
#29857=VERTEX_POINT ( 'NONE', #49260 ) ;
#29859=DIRECTION ( 'NONE',  ( -1.000000000000000000, -0.000000000000000000, -0.000000000000000000 ) ) ;
#29866=DIRECTION ( 'NONE',  ( -0.000000000000000000, -0.1205366802553268363, -0.9927088740980534176 ) ) ;
#29868=AXIS2_PLACEMENT_3D ( 'NONE', #9489, #48920, #5556 ) ;
#29871=DIRECTION ( 'NONE',  ( -0.000000000000000000, 0.8229838658936634577, 0.5680647467311457088 ) ) ;
#29872=VERTEX_POINT ( 'NONE', #19003 ) ;
#29876=DIRECTION ( 'NONE',  ( 1.000000000000000000, -0.000000000000000000, -0.000000000000000000 ) ) ;
#29882=CARTESIAN_POINT ( 'NONE',  ( -339.1964088526558498, -96.52406086224361559, 52.47426709956096147 ) ) ;
#29884=ADVANCED_FACE ( 'NONE', ( #47122 ), #2964, .F. ) ;
#29886=VECTOR ( 'NONE', #34292, 999.9999999999998863 ) ;
#29893=LINE ( 'NONE', #26729, #44259 ) ;
#29901=ORIENTED_EDGE ( 'NONE', *, *, #13985, .F. ) ;
#29903=AXIS2_PLACEMENT_3D ( 'NONE', #2767, #46411, #18034 ) ;
#29904=CARTESIAN_POINT ( 'NONE',  ( -336.3521761649654422, -91.61526299123897843, -50.82679948493848343 ) ) ;
#29908=ORIENTED_EDGE ( 'NONE', *, *, #5028, .F. ) ;
#29910=DIRECTION ( 'NONE',  ( 0.000000000000000000, 0.3546048870425396182, 0.9350162426854132791 ) ) ;
#29914=FACE_OUTER_BOUND ( 'NONE', #32302, .T. ) ;
#29918=FACE_OUTER_BOUND ( 'NONE', #8361, .T. ) ;
#29919=ORIENTED_EDGE ( 'NONE', *, *, #16077, .F. ) ;
#29921=CIRCLE ( 'NONE', #14821, 60.00000000000000000 ) ;
#29923=AXIS2_PLACEMENT_3D ( 'NONE', #17842, #13899, #13382 ) ;
#29929=EDGE_CURVE ( 'NONE', #33549, #18186, #23055, .T. ) ;
#29936=CARTESIAN_POINT ( 'NONE',  ( -336.3521761649654422, -145.9479049231020440, -54.58714071513102795 ) ) ;
#29943=VECTOR ( 'NONE', #37413, 1000.000000000000000 ) ;
#29949=ADVANCED_FACE ( 'NONE', ( #33986 ), #26100, .F. ) ;
#29951=LINE ( 'NONE', #42034, #48282 ) ;
#29959=LINE ( 'NONE', #9476, #46635 ) ;
#29960=VECTOR ( 'NONE', #14283, 1000.000000000000000 ) ;
#29963=EDGE_LOOP ( 'NONE', ( #9620, #18362, #13781, #28406 ) ) ;
#29964=EDGE_CURVE ( 'NONE', #41179, #38255, #22435, .T. ) ;
#29966=CARTESIAN_POINT ( 'NONE',  ( -336.3521761649653854, -175.8491356171901145, 29.31839013542587935 ) ) ;
#29969=ORIENTED_EDGE ( 'NONE', *, *, #1149, .T. ) ;
#29970=ORIENTED_EDGE ( 'NONE', *, *, #25944, .F. ) ;
#29974=PLANE ( 'NONE',  #44664 ) ;
#29975=DIRECTION ( 'NONE',  ( 0.000000000000000000, 0.3546048870425463906, 0.9350162426854107256 ) ) ;
#29977=PLANE ( 'NONE',  #45975 ) ;
#29983=CARTESIAN_POINT ( 'NONE',  ( -305.0000000000000568, -163.6602333390095509, 44.57752413668021774 ) ) ;
#29985=EDGE_CURVE ( 'NONE', #21253, #17026, #46354, .T. ) ;
#29987=ORIENTED_EDGE ( 'NONE', *, *, #286, .T. ) ;
#29989=VECTOR ( 'NONE', #1354, 1000.000000000000114 ) ;
#29996=EDGE_CURVE ( 'NONE', #49741, #14193, #26870, .T. ) ;
#29999=ADVANCED_FACE ( 'NONE', ( #30305 ), #38954, .F. ) ;
#30000=AXIS2_PLACEMENT_3D ( 'NONE', #51049, #15040, #3699 ) ;
#30005=ORIENTED_EDGE ( 'NONE', *, *, #5701, .F. ) ;
#30006=VECTOR ( 'NONE', #36769, 1000.000000000000000 ) ;
#30008=DIRECTION ( 'NONE',  ( 0.000000000000000000, -0.6631226582407863113, 0.7485107481711089639 ) ) ;
#30011=ORIENTED_EDGE ( 'NONE', *, *, #21388, .T. ) ;
#30012=EDGE_LOOP ( 'NONE', ( #28218, #14556, #23718, #22755 ) ) ;
#30025=ORIENTED_EDGE ( 'NONE', *, *, #15598, .T. ) ;
#30026=DIRECTION ( 'NONE',  ( 0.000000000000000000, 0.000000000000000000, 1.000000000000000000 ) ) ;
#30028=ORIENTED_EDGE ( 'NONE', *, *, #26972, .F. ) ;
#30029=LINE ( 'NONE', #25557, #45924 ) ;
#30030=DIRECTION ( 'NONE',  ( -0.000000000000000000, -0.8854560256532126861, -0.4647231720437631775 ) ) ;
#30036=CARTESIAN_POINT ( 'NONE',  ( -336.3521761649654422, -67.40061919120938683, 18.46045550523129819 ) ) ;
#30037=ORIENTED_EDGE ( 'NONE', *, *, #25103, .F. ) ;
#30039=EDGE_CURVE ( 'NONE', #19848, #51884, #14551, .T. ) ;
#30041=CARTESIAN_POINT ( 'NONE',  ( -336.3521761649654422, -78.25545813661345562, 37.90245108779119931 ) ) ;
#30053=DIRECTION ( 'NONE',  ( 0.000000000000000000, 0.3546048870425396182, 0.9350162426854132791 ) ) ;
#30060=CIRCLE ( 'NONE', #41808, 60.00000000000000000 ) ;
#30062=VECTOR ( 'NONE', #27863, 1000.000000000000000 ) ;
#30069=FACE_OUTER_BOUND ( 'NONE', #18569, .T. ) ;
#30071=ORIENTED_EDGE ( 'NONE', *, *, #14983, .F. ) ;
#30074=LINE ( 'NONE', #30851, #46002 ) ;
#30076=CARTESIAN_POINT ( 'NONE',  ( -336.3521761649654422, -148.5878911270064009, 53.46519113769075204 ) ) ;
#30079=VERTEX_POINT ( 'NONE', #11630 ) ;
#30085=ORIENTED_EDGE ( 'NONE', *, *, #39317, .T. ) ;
#30086=VERTEX_POINT ( 'NONE', #39982 ) ;
#30093=AXIS2_PLACEMENT_3D ( 'NONE', #4170, #7583, #19931 ) ;
#30094=CARTESIAN_POINT ( 'NONE',  ( -330.4913330509368166, -157.4273119900852578, -48.27201571436002325 ) ) ;
#30097=CARTESIAN_POINT ( 'NONE',  ( -339.1964088526558498, -168.7406467949209059, -39.41172259083857909 ) ) ;
#30100=DIRECTION ( 'NONE',  ( -1.000000000000000000, 0.000000000000000000, 0.000000000000000000 ) ) ;
#30116=FACE_OUTER_BOUND ( 'NONE', #31189, .T. ) ;
#30117=EDGE_CURVE ( 'NONE', #13092, #47587, #47896, .T. ) ;
#30120=ORIENTED_EDGE ( 'NONE', *, *, #22749, .F. ) ;
#30123=VERTEX_POINT ( 'NONE', #11871 ) ;
#30128=CARTESIAN_POINT ( 'NONE',  ( -330.4913330509368166, -78.25935320507949200, -39.41172259083896279 ) ) ;
#30130=CARTESIAN_POINT ( 'NONE',  ( -339.1964088526558498, -123.5000000000000284, 0.000000000000000000 ) ) ;
#30131=CARTESIAN_POINT ( 'NONE',  ( -339.1964088526558498, -157.1712093821534211, -49.66134974749665076 ) ) ;
#30134=VECTOR ( 'NONE', #21882, 1000.000000000000000 ) ;
#30140=ORIENTED_EDGE ( 'NONE', *, *, #22506, .F. ) ;
#30143=CARTESIAN_POINT ( 'NONE',  ( -336.3521761649654422, -154.8494888031386836, 50.05135858667791382 ) ) ;
#30145=LINE ( 'NONE', #1766, #6869 ) ;
#30146=CARTESIAN_POINT ( 'NONE',  ( -330.4913330509368166, -180.9052250602809693, -13.63415328425256945 ) ) ;
#30152=CARTESIAN_POINT ( 'NONE',  ( -330.4913330509368166, -138.1050951016791544, -57.16590939599326049 ) ) ;
#30158=VERTEX_POINT ( 'NONE', #28157 ) ;
#30167=VERTEX_POINT ( 'NONE', #12914 ) ;
#30168=EDGE_CURVE ( 'NONE', #17256, #14634, #10477, .T. ) ;
#30171=DIRECTION ( 'NONE',  ( 0.000000000000000000, -1.000000000000000000, 1.047444401652940007E-14 ) ) ;
#30177=EDGE_LOOP ( 'NONE', ( #39884, #28103, #29164, #45208 ) ) ;
#30180=LINE ( 'NONE', #22562, #2113 ) ;
#30183=CARTESIAN_POINT ( 'NONE',  ( -332.3517673607765914, -171.3361784870343740, 36.21739951675979086 ) ) ;
#30187=DIRECTION ( 'NONE',  ( 0.000000000000000000, 0.000000000000000000, -1.000000000000000000 ) ) ;
#30189=CARTESIAN_POINT ( 'NONE',  ( -330.4913330509368166, -71.02573290043841325, 26.97593913775512320 ) ) ;
#30201=DIRECTION ( 'NONE',  ( 1.000000000000000000, 0.000000000000000000, 0.000000000000000000 ) ) ;
#30205=ORIENTED_EDGE ( 'NONE', *, *, #45781, .T. ) ;
#30211=ORIENTED_EDGE ( 'NONE', *, *, #21136, .F. ) ;
#30213=DIRECTION ( 'NONE',  ( 0.000000000000000000, 0.7485107481710953081, -0.6631226582408016323 ) ) ;
#30215=DIRECTION ( 'NONE',  ( 1.000000000000000000, 0.000000000000000000, 0.000000000000000000 ) ) ;
#30218=CARTESIAN_POINT ( 'NONE',  ( -336.3521761649654422, -170.5607375887735770, 35.68215131113770155 ) ) ;
#30219=VERTEX_POINT ( 'NONE', #34129 ) ;
#30220=CARTESIAN_POINT ( 'NONE',  ( -332.3517673607765914, -173.5513585866778214, -31.34948880313881503 ) ) ;
#30221=EDGE_LOOP ( 'NONE', ( #27674, #41960, #19482, #51172 ) ) ;
#30224=ADVANCED_FACE ( 'NONE', ( #28938 ), #40505, .F. ) ;
#30226=CARTESIAN_POINT ( 'NONE',  ( -336.3521761649654422, -123.5000000000000284, 0.000000000000000000 ) ) ;
#30227=DIRECTION ( 'NONE',  ( 0.000000000000000000, 0.000000000000000000, 1.000000000000000000 ) ) ;
#30230=EDGE_LOOP ( 'NONE', ( #37329, #16120, #29371, #49137 ) ) ;
#30235=CARTESIAN_POINT ( 'NONE',  ( -332.3517673607765914, -68.91285928486892942, -22.44790492310182017 ) ) ;
#30238=LINE ( 'NONE', #46792, #38121 ) ;
#30240=LINE ( 'NONE', #50481, #9821 ) ;
#30241=DIRECTION ( 'NONE',  ( 0.000000000000000000, -0.7485107481710999711, 0.6631226582407964143 ) ) ;
#30248=VECTOR ( 'NONE', #5968, 1000.000000000000000 ) ;
#30249=DIRECTION ( 'NONE',  ( 0.000000000000000000, 0.000000000000000000, -1.000000000000000000 ) ) ;
#30250=LINE ( 'NONE', #34192, #10146 ) ;
#30259=VERTEX_POINT ( 'NONE', #2588 ) ;
#30260=CARTESIAN_POINT ( 'NONE',  ( -336.3521761649654422, -80.42027357919624819, -40.34602258462219027 ) ) ;
#30262=AXIS2_PLACEMENT_3D ( 'NONE', #9505, #32366, #48678 ) ;
#30266=VERTEX_POINT ( 'NONE', #14952 ) ;
#30268=PLANE ( 'NONE',  #6598 ) ;
#30269=FACE_OUTER_BOUND ( 'NONE', #43284, .T. ) ;
#30272=CARTESIAN_POINT ( 'NONE',  ( -336.3521761649654422, -123.5000000000000284, 0.000000000000000000 ) ) ;
#30276=VERTEX_POINT ( 'NONE', #34633 ) ;
#30285=DIRECTION ( 'NONE',  ( 0.000000000000000000, -0.9927088740980535286, 0.1205366802553268502 ) ) ;
#30288=CARTESIAN_POINT ( 'NONE',  ( -339.1964088526558498, -74.40671499923440990, -34.49419324804689779 ) ) ;
#30293=ORIENTED_EDGE ( 'NONE', *, *, #7208, .T. ) ;
#30294=CARTESIAN_POINT ( 'NONE',  ( -340.0000000000000568, -78.50000000000002842, 0.000000000000000000 ) ) ;
#30298=LINE ( 'NONE', #50291, #29960 ) ;
#30302=EDGE_CURVE ( 'NONE', #14589, #1636, #46743, .T. ) ;
#30304=DIRECTION ( 'NONE',  ( 1.000000000000000000, -0.000000000000000000, -0.000000000000000000 ) ) ;
#30305=FACE_OUTER_BOUND ( 'NONE', #51971, .T. ) ;
#30312=DIRECTION ( 'NONE',  ( 0.000000000000000000, 5.319818659662208160E-15, -1.000000000000000000 ) ) ;
#30313=CARTESIAN_POINT ( 'NONE',  ( -332.3517673607765914, -63.52220716707010695, -1.632288850093980725 ) ) ;
#30316=CARTESIAN_POINT ( 'NONE',  ( -339.1964088526558498, -64.86990808808704401, 6.615309698014191220 ) ) ;
#30320=VERTEX_POINT ( 'NONE', #50949 ) ;
#30323=AXIS2_PLACEMENT_3D ( 'NONE', #44008, #40055, #48222 ) ;
#30325=EDGE_CURVE ( 'NONE', #40382, #14358, #38835, .T. ) ;
#30329=CIRCLE ( 'NONE', #7676, 60.00000000000000000 ) ;
#30330=ORIENTED_EDGE ( 'NONE', *, *, #27458, .T. ) ;
#30332=CARTESIAN_POINT ( 'NONE',  ( -330.4913330509368166, -64.99044476834247064, -7.608018572113060429 ) ) ;
#30335=LINE ( 'NONE', #34027, #20502 ) ;
#30338=PLANE ( 'NONE',  #6386 ) ;
#30339=AXIS2_PLACEMENT_3D ( 'NONE', #20226, #43876, #51786 ) ;
#30342=EDGE_LOOP ( 'NONE', ( #23222, #49544, #33460, #36661 ) ) ;
#30345=VECTOR ( 'NONE', #14639, 1000.000000000000000 ) ;
#30354=DIRECTION ( 'NONE',  ( -0.000000000000000000, 0.7485107481711089639, 0.6631226582407863113 ) ) ;
#30357=ORIENTED_EDGE ( 'NONE', *, *, #18425, .T. ) ;
#30362=VECTOR ( 'NONE', #12524, 999.9999999999998863 ) ;
#30370=AXIS2_PLACEMENT_3D ( 'NONE', #32641, #36317, #24758 ) ;
#30371=CARTESIAN_POINT ( 'NONE',  ( -170.0000000000000284, -123.5000000000000284, 15.24495751795539000 ) ) ;
#30372=VECTOR ( 'NONE', #22125, 1000.000000000000000 ) ;
#30379=EDGE_CURVE ( 'NONE', #26602, #38101, #43563, .T. ) ;
#30381=CARTESIAN_POINT ( 'NONE',  ( -336.3521761649653854, -100.7053649598255163, 55.50139289590170222 ) ) ;
#30385=ORIENTED_EDGE ( 'NONE', *, *, #15412, .T. ) ;
#30387=CARTESIAN_POINT ( 'NONE',  ( -336.3521761649654422, -141.9604555052315220, 56.09938080879057765 ) ) ;
#30389=DIRECTION ( 'NONE',  ( 0.000000000000000000, 0.000000000000000000, -1.000000000000000000 ) ) ;
#30390=DIRECTION ( 'NONE',  ( 0.000000000000000000, -1.000000000000000000, 0.000000000000000000 ) ) ;
#30393=EDGE_CURVE ( 'NONE', #5531, #45414, #7052, .T. ) ;
#30396=DIRECTION ( 'NONE',  ( -1.000000000000000000, -0.000000000000000000, 0.000000000000000000 ) ) ;
#30399=ORIENTED_EDGE ( 'NONE', *, *, #48967, .F. ) ;
#30404=CARTESIAN_POINT ( 'NONE',  ( -339.1964088526558498, -123.0000000000002700, -59.99791663049643375 ) ) ;
#30405=ORIENTED_EDGE ( 'NONE', *, *, #6777, .F. ) ;
#30409=EDGE_LOOP ( 'NONE', ( #8166, #37451, #41708, #24767 ) ) ;
#30410=DIRECTION ( 'NONE',  ( -1.000000000000000000, 0.000000000000000000, 0.000000000000000000 ) ) ;
#30418=VECTOR ( 'NONE', #18493, 1000.000000000000000 ) ;
#30420=DIRECTION ( 'NONE',  ( 0.000000000000000000, 1.000000000000000000, 0.000000000000000000 ) ) ;
#30421=ORIENTED_EDGE ( 'NONE', *, *, #155, .F. ) ;
#30425=LINE ( 'NONE', #21783, #45517 ) ;
#30426=ORIENTED_EDGE ( 'NONE', *, *, #39112, .F. ) ;
#30434=FACE_OUTER_BOUND ( 'NONE', #36872, .T. ) ;
#30438=DIRECTION ( 'NONE',  ( 0.000000000000000000, 0.000000000000000000, -1.000000000000000000 ) ) ;
#30439=DIRECTION ( 'NONE',  ( 0.000000000000000000, 0.000000000000000000, -1.000000000000000000 ) ) ;
#30442=EDGE_CURVE ( 'NONE', #30079, #39568, #19906, .T. ) ;
#30443=CARTESIAN_POINT ( 'NONE',  ( -330.4913330509368166, -162.2499814621210419, 44.49369547121568758 ) ) ;
#30447=AXIS2_PLACEMENT_3D ( 'NONE', #16238, #23593, #27788 ) ;
#30449=EDGE_CURVE ( 'NONE', #47538, #8253, #16763, .T. ) ;
#30451=VERTEX_POINT ( 'NONE', #32511 ) ;
#30453=AXIS2_PLACEMENT_3D ( 'NONE', #26940, #51652, #15656 ) ;
#30454=AXIS2_PLACEMENT_3D ( 'NONE', #3480, #19508, #43443 ) ;
#30456=ADVANCED_FACE ( 'NONE', ( #40905 ), #8587, .F. ) ;
#30457=CARTESIAN_POINT ( 'NONE',  ( -305.0000000000000568, -151.8251501453679850, 52.89315522109039591 ) ) ;
#30458=EDGE_CURVE ( 'NONE', #5935, #15465, #48560, .T. ) ;
#30461=FACE_OUTER_BOUND ( 'NONE', #37585, .T. ) ;
#30464=DIRECTION ( 'NONE',  ( -0.000000000000000000, -0.7485107481710953081, 0.6631226582408016323 ) ) ;
#30465=ORIENTED_EDGE ( 'NONE', *, *, #33241, .F. ) ;
#30471=VERTEX_POINT ( 'NONE', #15973 ) ;
#30472=EDGE_CURVE ( 'NONE', #42957, #43466, #31981, .T. ) ;
#30473=CARTESIAN_POINT ( 'NONE',  ( -330.4913330509368166, -182.1300919119129560, -6.615309698014691264 ) ) ;
#30474=CARTESIAN_POINT ( 'NONE',  ( -490.0000000000001137, -78.50000000000002842, 0.000000000000000000 ) ) ;
#30481=DIRECTION ( 'NONE',  ( -1.000000000000000000, 0.000000000000000000, 0.000000000000000000 ) ) ;
#30484=DIRECTION ( 'NONE',  ( -0.000000000000000000, -0.9709418174260502354, 0.2393156642875652051 ) ) ;
#30486=CARTESIAN_POINT ( 'NONE',  ( 0.000000000000000000, -68.33404168156053515, -20.92168833550964990 ) ) ;
#30487=LINE ( 'NONE', #38107, #28446 ) ;
#30490=VECTOR ( 'NONE', #28129, 1000.000000000000114 ) ;
#30491=DIRECTION ( 'NONE',  ( 0.000000000000000000, -1.000000000000000000, 0.000000000000000000 ) ) ;
#30494=LINE ( 'NONE', #26042, #17085 ) ;
#30495=ORIENTED_EDGE ( 'NONE', *, *, #22399, .F. ) ;
#30498=DIRECTION ( 'NONE',  ( -1.000000000000000000, 0.000000000000000000, 0.000000000000000000 ) ) ;
#30500=DIRECTION ( 'NONE',  ( -0.000000000000000000, -0.4647231720437724478, -0.8854560256532078011 ) ) ;
#30501=VECTOR ( 'NONE', #20355, 1000.000000000000227 ) ;
#30505=PLANE ( 'NONE',  #47202 ) ;
#30506=VECTOR ( 'NONE', #36430, 1000.000000000000000 ) ;
#30512=EDGE_CURVE ( 'NONE', #18084, #32311, #20414, .T. ) ;
#30518=DIRECTION ( 'NONE',  ( -1.000000000000000000, -0.000000000000000000, -0.000000000000000000 ) ) ;
#30521=VECTOR ( 'NONE', #739, 1000.000000000000000 ) ;
#30522=ORIENTED_EDGE ( 'NONE', *, *, #31727, .F. ) ;
#30524=LINE ( 'NONE', #34723, #14326 ) ;
#30526=LINE ( 'NONE', #42354, #9859 ) ;
#30530=ORIENTED_EDGE ( 'NONE', *, *, #23356, .T. ) ;
#30531=DIRECTION ( 'NONE',  ( -1.000000000000000000, 7.812315528781935576E-15, 6.921107616850706142E-15 ) ) ;
#30532=VERTEX_POINT ( 'NONE', #14106 ) ;
#30533=PLANE ( 'NONE',  #22432 ) ;
#30535=DIRECTION ( 'NONE',  ( -0.000000000000000000, 0.9350162426854194964, 0.3546048870425235200 ) ) ;
#30543=CARTESIAN_POINT ( 'NONE',  ( -332.3517673607765914, -177.7325358280884586, 23.38292116578760726 ) ) ;
#30545=EDGE_LOOP ( 'NONE', ( #42596, #35894, #7230, #32318 ) ) ;
#30548=VECTOR ( 'NONE', #18608, 1000.000000000000000 ) ;
#30549=ORIENTED_EDGE ( 'NONE', *, *, #20088, .T. ) ;
#30550=FACE_OUTER_BOUND ( 'NONE', #14207, .T. ) ;
#30551=ORIENTED_EDGE ( 'NONE', *, *, #39576, .T. ) ;
#30555=CARTESIAN_POINT ( 'NONE',  ( 0.000000000000000000, -96.08133284941780516, -52.24190551353947143 ) ) ;
#30559=ORIENTED_EDGE ( 'NONE', *, *, #38805, .F. ) ;
#30563=DIRECTION ( 'NONE',  ( 0.000000000000000000, 0.7485107481711089639, 0.6631226582407863113 ) ) ;
#30564=LINE ( 'NONE', #50559, #10234 ) ;
#30569=FACE_OUTER_BOUND ( 'NONE', #19584, .T. ) ;
#30573=DIRECTION ( 'NONE',  ( -0.000000000000000000, -0.9927088740980548609, -0.1205366802553164696 ) ) ;
#30582=ORIENTED_EDGE ( 'NONE', *, *, #51775, .F. ) ;
#30589=VECTOR ( 'NONE', #7271, 1000.000000000000000 ) ;
#30590=CARTESIAN_POINT ( 'NONE',  ( -330.4913330509368166, -167.9936954712150339, 38.74998146212178796 ) ) ;
#30594=ORIENTED_EDGE ( 'NONE', *, *, #24527, .F. ) ;
#30596=CARTESIAN_POINT ( 'NONE',  ( -336.3521761649653854, -149.9277501395804677, 53.86626052140529453 ) ) ;
#30601=EDGE_CURVE ( 'NONE', #23160, #27018, #5710, .T. ) ;
#30603=DIRECTION ( 'NONE',  ( 0.000000000000000000, -0.2393156642875547968, 0.9709418174260527890 ) ) ;
#30605=DIRECTION ( 'NONE',  ( 0.000000000000000000, -3.491481338843133355E-15, -1.000000000000000000 ) ) ;
#30610=DIRECTION ( 'NONE',  ( 0.000000000000000000, -0.1205366802553337752, -0.9927088740980526405 ) ) ;
#30617=CARTESIAN_POINT ( 'NONE',  ( -332.3517673607765914, -75.66382151296542702, -36.21739951675945690 ) ) ;
#30618=ORIENTED_EDGE ( 'NONE', *, *, #20787, .F. ) ;
#30619=CIRCLE ( 'NONE', #33149, 5.000000000000001776 ) ;
#30623=CIRCLE ( 'NONE', #47411, 60.00000000000000000 ) ;
#30628=EDGE_CURVE ( 'NONE', #13250, #28174, #45909, .T. ) ;
#30629=EDGE_LOOP ( 'NONE', ( #48993, #2444, #43048, #27947 ) ) ;
#30632=VERTEX_POINT ( 'NONE', #9631 ) ;
#30633=DIRECTION ( 'NONE',  ( 0.000000000000000000, 0.1205366802553233113, 0.9927088740980538617 ) ) ;
#30634=CARTESIAN_POINT ( 'NONE',  ( -330.4913330509368166, -137.1341532842523918, 57.40522506028099770 ) ) ;
#30635=DIRECTION ( 'NONE',  ( -1.000000000000000000, -0.000000000000000000, -0.000000000000000000 ) ) ;
#30643=CARTESIAN_POINT ( 'NONE',  ( -330.4913330509368166, -122.9999999999994600, 59.00000000000002132 ) ) ;
#30644=AXIS2_PLACEMENT_3D ( 'NONE', #37005, #29114, #16529 ) ;
#30646=DIRECTION ( 'NONE',  ( 0.000000000000000000, -0.9709418174260511236, 0.2393156642875615969 ) ) ;
#30649=VECTOR ( 'NONE', #44075, 999.9999999999998863 ) ;
#30653=VERTEX_POINT ( 'NONE', #13838 ) ;
#30657=ORIENTED_EDGE ( 'NONE', *, *, #40446, .F. ) ;
#30658=CARTESIAN_POINT ( 'NONE',  ( -365.0000000000001137, -78.50000000000002842, 0.000000000000000000 ) ) ;
#30660=DIRECTION ( 'NONE',  ( 1.000000000000000000, -0.000000000000000000, -0.000000000000000000 ) ) ;
#30665=ORIENTED_EDGE ( 'NONE', *, *, #36446, .F. ) ;
#30672=VERTEX_POINT ( 'NONE', #45137 ) ;
#30674=FACE_OUTER_BOUND ( 'NONE', #13366, .T. ) ;
#30676=EDGE_CURVE ( 'NONE', #14977, #32186, #6213, .T. ) ;
#30677=CARTESIAN_POINT ( 'NONE',  ( -339.1964088526558498, -178.8432607619606358, 20.45418021416736565 ) ) ;
#30678=LINE ( 'NONE', #25976, #6944 ) ;
#30680=DIRECTION ( 'NONE',  ( 0.000000000000000000, 0.3546048870425463906, 0.9350162426854107256 ) ) ;
#30690=DIRECTION ( 'NONE',  ( 0.000000000000000000, -0.8854560256532141294, -0.4647231720437604574 ) ) ;
#30691=EDGE_CURVE ( 'NONE', #2959, #8311, #44088, .T. ) ;
#30692=ORIENTED_EDGE ( 'NONE', *, *, #15427, .T. ) ;
#30693=EDGE_CURVE ( 'NONE', #21286, #47980, #29071, .T. ) ;
#30694=CARTESIAN_POINT ( 'NONE',  ( -339.1964088526558498, -178.8432607619609485, -20.45418021416653076 ) ) ;
#30695=ADVANCED_FACE ( 'NONE', ( #18040 ), #25154, .F. ) ;
#30696=DIRECTION ( 'NONE',  ( 1.000000000000000000, 0.000000000000000000, 0.000000000000000000 ) ) ;
#30701=FACE_OUTER_BOUND ( 'NONE', #38583, .T. ) ;
#30702=CIRCLE ( 'NONE', #41583, 60.00000000000000000 ) ;
#30703=CARTESIAN_POINT ( 'NONE',  ( -339.1964088526558498, -115.8919814278871598, -58.50955523165758621 ) ) ;
#30704=ORIENTED_EDGE ( 'NONE', *, *, #29013, .F. ) ;
#30705=DIRECTION ( 'NONE',  ( 1.000000000000000000, -0.000000000000000000, 0.000000000000000000 ) ) ;
#30717=AXIS2_PLACEMENT_3D ( 'NONE', #13566, #24361, #45130 ) ;
#30719=CARTESIAN_POINT ( 'NONE',  ( -332.3517673607765914, -82.40546666720629787, 42.41660376256258047 ) ) ;
#30720=AXIS2_PLACEMENT_3D ( 'NONE', #27311, #43354, #7096 ) ;
#30722=CARTESIAN_POINT ( 'NONE',  ( -336.3521761649654422, -98.41210887299327226, -53.46519113769058151 ) ) ;
#30727=DIRECTION ( 'NONE',  ( 1.043714542225393381E-14, 1.000000000000000000, -1.047444401652940007E-14 ) ) ;
#30729=ORIENTED_EDGE ( 'NONE', *, *, #38154, .F. ) ;
#30731=VERTEX_POINT ( 'NONE', #34817 ) ;
#30732=PLANE ( 'NONE',  #3496 ) ;
#30738=FACE_OUTER_BOUND ( 'NONE', #29579, .T. ) ;
#30740=DIRECTION ( 'NONE',  ( 0.000000000000000000, 0.1205366802553233113, 0.9927088740980538617 ) ) ;
#30745=EDGE_CURVE ( 'NONE', #35288, #46710, #14353, .T. ) ;
#30746=EDGE_LOOP ( 'NONE', ( #23278, #20069, #44556, #19797 ) ) ;
#30747=ADVANCED_FACE ( 'NONE', ( #18305 ), #31401, .T. ) ;
#30748=VECTOR ( 'NONE', #28656, 1000.000000000000000 ) ;
#30749=LINE ( 'NONE', #11029, #36360 ) ;
#30752=AXIS2_PLACEMENT_3D ( 'NONE', #48194, #44504, #4559 ) ;
#30759=EDGE_CURVE ( 'NONE', #4224, #23080, #6483, .T. ) ;
#30764=EDGE_CURVE ( 'NONE', #34791, #18286, #14609, .T. ) ;
#30766=VECTOR ( 'NONE', #24039, 1000.000000000000000 ) ;
#30768=AXIS2_PLACEMENT_3D ( 'NONE', #41884, #21663, #14035 ) ;
#30770=CARTESIAN_POINT ( 'NONE',  ( -339.1964088526558498, -68.51134412508150717, 21.38919645685156112 ) ) ;
#30771=CARTESIAN_POINT ( 'NONE',  ( -305.0000000000000568, -90.77207769297352513, -50.28800156563429624 ) ) ;
#30775=LINE ( 'NONE', #26054, #20983 ) ;
#30776=LINE ( 'NONE', #46307, #26312 ) ;
#30780=VECTOR ( 'NONE', #31624, 1000.000000000000000 ) ;
#30781=VERTEX_POINT ( 'NONE', #30617 ) ;
#30786=FACE_OUTER_BOUND ( 'NONE', #27107, .T. ) ;
#30789=AXIS2_PLACEMENT_3D ( 'NONE', #24162, #23877, #48063 ) ;
#30790=CARTESIAN_POINT ( 'NONE',  ( -339.1964088526558498, -102.1108035431478811, -54.98865587491830809 ) ) ;
#30794=ORIENTED_EDGE ( 'NONE', *, *, #48206, .F. ) ;
#30796=ORIENTED_EDGE ( 'NONE', *, *, #6675, .F. ) ;
#30797=CARTESIAN_POINT ( 'NONE',  ( -330.4913330509368166, -144.3080463282014989, 56.27632902032097917 ) ) ;
#30798=ORIENTED_EDGE ( 'NONE', *, *, #42140, .F. ) ;
#30800=FACE_OUTER_BOUND ( 'NONE', #16581, .T. ) ;
#30801=VERTEX_POINT ( 'NONE', #47192 ) ;
#30806=CIRCLE ( 'NONE', #47628, 60.00000000000000000 ) ;
#30812=ADVANCED_FACE ( 'NONE', ( #46416 ), #42731, .F. ) ;
#30814=ORIENTED_EDGE ( 'NONE', *, *, #37537, .F. ) ;
#30815=EDGE_CURVE ( 'NONE', #16981, #30632, #2271, .T. ) ;
#30816=CARTESIAN_POINT ( 'NONE',  ( -339.1964088526558498, -178.4886558749184076, -21.38919645685194837 ) ) ;
#30817=DIRECTION ( 'NONE',  ( 0.000000000000000000, -3.491481338843133355E-15, -1.000000000000000000 ) ) ;
#30818=ADVANCED_FACE ( 'NONE', ( #35596 ), #51926, .T. ) ;
#30820=DIRECTION ( 'NONE',  ( -0.000000000000000000, -0.8854560256532126861, -0.4647231720437631775 ) ) ;
#30822=CIRCLE ( 'NONE', #48464, 60.00000000000000000 ) ;
#30823=DIRECTION ( 'NONE',  ( 0.000000000000000000, -0.2393156642875652051, -0.9709418174260502354 ) ) ;
#30825=DIRECTION ( 'NONE',  ( 1.043714542225393223E-14, 0.9927088740980551940, 0.1205366802553130001 ) ) ;
#30829=CARTESIAN_POINT ( 'NONE',  ( -336.3521761649654422, -180.1556192733800117, 16.67542351306693149 ) ) ;
#30833=ORIENTED_EDGE ( 'NONE', *, *, #14695, .F. ) ;
#30839=CARTESIAN_POINT ( 'NONE',  ( -339.1964088526558498, -178.4886558749180949, 21.38919645685277970 ) ) ;
#30840=VERTEX_POINT ( 'NONE', #15915 ) ;
#30851=CARTESIAN_POINT ( 'NONE',  ( -339.1964088526558498, -116.8846903019852164, -58.63009191191289915 ) ) ;
#30859=EDGE_CURVE ( 'NONE', #47574, #12090, #24046, .T. ) ;
#30871=ORIENTED_EDGE ( 'NONE', *, *, #32453, .F. ) ;
#30872=ORIENTED_EDGE ( 'NONE', *, *, #23117, .F. ) ;
#30876=DIRECTION ( 'NONE',  ( 1.000000000000000000, -0.000000000000000000, -0.000000000000000000 ) ) ;
#30878=EDGE_CURVE ( 'NONE', #42173, #26071, #19581, .T. ) ;
#30880=EDGE_CURVE ( 'NONE', #17876, #11338, #24445, .T. ) ;
#30887=CARTESIAN_POINT ( 'NONE',  ( -336.3521761649654422, -97.52665284734005979, -53.00046796564681983 ) ) ;
#30892=LINE ( 'NONE', #10917, #46671 ) ;
#30893=CARTESIAN_POINT ( 'NONE',  ( -339.1964088526558498, -162.9117225908384796, 45.24064679492099117 ) ) ;
#30894=LINE ( 'NONE', #50876, #47145 ) ;
#30901=ORIENTED_EDGE ( 'NONE', *, *, #26615, .T. ) ;
#30904=ADVANCED_FACE ( 'NONE', ( #11942 ), #27979, .T. ) ;
#30906=DIRECTION ( 'NONE',  ( -1.000000000000000000, 0.000000000000000000, 0.000000000000000000 ) ) ;
#30909=DIRECTION ( 'NONE',  ( 1.000000000000000000, 0.000000000000000000, 0.000000000000000000 ) ) ;
#30912=CARTESIAN_POINT ( 'NONE',  ( -336.3521761649654422, -104.1045282520827300, -55.74477592174792306 ) ) ;
#30918=DIRECTION ( 'NONE',  ( -1.000000000000000000, 0.000000000000000000, -0.000000000000000000 ) ) ;
#30923=CARTESIAN_POINT ( 'NONE',  ( -330.4913330509368166, -66.09477493971897388, 13.63415328425216622 ) ) ;
#30924=ORIENTED_EDGE ( 'NONE', *, *, #10219, .T. ) ;
#30929=ORIENTED_EDGE ( 'NONE', *, *, #15630, .F. ) ;
#30933=DIRECTION ( 'NONE',  ( 0.000000000000000000, 0.000000000000000000, 1.000000000000000000 ) ) ;
#30934=DIRECTION ( 'NONE',  ( 0.000000000000000000, 0.6631226582407937498, -0.7485107481711024136 ) ) ;
#30942=DIRECTION ( 'NONE',  ( -1.000000000000000000, 0.000000000000000000, 0.000000000000000000 ) ) ;
#30944=LINE ( 'NONE', #4064, #15683 ) ;
#30956=VECTOR ( 'NONE', #34116, 1000.000000000000000 ) ;
#30958=EDGE_CURVE ( 'NONE', #5217, #50146, #4328, .T. ) ;
#30960=VECTOR ( 'NONE', #1049, 1000.000000000000000 ) ;
#30961=DIRECTION ( 'NONE',  ( -1.000000000000000000, -0.000000000000000000, -0.000000000000000000 ) ) ;
#30965=VECTOR ( 'NONE', #8594, 1000.000000000000114 ) ;
#30970=VERTEX_POINT ( 'NONE', #32448 ) ;
#30972=VERTEX_POINT ( 'NONE', #12468 ) ;
#30979=LINE ( 'NONE', #47024, #4649 ) ;
#30980=VERTEX_POINT ( 'NONE', #3548 ) ;
#30984=VECTOR ( 'NONE', #18628, 1000.000000000000000 ) ;
#30990=ADVANCED_FACE ( 'NONE', ( #36913 ), #33220, .F. ) ;
#31000=DIRECTION ( 'NONE',  ( 1.000000000000000000, 0.000000000000000000, -0.000000000000000000 ) ) ;
#31005=CARTESIAN_POINT ( 'NONE',  ( -330.4913330509368166, -67.22367097967895688, 20.80804632820126443 ) ) ;
#31006=FACE_OUTER_BOUND ( 'NONE', #39991, .T. ) ;
#31013=ORIENTED_EDGE ( 'NONE', *, *, #31999, .F. ) ;
#31016=DIRECTION ( 'NONE',  ( -0.000000000000000000, 0.4647231720437789981, 0.8854560256532044704 ) ) ;
#31022=CIRCLE ( 'NONE', #24314, 60.00000000000000000 ) ;
#31026=ORIENTED_EDGE ( 'NONE', *, *, #46490, .F. ) ;
#31031=ORIENTED_EDGE ( 'NONE', *, *, #30691, .T. ) ;
#31032=DIRECTION ( 'NONE',  ( -0.000000000000000000, 0.3546048870425331789, -0.9350162426854158326 ) ) ;
#31033=EDGE_CURVE ( 'NONE', #46014, #46919, #37761, .T. ) ;
#31039=CARTESIAN_POINT ( 'NONE',  ( -332.3517673607765914, -81.08339623743702873, -41.09453333279329712 ) ) ;
#31047=FACE_OUTER_BOUND ( 'NONE', #4607, .T. ) ;
#31051=LINE ( 'NONE', #11328, #2801 ) ;
#31053=DIRECTION ( 'NONE',  ( 0.000000000000000000, 0.8854560256532157947, 0.4647231720437573488 ) ) ;
#31055=EDGE_CURVE ( 'NONE', #8505, #15290, #899, .T. ) ;
#31056=LINE ( 'NONE', #43417, #50012 ) ;
#31057=ORIENTED_EDGE ( 'NONE', *, *, #44948, .F. ) ;
#31065=EDGE_CURVE ( 'NONE', #77, #36042, #8781, .T. ) ;
#31066=VERTEX_POINT ( 'NONE', #5123 ) ;
#31069=VERTEX_POINT ( 'NONE', #9838 ) ;
#31076=DIRECTION ( 'NONE',  ( 1.000000000000000000, 5.781354811211875074E-17, 6.525800561034969538E-17 ) ) ;
#31077=CARTESIAN_POINT ( 'NONE',  ( -336.3521761649654422, -153.2494431741581025, -51.01861988938816950 ) ) ;
#31082=DIRECTION ( 'NONE',  ( -1.000000000000000000, -0.000000000000000000, -0.000000000000000000 ) ) ;
#31083=CARTESIAN_POINT ( 'NONE',  ( -339.1964088526558498, -79.00630452878414189, 38.74998146212082162 ) ) ;
#31092=VECTOR ( 'NONE', #38847, 1000.000000000000000 ) ;
#31094=VERTEX_POINT ( 'NONE', #44799 ) ;
#31097=EDGE_CURVE ( 'NONE', #51539, #49907, #9323, .T. ) ;
#31101=DIRECTION ( 'NONE',  ( -1.000000000000000000, -0.000000000000000000, -0.000000000000000000 ) ) ;
#31102=PLANE ( 'NONE',  #45927 ) ;
#31103=ORIENTED_EDGE ( 'NONE', *, *, #38838, .T. ) ;
#31107=DIRECTION ( 'NONE',  ( -0.000000000000000000, 1.047444401652940007E-14, 1.000000000000000000 ) ) ;
#31109=DIRECTION ( 'NONE',  ( -0.000000000000000000, 0.6631226582407937498, -0.7485107481711024136 ) ) ;
#31112=DIRECTION ( 'NONE',  ( 1.043714542225393854E-14, -0.6631226582407965253, -0.7485107481711000821 ) ) ;
#31116=PLANE ( 'NONE',  #18941 ) ;
#31120=ORIENTED_EDGE ( 'NONE', *, *, #25581, .F. ) ;
#31122=FACE_OUTER_BOUND ( 'NONE', #3387, .T. ) ;
#31126=DIRECTION ( 'NONE',  ( 1.043714542225393381E-14, 0.1205366802553303057, 0.9927088740980530845 ) ) ;
#31127=ADVANCED_FACE ( 'NONE', ( #10345 ), #38460, .F. ) ;
#31128=LINE ( 'NONE', #43732, #38811 ) ;
#31132=ADVANCED_FACE ( 'NONE', ( #6672 ), #18498, .F. ) ;
#31133=ORIENTED_EDGE ( 'NONE', *, *, #36926, .T. ) ;
#31134=FACE_OUTER_BOUND ( 'NONE', #44668, .T. ) ;
#31141=CARTESIAN_POINT ( 'NONE',  ( -330.4913330509368166, -96.06030588028485795, -53.35787839313392311 ) ) ;
#31143=EDGE_CURVE ( 'NONE', #29348, #18800, #49534, .T. ) ;
#31144=PLANE ( 'NONE',  #20269 ) ;
#31148=ORIENTED_EDGE ( 'NONE', *, *, #1154, .F. ) ;
#31149=AXIS2_PLACEMENT_3D ( 'NONE', #33920, #30498, #18429 ) ;
#31154=LINE ( 'NONE', #47205, #3308 ) ;
#31155=EDGE_LOOP ( 'NONE', ( #25877, #20257, #7544, #43705 ) ) ;
#31160=LINE ( 'NONE', #6225, #26619 ) ;
#31167=EDGE_CURVE ( 'NONE', #50146, #4273, #48692, .T. ) ;
#31173=FACE_OUTER_BOUND ( 'NONE', #18553, .T. ) ;
#31178=VERTEX_POINT ( 'NONE', #2200 ) ;
#31181=CARTESIAN_POINT ( 'NONE',  ( -336.3521761649654422, -98.41210887299327226, -53.46519113769058151 ) ) ;
#31189=EDGE_LOOP ( 'NONE', ( #45, #17483, #5853, #36376 ) ) ;
#31190=CARTESIAN_POINT ( 'NONE',  ( -332.3517673607765914, -126.1322888500942270, -59.00000000000001421 ) ) ;
#31195=VERTEX_POINT ( 'NONE', #39235 ) ;
#31198=ORIENTED_EDGE ( 'NONE', *, *, #28258, .T. ) ;
#31210=DIRECTION ( 'NONE',  ( 1.000000000000000000, -0.000000000000000000, -0.000000000000000000 ) ) ;
#31213=CARTESIAN_POINT ( 'NONE',  ( -336.3521761649654422, -146.8829211657874794, -54.23253582808848705 ) ) ;
#31214=VERTEX_POINT ( 'NONE', #38961 ) ;
#31215=CARTESIAN_POINT ( 'NONE',  ( -336.3521761649654422, -72.01665693856799066, -28.86398714850468039 ) ) ;
#31221=VECTOR ( 'NONE', #41878, 1000.000000000000114 ) ;
#31224=VECTOR ( 'NONE', #30696, 1000.000000000000000 ) ;
#31226=PLANE ( 'NONE',  #36789 ) ;
#31227=ORIENTED_EDGE ( 'NONE', *, *, #12652, .F. ) ;
#31230=VECTOR ( 'NONE', #27235, 1000.000000000000000 ) ;
#31238=AXIS2_PLACEMENT_3D ( 'NONE', #17228, #38217, #37967 ) ;
#31241=ORIENTED_EDGE ( 'NONE', *, *, #46521, .F. ) ;
#31247=CARTESIAN_POINT ( 'NONE',  ( -336.3521761649654422, -179.5993808087905279, -18.46045550523168899 ) ) ;
#31250=VERTEX_POINT ( 'NONE', #47127 ) ;
#31251=DIRECTION ( 'NONE',  ( 0.000000000000000000, 0.1205366802553164696, -0.9927088740980548609 ) ) ;
#31254=FACE_OUTER_BOUND ( 'NONE', #45708, .T. ) ;
#31258=DIRECTION ( 'NONE',  ( -1.000000000000000000, 0.000000000000000000, 0.000000000000000000 ) ) ;
#31259=ORIENTED_EDGE ( 'NONE', *, *, #14446, .T. ) ;
#31272=VERTEX_POINT ( 'NONE', #35802 ) ;
#31274=EDGE_CURVE ( 'NONE', #18899, #43264, #28162, .T. ) ;
#31277=AXIS2_PLACEMENT_3D ( 'NONE', #33981, #13504, #29519 ) ;
#31283=EDGE_CURVE ( 'NONE', #232, #49593, #20549, .T. ) ;
#31288=EDGE_LOOP ( 'NONE', ( #6516, #28670, #40876, #41439 ) ) ;
#31292=AXIS2_PLACEMENT_3D ( 'NONE', #45635, #16475, #700 ) ;
#31296=PLANE ( 'NONE',  #29232 ) ;
#31297=CARTESIAN_POINT ( 'NONE',  ( -339.1964088526558498, -65.12585595286510909, 13.87297036558291197 ) ) ;
#31298=CARTESIAN_POINT ( 'NONE',  ( -330.4913330509368166, -95.63860483659048839, 52.00954392751722111 ) ) ;
#31302=CARTESIAN_POINT ( 'NONE',  ( -336.3521761649653854, -64.15626348514393840, -8.849911663702499709 ) ) ;
#31311=AXIS2_PLACEMENT_3D ( 'NONE', #6222, #39308, #34334 ) ;
#31313=DIRECTION ( 'NONE',  ( 0.000000000000000000, 0.4647231720437664526, -0.8854560256532110207 ) ) ;
#31317=VERTEX_POINT ( 'NONE', #7448 ) ;
#31319=LINE ( 'NONE', #47363, #44160 ) ;
#31321=FACE_BOUND ( 'NONE', #22139, .T. ) ;
#31323=PLANE ( 'NONE',  #43253 ) ;
#31326=PLANE ( 'NONE',  #45925 ) ;
#31334=CARTESIAN_POINT ( 'NONE',  ( -330.4913330509368166, -123.5000000000000284, 0.000000000000000000 ) ) ;
#31340=DIRECTION ( 'NONE',  ( 1.000000000000000000, -0.000000000000000000, -0.000000000000000000 ) ) ;
#31343=DIRECTION ( 'NONE',  ( 0.000000000000000000, 0.9350162426854194964, 0.3546048870425235200 ) ) ;
#31346=EDGE_CURVE ( 'NONE', #15571, #11734, #43446, .T. ) ;
#31351=EDGE_LOOP ( 'NONE', ( #16574, #38264, #30814, #37207 ) ) ;
#31358=CARTESIAN_POINT ( 'NONE',  ( -330.4913330509368166, -138.3439121830091665, 58.13482838284733845 ) ) ;
#31359=DIRECTION ( 'NONE',  ( 1.043714542225393697E-14, 0.7485107481710934207, -0.6631226582408039638 ) ) ;
#31368=AXIS2_PLACEMENT_3D ( 'NONE', #38580, #30680, #46735 ) ;
#31369=EDGE_LOOP ( 'NONE', ( #42987, #36111, #50934, #22851 ) ) ;
#31370=DIRECTION ( 'NONE',  ( -1.000000000000000000, -0.000000000000000000, -0.000000000000000000 ) ) ;
#31376=DIRECTION ( 'NONE',  ( 1.000000000000000000, 0.000000000000000000, -0.000000000000000000 ) ) ;
#31377=ORIENTED_EDGE ( 'NONE', *, *, #20009, .T. ) ;
#31379=DIRECTION ( 'NONE',  ( 0.000000000000000000, 0.000000000000000000, 1.000000000000000000 ) ) ;
#31382=LINE ( 'NONE', #3015, #50255 ) ;
#31384=VERTEX_POINT ( 'NONE', #44211 ) ;
#31389=EDGE_CURVE ( 'NONE', #47761, #9672, #4267, .T. ) ;
#31391=EDGE_CURVE ( 'NONE', #45944, #28183, #315, .T. ) ;
#31394=EDGE_CURVE ( 'NONE', #8493, #13356, #24490, .T. ) ;
#31395=LINE ( 'NONE', #11421, #41685 ) ;
#31396=EDGE_CURVE ( 'NONE', #8311, #5668, #36579, .T. ) ;
#31398=ORIENTED_EDGE ( 'NONE', *, *, #20419, .T. ) ;
#31399=ORIENTED_EDGE ( 'NONE', *, *, #39678, .T. ) ;
#31401=PLANE ( 'NONE',  #44931 ) ;
#31402=DIRECTION ( 'NONE',  ( -1.000000000000000000, -0.000000000000000000, -0.000000000000000000 ) ) ;
#31406=EDGE_LOOP ( 'NONE', ( #5389, #6906, #45375, #31830 ) ) ;
#31409=VECTOR ( 'NONE', #22223, 1000.000000000000114 ) ;
#31410=ADVANCED_FACE ( 'NONE', ( #3404 ), #19434, .F. ) ;
#31412=ORIENTED_EDGE ( 'NONE', *, *, #4295, .T. ) ;
#31416=ORIENTED_EDGE ( 'NONE', *, *, #2216, .F. ) ;
#31419=LINE ( 'NONE', #30912, #44567 ) ;
#31423=ORIENTED_EDGE ( 'NONE', *, *, #41660, .T. ) ;
#31430=DIRECTION ( 'NONE',  ( 0.000000000000000000, 0.000000000000000000, -1.000000000000000000 ) ) ;
#31438=LINE ( 'NONE', #34602, #3986 ) ;
#31440=VECTOR ( 'NONE', #5546, 1000.000000000000114 ) ;
#31443=CARTESIAN_POINT ( 'NONE',  ( -339.1964088526558498, -102.1108035431470427, 54.98865587491797413 ) ) ;
#31448=ADVANCED_FACE ( 'NONE', ( #4449 ), #4195, .F. ) ;
#31453=DIRECTION ( 'NONE',  ( 0.000000000000000000, -0.8854560256532141294, -0.4647231720437604574 ) ) ;
#31455=EDGE_CURVE ( 'NONE', #28202, #2676, #48073, .T. ) ;
#31457=LINE ( 'NONE', #22809, #30548 ) ;
#31465=EDGE_LOOP ( 'NONE', ( #22036, #9031, #34806, #32717 ) ) ;
#31468=DIRECTION ( 'NONE',  ( 0.000000000000000000, -0.3546048870425396182, -0.9350162426854132791 ) ) ;
#31474=DIRECTION ( 'NONE',  ( -0.000000000000000000, 0.1205366802553199113, -0.9927088740980544168 ) ) ;
#31479=CARTESIAN_POINT ( 'NONE',  ( 0.000000000000000000, -66.21443277186293130, -14.11962419296594362 ) ) ;
#31484=LINE ( 'NONE', #50967, #17489 ) ;
#31489=VECTOR ( 'NONE', #50714, 1000.000000000000000 ) ;
#31493=VERTEX_POINT ( 'NONE', #36771 ) ;
#31495=FACE_OUTER_BOUND ( 'NONE', #47031, .T. ) ;
#31496=ORIENTED_EDGE ( 'NONE', *, *, #21208, .F. ) ;
#31499=FACE_OUTER_BOUND ( 'NONE', #47657, .T. ) ;
#31501=DIRECTION ( 'NONE',  ( 0.000000000000000000, -8.095376221225100300E-15, -1.000000000000000000 ) ) ;
#31509=VECTOR ( 'NONE', #33664, 1000.000000000000114 ) ;
#31523=LINE ( 'NONE', #7617, #36333 ) ;
#31525=DIRECTION ( 'NONE',  ( 0.000000000000000000, 0.2393156642875548246, -0.9709418174260527890 ) ) ;
#31541=CARTESIAN_POINT ( 'NONE',  ( -339.1964088526558498, -70.14212160686619768, -27.43969411971537298 ) ) ;
#31543=ORIENTED_EDGE ( 'NONE', *, *, #49929, .T. ) ;
#31546=AXIS2_PLACEMENT_3D ( 'NONE', #22283, #10448, #21519 ) ;
#31548=CARTESIAN_POINT ( 'NONE',  ( -336.3521761649654422, -66.84438072661991725, -16.67542351306652648 ) ) ;
#31551=FACE_OUTER_BOUND ( 'NONE', #3257, .T. ) ;
#31566=AXIS2_PLACEMENT_3D ( 'NONE', #19177, #19680, #35445 ) ;
#31567=DIRECTION ( 'NONE',  ( 1.000000000000000000, -0.000000000000000000, -0.000000000000000000 ) ) ;
#31570=EDGE_LOOP ( 'NONE', ( #23530, #47084, #15231, #22291 ) ) ;
#31571=EDGE_CURVE ( 'NONE', #17630, #23609, #29648, .T. ) ;
#31576=DIRECTION ( 'NONE',  ( 1.000000000000000000, 0.000000000000000000, 0.000000000000000000 ) ) ;
#31578=ORIENTED_EDGE ( 'NONE', *, *, #21148, .T. ) ;
#31581=DIRECTION ( 'NONE',  ( -0.000000000000000000, -0.7485107481711046340, -0.6631226582407911962 ) ) ;
#31582=CARTESIAN_POINT ( 'NONE',  ( -330.4913330509368166, -102.1108035431478811, -54.98865587491830809 ) ) ;
#31584=DIRECTION ( 'NONE',  ( -0.000000000000000000, 0.6631226582407937498, -0.7485107481711024136 ) ) ;
#31585=ORIENTED_EDGE ( 'NONE', *, *, #2093, .T. ) ;
#31593=CARTESIAN_POINT ( 'NONE',  ( -330.4913330509368166, -179.4217241332784454, -21.74306257088698757 ) ) ;
#31594=PLANE ( 'NONE',  #23785 ) ;
#31598=EDGE_CURVE ( 'NONE', #17396, #2622, #4707, .T. ) ;
#31613=EDGE_LOOP ( 'NONE', ( #24661, #42573, #4370, #14087 ) ) ;
#31619=ORIENTED_EDGE ( 'NONE', *, *, #1149, .F. ) ;
#31621=CARTESIAN_POINT ( 'NONE',  ( -332.3517673607765914, -123.5000000000000284, 0.000000000000000000 ) ) ;
#31623=CIRCLE ( 'NONE', #3952, 60.00000000000000000 ) ;
#31624=DIRECTION ( 'NONE',  ( -0.000000000000000000, 0.8229838658936556861, -0.5680647467311569221 ) ) ;
#31638=PLANE ( 'NONE',  #14919 ) ;
#31641=CARTESIAN_POINT ( 'NONE',  ( -332.3517673607765914, -123.5000000000000284, 0.000000000000000000 ) ) ;
#31643=CIRCLE ( 'NONE', #37498, 60.00000000000000000 ) ;
#31644=CARTESIAN_POINT ( 'NONE',  ( -332.3517673607765914, -117.8908635894569272, -59.73723787327232060 ) ) ;
#31645=DIRECTION ( 'NONE',  ( -0.000000000000000000, 0.000000000000000000, -1.000000000000000000 ) ) ;
#31650=EDGE_CURVE ( 'NONE', #39961, #39674, #37020, .T. ) ;
#31652=AXIS2_PLACEMENT_3D ( 'NONE', #30474, #19174, #30227 ) ;
#31653=ORIENTED_EDGE ( 'NONE', *, *, #626, .T. ) ;
#31654=DIRECTION ( 'NONE',  ( 0.000000000000000000, 0.000000000000000000, -1.000000000000000000 ) ) ;
#31660=DIRECTION ( 'NONE',  ( 1.000000000000000000, -0.000000000000000000, 0.000000000000000000 ) ) ;
#31663=ORIENTED_EDGE ( 'NONE', *, *, #8216, .T. ) ;
#31664=CARTESIAN_POINT ( 'NONE',  ( -339.1964088526558498, -151.3613951634084742, 52.00954392751779665 ) ) ;
#31665=ORIENTED_EDGE ( 'NONE', *, *, #49465, .T. ) ;
#31670=DIRECTION ( 'NONE',  ( 0.000000000000000000, 6.938893903907228378E-14, -1.000000000000000000 ) ) ;
#31676=VECTOR ( 'NONE', #30633, 1000.000000000000114 ) ;
#31678=CARTESIAN_POINT ( 'NONE',  ( -332.3517673607765914, -76.43926241122620979, -35.68215131113738181 ) ) ;
#31680=DIRECTION ( 'NONE',  ( -0.000000000000000000, 0.000000000000000000, -1.000000000000000000 ) ) ;
#31682=DIRECTION ( 'NONE',  ( 0.000000000000000000, 0.000000000000000000, 1.000000000000000000 ) ) ;
#31684=CIRCLE ( 'NONE', #19093, 60.00000000000000000 ) ;
#31686=CARTESIAN_POINT ( 'NONE',  ( -339.1964088526558498, -131.1080185721133660, -58.50955523165751515 ) ) ;
#31690=ORIENTED_EDGE ( 'NONE', *, *, #6729, .F. ) ;
#31693=CARTESIAN_POINT ( 'NONE',  ( -339.1964088526558498, -137.1341532842523065, 57.40522506028101901 ) ) ;
#31698=EDGE_CURVE ( 'NONE', #22737, #15872, #8785, .T. ) ;
#31708=CIRCLE ( 'NONE', #9063, 60.00000000000000000 ) ;
#31710=EDGE_CURVE ( 'NONE', #2676, #1973, #9957, .T. ) ;
#31711=FACE_OUTER_BOUND ( 'NONE', #16366, .T. ) ;
#31712=VECTOR ( 'NONE', #47668, 1000.000000000000114 ) ;
#31720=ORIENTED_EDGE ( 'NONE', *, *, #7360, .T. ) ;
#31722=AXIS2_PLACEMENT_3D ( 'NONE', #21150, #12731, #49801 ) ;
#31725=DIRECTION ( 'NONE',  ( 1.000000000000000000, -0.000000000000000000, -0.000000000000000000 ) ) ;
#31726=CARTESIAN_POINT ( 'NONE',  ( -330.4913330509368166, -123.5000000000000284, 0.000000000000000000 ) ) ;
#31727=EDGE_CURVE ( 'NONE', #43845, #18286, #30180, .T. ) ;
#31729=DIRECTION ( 'NONE',  ( 1.000000000000000000, -0.000000000000000000, 0.000000000000000000 ) ) ;
#31732=DIRECTION ( 'NONE',  ( -1.000000000000000000, 0.000000000000000000, 0.000000000000000000 ) ) ;
#31739=CARTESIAN_POINT ( 'NONE',  ( -339.1964088526558498, -109.8658467157473666, -57.40522506028092664 ) ) ;
#31742=AXIS2_PLACEMENT_3D ( 'NONE', #3714, #31843, #8438 ) ;
#31757=PLANE ( 'NONE',  #47744 ) ;
#31761=EDGE_CURVE ( 'NONE', #49096, #6252, #10449, .T. ) ;
#31763=ADVANCED_FACE ( 'NONE', ( #30674 ), #46729, .F. ) ;
#31767=ORIENTED_EDGE ( 'NONE', *, *, #29562, .F. ) ;
#31770=ORIENTED_EDGE ( 'NONE', *, *, #31571, .F. ) ;
#31775=ORIENTED_EDGE ( 'NONE', *, *, #12136, .T. ) ;
#31776=PLANE ( 'NONE',  #15840 ) ;
#31791=LINE ( 'NONE', #8642, #30006 ) ;
#31798=DIRECTION ( 'NONE',  ( -0.000000000000000000, -0.9927088740980548609, -0.1205366802553164696 ) ) ;
#31800=ADVANCED_FACE ( 'NONE', ( #7298 ), #47766, .F. ) ;
#31802=ORIENTED_EDGE ( 'NONE', *, *, #3640, .F. ) ;
#31805=CARTESIAN_POINT ( 'NONE',  ( -336.3521761649654422, -168.7445418633863596, -37.90245108779149064 ) ) ;
#31806=CARTESIAN_POINT ( 'NONE',  ( -305.0000000000000568, -123.5000000000000284, 0.000000000000000000 ) ) ;
#31808=ORIENTED_EDGE ( 'NONE', *, *, #20635, .T. ) ;
#31814=DIRECTION ( 'NONE',  ( -0.000000000000000000, 0.8854560256532157947, 0.4647231720437573488 ) ) ;
#31818=ORIENTED_EDGE ( 'NONE', *, *, #46567, .F. ) ;
#31829=CARTESIAN_POINT ( 'NONE',  ( 0.000000000000000000, -162.6242368362071602, -44.16213414209478572 ) ) ;
#31830=ORIENTED_EDGE ( 'NONE', *, *, #49747, .F. ) ;
#31831=FACE_OUTER_BOUND ( 'NONE', #49510, .T. ) ;
#31836=CARTESIAN_POINT ( 'NONE',  ( -336.3521761649654422, -153.2494431741581025, -51.01861988938816950 ) ) ;
#31837=LINE ( 'NONE', #4240, #19834 ) ;
#31841=DIRECTION ( 'NONE',  ( -0.000000000000000000, 0.4647231720437789981, 0.8854560256532044704 ) ) ;
#31843=DIRECTION ( 'NONE',  ( 0.000000000000000000, 0.000000000000000000, 1.000000000000000000 ) ) ;
#31851=DIRECTION ( 'NONE',  ( 0.000000000000000000, 0.000000000000000000, -1.000000000000000000 ) ) ;
#31852=ADVANCED_FACE ( 'NONE', ( #27250 ), #47502, .F. ) ;
#31855=ORIENTED_EDGE ( 'NONE', *, *, #17369, .F. ) ;
#31868=ORIENTED_EDGE ( 'NONE', *, *, #49583, .T. ) ;
#31871=CARTESIAN_POINT ( 'NONE',  ( -332.3517673607765914, -171.9335100611925213, 35.41461708323791413 ) ) ;
#31880=ORIENTED_EDGE ( 'NONE', *, *, #9942, .F. ) ;
#31886=AXIS2_PLACEMENT_3D ( 'NONE', #18117, #34143, #29673 ) ;
#31898=LINE ( 'NONE', #350, #1477 ) ;
#31899=ORIENTED_EDGE ( 'NONE', *, *, #5689, .F. ) ;
#31900=EDGE_CURVE ( 'NONE', #40482, #46919, #39845, .T. ) ;
#31902=PLANE ( 'NONE',  #8581 ) ;
#31903=DIRECTION ( 'NONE',  ( 1.000000000000000000, 0.000000000000000000, 0.000000000000000000 ) ) ;
#31905=CYLINDRICAL_SURFACE ( 'NONE', #46058, 5.000000000000001776 ) ;
#31910=DIRECTION ( 'NONE',  ( 0.000000000000000000, 0.000000000000000000, -1.000000000000000000 ) ) ;
#31913=CARTESIAN_POINT ( 'NONE',  ( -336.3521761649654422, -165.9166037625627439, 41.09453333279358134 ) ) ;
#31920=ORIENTED_EDGE ( 'NONE', *, *, #10367, .T. ) ;
#31921=EDGE_LOOP ( 'NONE', ( #14224, #43431, #48509, #28123 ) ) ;
#31926=EDGE_CURVE ( 'NONE', #47587, #7980, #16215, .T. ) ;
#31929=EDGE_CURVE ( 'NONE', #46931, #20894, #26451, .T. ) ;
#31931=EDGE_LOOP ( 'NONE', ( #48956, #35350, #19045, #46226 ) ) ;
#31939=DIRECTION ( 'NONE',  ( -0.000000000000000000, 0.9709418174260544543, 0.2393156642875482465 ) ) ;
#31943=VECTOR ( 'NONE', #16847, 1000.000000000000000 ) ;
#31944=VECTOR ( 'NONE', #43105, 1000.000000000000000 ) ;
#31948=EDGE_CURVE ( 'NONE', #17967, #31195, #8329, .T. ) ;
#31967=VERTEX_POINT ( 'NONE', #28796 ) ;
#31973=CARTESIAN_POINT ( 'NONE',  ( -332.3517673607765914, -74.01670616005314685, 32.17247266903214609 ) ) ;
#31981=LINE ( 'NONE', #8343, #46624 ) ;
#31982=DIRECTION ( 'NONE',  ( 0.000000000000000000, 0.8229838658936575735, 0.5680647467311540355 ) ) ;
#31986=LINE ( 'NONE', #51723, #12869 ) ;
#31994=LINE ( 'NONE', #4161, #8439 ) ;
#31995=VERTEX_POINT ( 'NONE', #8573 ) ;
#31996=EDGE_CURVE ( 'NONE', #23080, #33448, #40618, .T. ) ;
#31999=EDGE_CURVE ( 'NONE', #21924, #37305, #4639, .T. ) ;
#32003=VECTOR ( 'NONE', #41418, 1000.000000000000000 ) ;
#32017=VERTEX_POINT ( 'NONE', #48551 ) ;
#32018=CARTESIAN_POINT ( 'NONE',  ( -336.3521761649654422, -181.7525362123217292, 9.724760635742144999 ) ) ;
#32023=CIRCLE ( 'NONE', #43769, 60.00000000000000000 ) ;
#32026=DIRECTION ( 'NONE',  ( 1.000000000000000000, 0.000000000000000000, 0.000000000000000000 ) ) ;
#32027=AXIS2_PLACEMENT_3D ( 'NONE', #13074, #9149, #20706 ) ;
#32029=DIRECTION ( 'NONE',  ( 0.000000000000000000, 0.000000000000000000, -1.000000000000000000 ) ) ;
#32030=CARTESIAN_POINT ( 'NONE',  ( -336.3521761649654422, -110.9652333097088217, -57.67619951860654481 ) ) ;
#32031=CARTESIAN_POINT ( 'NONE',  ( -336.3521761649654422, -141.9604555052315220, 56.09938080879057765 ) ) ;
#32035=EDGE_CURVE ( 'NONE', #26860, #41341, #20666, .T. ) ;
#32036=CARTESIAN_POINT ( 'NONE',  ( -336.3521761649654422, -158.3591674452439122, -47.62880233550485087 ) ) ;
#32038=FACE_OUTER_BOUND ( 'NONE', #3371, .T. ) ;
#32042=CARTESIAN_POINT ( 'NONE',  ( -339.1964088526558498, -182.1300919119128423, 6.615309698015510165 ) ) ;
#32043=EDGE_CURVE ( 'NONE', #41791, #51089, #25850, .T. ) ;
#32044=ORIENTED_EDGE ( 'NONE', *, *, #9249, .T. ) ;
#32046=EDGE_LOOP ( 'NONE', ( #20079, #34149, #47920, #50775 ) ) ;
#32055=CARTESIAN_POINT ( 'NONE',  ( -339.1964088526558498, -123.5000000000000284, 0.000000000000000000 ) ) ;
#32056=ORIENTED_EDGE ( 'NONE', *, *, #17702, .T. ) ;
#32063=AXIS2_PLACEMENT_3D ( 'NONE', #3827, #15924, #11955 ) ;
#32064=ORIENTED_EDGE ( 'NONE', *, *, #15285, .T. ) ;
#32067=VERTEX_POINT ( 'NONE', #26357 ) ;
#32070=ORIENTED_EDGE ( 'NONE', *, *, #27779, .F. ) ;
#32074=CARTESIAN_POINT ( 'NONE',  ( -339.1964088526558498, -64.86990808808717190, -6.615309698015097162 ) ) ;
#32075=LINE ( 'NONE', #23434, #9865 ) ;
#32082=ORIENTED_EDGE ( 'NONE', *, *, #28055, .T. ) ;
#32086=CARTESIAN_POINT ( 'NONE',  ( -305.0000000000000568, -97.97423230103774472, -54.29949524055093946 ) ) ;
#32098=PLANE ( 'NONE',  #45787 ) ;
#32099=AXIS2_PLACEMENT_3D ( 'NONE', #49570, #2500, #50597 ) ;
#32100=ORIENTED_EDGE ( 'NONE', *, *, #29434, .T. ) ;
#32111=EDGE_CURVE ( 'NONE', #16080, #43501, #449, .T. ) ;
#32118=LINE ( 'NONE', #4531, #26168 ) ;
#32119=VERTEX_POINT ( 'NONE', #14546 ) ;
#32120=VECTOR ( 'NONE', #17252, 999.9999999999998863 ) ;
#32121=ORIENTED_EDGE ( 'NONE', *, *, #22048, .T. ) ;
#32123=AXIS2_PLACEMENT_3D ( 'NONE', #2408, #22636, #38648 ) ;
#32129=CARTESIAN_POINT ( 'NONE',  ( -332.3517673607765914, -120.8677111499054320, 59.94223098458771659 ) ) ;
#32130=DIRECTION ( 'NONE',  ( 0.000000000000000000, 0.2393156642875547968, -0.9709418174260527890 ) ) ;
#32133=VECTOR ( 'NONE', #6603, 1000.000000000000000 ) ;
#32134=ORIENTED_EDGE ( 'NONE', *, *, #20083, .T. ) ;
#32135=VECTOR ( 'NONE', #49072, 1000.000000000000000 ) ;
#32138=VERTEX_POINT ( 'NONE', #3472 ) ;
#32139=DIRECTION ( 'NONE',  ( -1.000000000000000000, 0.000000000000000000, -0.000000000000000000 ) ) ;
#32140=CARTESIAN_POINT ( 'NONE',  ( -336.3521761649654422, -63.55776901541228341, -2.632288850093980503 ) ) ;
#32141=DIRECTION ( 'NONE',  ( 1.000000000000000000, 0.000000000000000000, 0.000000000000000000 ) ) ;
#32142=AXIS2_PLACEMENT_3D ( 'NONE', #21605, #41828, #25795 ) ;
#32151=EDGE_LOOP ( 'NONE', ( #47937, #31031, #395, #38367 ) ) ;
#32153=VERTEX_POINT ( 'NONE', #51081 ) ;
#32155=DIRECTION ( 'NONE',  ( -0.000000000000000000, 0.9927088740980544168, 0.1205366802553199113 ) ) ;
#32159=LINE ( 'NONE', #40034, #46379 ) ;
#32160=CARTESIAN_POINT ( 'NONE',  ( -336.3521761649654422, -120.8677111499054320, 59.00000000000000000 ) ) ;
#32161=VERTEX_POINT ( 'NONE', #18481 ) ;
#32162=ADVANCED_FACE ( 'NONE', ( #19503 ), #2960, .T. ) ;
#32167=EDGE_LOOP ( 'NONE', ( #9051, #43257, #40631, #7593 ) ) ;
#32174=CARTESIAN_POINT ( 'NONE',  ( -332.3517673607765914, -92.15051119686104641, -50.05135858667769355 ) ) ;
#32176=ADVANCED_FACE ( 'NONE', ( #51570 ), #26866, .F. ) ;
#32179=EDGE_LOOP ( 'NONE', ( #9421, #50313, #2992, #9060 ) ) ;
#32181=ORIENTED_EDGE ( 'NONE', *, *, #48138, .T. ) ;
#32183=CIRCLE ( 'NONE', #37209, 60.00000000000000000 ) ;
#32186=VERTEX_POINT ( 'NONE', #11627 ) ;
#32189=CARTESIAN_POINT ( 'NONE',  ( -336.3521761649654422, -87.81784868886214213, 47.06073758877343494 ) ) ;
#32191=LINE ( 'NONE', #32965, #51655 ) ;
#32198=CARTESIAN_POINT ( 'NONE',  ( -339.1964088526558498, -63.50208336950359467, -0.5000000000000457412 ) ) ;
#32201=ORIENTED_EDGE ( 'NONE', *, *, #13979, .F. ) ;
#32207=DIRECTION ( 'NONE',  ( -0.000000000000000000, 0.000000000000000000, -1.000000000000000000 ) ) ;
#32208=FACE_BOUND ( 'NONE', #51936, .T. ) ;
#32209=CARTESIAN_POINT ( 'NONE',  ( -330.4913330509368166, -131.1080185721132807, -58.50955523165751515 ) ) ;
#32213=ORIENTED_EDGE ( 'NONE', *, *, #21031, .T. ) ;
#32214=PLANE ( 'NONE',  #33178 ) ;
#32216=ORIENTED_EDGE ( 'NONE', *, *, #21443, .F. ) ;
#32221=VERTEX_POINT ( 'NONE', #36840 ) ;
#32223=ORIENTED_EDGE ( 'NONE', *, *, #11829, .T. ) ;
#32224=EDGE_CURVE ( 'NONE', #46894, #11150, #43258, .T. ) ;
#32230=AXIS2_PLACEMENT_3D ( 'NONE', #19955, #47308, #47568 ) ;
#32233=EDGE_CURVE ( 'NONE', #28874, #8885, #831, .T. ) ;
#32236=CARTESIAN_POINT ( 'NONE',  ( -336.3521761649654422, -148.5878911270064009, 53.46519113769075204 ) ) ;
#32246=ORIENTED_EDGE ( 'NONE', *, *, #34160, .F. ) ;
#32248=CARTESIAN_POINT ( 'NONE',  ( -330.4913330509368166, -124.0000000000001990, -59.00000000000002132 ) ) ;
#32249=CARTESIAN_POINT ( 'NONE',  ( -336.3521761649653854, -180.1590281025188460, -19.74220186498920881 ) ) ;
#32252=FACE_OUTER_BOUND ( 'NONE', #20893, .T. ) ;
#32253=ORIENTED_EDGE ( 'NONE', *, *, #19711, .T. ) ;
#32255=CARTESIAN_POINT ( 'NONE',  ( -336.3521761649653854, -67.99860710409808462, -22.79463504017392950 ) ) ;
#32256=EDGE_LOOP ( 'NONE', ( #37921, #7992, #16869, #17093 ) ) ;
#32267=EDGE_LOOP ( 'NONE', ( #48494, #23701, #30426, #52002 ) ) ;
#32268=CARTESIAN_POINT ( 'NONE',  ( -339.1964088526558498, -178.8432607619609485, -20.45418021416653076 ) ) ;
#32271=ORIENTED_EDGE ( 'NONE', *, *, #3657, .T. ) ;
#32273=EDGE_CURVE ( 'NONE', #28202, #28554, #44201, .T. ) ;
#32276=DIRECTION ( 'NONE',  ( 1.000000000000000000, -0.000000000000000000, -0.000000000000000000 ) ) ;
#32277=PLANE ( 'NONE',  #40060 ) ;
#32279=ORIENTED_EDGE ( 'NONE', *, *, #10826, .F. ) ;
#32280=ORIENTED_EDGE ( 'NONE', *, *, #51596, .T. ) ;
#32281=CARTESIAN_POINT ( 'NONE',  ( -336.3521761649654422, -67.40061919120938683, 18.46045550523129819 ) ) ;
#32284=CARTESIAN_POINT ( 'NONE',  ( 0.000000000000000000, -182.0698235717852924, -7.111664135063673342 ) ) ;
#32289=FACE_OUTER_BOUND ( 'NONE', #21039, .T. ) ;
#32291=EDGE_CURVE ( 'NONE', #9248, #16704, #23707, .T. ) ;
#32295=VECTOR ( 'NONE', #24538, 1000.000000000000114 ) ;
#32302=EDGE_LOOP ( 'NONE', ( #48949, #32934, #12600, #48500 ) ) ;
#32304=VECTOR ( 'NONE', #35407, 1000.000000000000114 ) ;
#32305=FACE_OUTER_BOUND ( 'NONE', #10389, .T. ) ;
#32307=AXIS2_PLACEMENT_3D ( 'NONE', #47544, #7077, #15223 ) ;
#32311=VERTEX_POINT ( 'NONE', #20027 ) ;
#32317=LINE ( 'NONE', #7402, #38463 ) ;
#32318=ORIENTED_EDGE ( 'NONE', *, *, #50057, .F. ) ;
#32320=DIRECTION ( 'NONE',  ( 1.000000000000000000, -0.000000000000000000, -0.000000000000000000 ) ) ;
#32321=DIRECTION ( 'NONE',  ( -1.000000000000000000, 0.000000000000000000, 0.000000000000000000 ) ) ;
#32322=DIRECTION ( 'NONE',  ( 0.000000000000000000, 0.1205366802553338029, 0.9927088740980527515 ) ) ;
#32323=ORIENTED_EDGE ( 'NONE', *, *, #40430, .T. ) ;
#32332=EDGE_CURVE ( 'NONE', #30086, #8637, #1325, .T. ) ;
#32336=LINE ( 'NONE', #16074, #51781 ) ;
#32340=CARTESIAN_POINT ( 'NONE',  ( -336.3521761649654422, -123.5000000000000284, 0.000000000000000000 ) ) ;
#32342=DIRECTION ( 'NONE',  ( 0.000000000000000000, -0.4647231720437725033, -0.8854560256532079121 ) ) ;
#32343=ORIENTED_EDGE ( 'NONE', *, *, #3173, .T. ) ;
#32345=VECTOR ( 'NONE', #13085, 1000.000000000000000 ) ;
#32346=DIRECTION ( 'NONE',  ( 1.000000000000000000, -0.000000000000000000, -0.000000000000000000 ) ) ;
#32347=DIRECTION ( 'NONE',  ( -0.000000000000000000, 0.000000000000000000, -1.000000000000000000 ) ) ;
#32348=EDGE_CURVE ( 'NONE', #5759, #50025, #51685, .T. ) ;
#32351=EDGE_LOOP ( 'NONE', ( #43665, #51179, #6407, #45826 ) ) ;
#32353=EDGE_CURVE ( 'NONE', #11613, #18519, #36567, .T. ) ;
#32354=AXIS2_PLACEMENT_3D ( 'NONE', #47880, #7661, #23685 ) ;
#32356=EDGE_CURVE ( 'NONE', #32186, #3877, #9699, .T. ) ;
#32358=EDGE_CURVE ( 'NONE', #16769, #49622, #6083, .T. ) ;
#32359=VERTEX_POINT ( 'NONE', #21064 ) ;
#32361=EDGE_LOOP ( 'NONE', ( #50270, #49278 ) ) ;
#32366=DIRECTION ( 'NONE',  ( 1.000000000000000000, -0.000000000000000000, 0.000000000000000000 ) ) ;
#32371=DIRECTION ( 'NONE',  ( -0.000000000000000000, -0.7485107481710953081, 0.6631226582408016323 ) ) ;
#32373=ORIENTED_EDGE ( 'NONE', *, *, #21504, .T. ) ;
#32377=DIRECTION ( 'NONE',  ( 0.000000000000000000, 0.5680647467311569221, 0.8229838658936556861 ) ) ;
#32378=EDGE_CURVE ( 'NONE', #16147, #13737, #13963, .T. ) ;
#32379=DIRECTION ( 'NONE',  ( -0.000000000000000000, -0.3546048870425396182, -0.9350162426854132791 ) ) ;
#32381=VERTEX_POINT ( 'NONE', #41542 ) ;
#32382=CIRCLE ( 'NONE', #13951, 60.00000000000000000 ) ;
#32388=VERTEX_POINT ( 'NONE', #1625 ) ;
#32390=VERTEX_POINT ( 'NONE', #9503 ) ;
#32396=ORIENTED_EDGE ( 'NONE', *, *, #3033, .F. ) ;
#32400=DIRECTION ( 'NONE',  ( 0.000000000000000000, -0.9709418174260544543, -0.2393156642875482465 ) ) ;
#32405=DIRECTION ( 'NONE',  ( -0.000000000000000000, 0.000000000000000000, -1.000000000000000000 ) ) ;
#32407=ADVANCED_FACE ( 'NONE', ( #1085 ), #2120, .T. ) ;
#32408=ORIENTED_EDGE ( 'NONE', *, *, #18127, .F. ) ;
#32412=CARTESIAN_POINT ( 'NONE',  ( -339.1964088526558498, -172.3400804610915600, -33.10432812419107051 ) ) ;
#32415=VERTEX_POINT ( 'NONE', #1867 ) ;
#32416=EDGE_CURVE ( 'NONE', #51152, #15690, #17911, .T. ) ;
#32417=DIRECTION ( 'NONE',  ( -8.718379230999705894E-17, -0.3546048870425235200, 0.9350162426854194964 ) ) ;
#32423=DIRECTION ( 'NONE',  ( 0.000000000000000000, -0.7485107481711069655, -0.6631226582407885317 ) ) ;
#32424=ORIENTED_EDGE ( 'NONE', *, *, #9720, .F. ) ;
#32428=AXIS2_PLACEMENT_3D ( 'NONE', #51134, #31126, #29257 ) ;
#32431=CARTESIAN_POINT ( 'NONE',  ( -336.3521761649654422, -110.9652333097088217, -57.67619951860654481 ) ) ;
#32434=AXIS2_PLACEMENT_3D ( 'NONE', #103, #2326, #18851 ) ;
#32437=DIRECTION ( 'NONE',  ( 1.000000000000000000, 0.000000000000000000, 0.000000000000000000 ) ) ;
#32440=PLANE ( 'NONE',  #26601 ) ;
#32446=EDGE_LOOP ( 'NONE', ( #44538, #51865, #30120, #34368 ) ) ;
#32448=CARTESIAN_POINT ( 'NONE',  ( -336.3521761649654422, -111.9361751271348879, -57.91551518289410438 ) ) ;
#32451=VERTEX_POINT ( 'NONE', #29717 ) ;
#32453=EDGE_CURVE ( 'NONE', #15240, #22737, #22105, .T. ) ;
#32454=LINE ( 'NONE', #4092, #16762 ) ;
#32455=VECTOR ( 'NONE', #48220, 1000.000000000000000 ) ;
#32463=CARTESIAN_POINT ( 'NONE',  ( 0.000000000000000000, -74.94395191227431496, -33.51582005713827783 ) ) ;
#32472=LINE ( 'NONE', #25120, #1635 ) ;
#32474=FACE_BOUND ( 'NONE', #22282, .T. ) ;
#32476=CARTESIAN_POINT ( 'NONE',  ( -332.3517673607765914, -149.4733471526596134, 53.00046796564699036 ) ) ;
#32480=CIRCLE ( 'NONE', #41709, 60.00000000000000000 ) ;
#32481=ORIENTED_EDGE ( 'NONE', *, *, #40396, .T. ) ;
#32484=ORIENTED_EDGE ( 'NONE', *, *, #4942, .F. ) ;
#32485=FACE_OUTER_BOUND ( 'NONE', #22213, .T. ) ;
#32492=ORIENTED_EDGE ( 'NONE', *, *, #20337, .T. ) ;
#32495=EDGE_CURVE ( 'NONE', #12363, #42035, #50240, .T. ) ;
#32496=DIRECTION ( 'NONE',  ( 1.000000000000000000, -0.000000000000000000, 0.000000000000000000 ) ) ;
#32499=CIRCLE ( 'NONE', #9026, 60.00000000000000000 ) ;
#32503=DIRECTION ( 'NONE',  ( -0.000000000000000000, 0.7485107481710999711, -0.6631226582407964143 ) ) ;
#32511=CARTESIAN_POINT ( 'NONE',  ( -330.4913330509368166, -137.3729703655831997, 58.37414404713486249 ) ) ;
#32513=FACE_OUTER_BOUND ( 'NONE', #4919, .T. ) ;
#32517=ORIENTED_EDGE ( 'NONE', *, *, #42378, .F. ) ;
#32522=ORIENTED_EDGE ( 'NONE', *, *, #48029, .T. ) ;
#32525=VERTEX_POINT ( 'NONE', #23142 ) ;
#32527=VECTOR ( 'NONE', #32678, 1000.000000000000000 ) ;
#32528=VECTOR ( 'NONE', #19949, 1000.000000000000000 ) ;
#32540=ORIENTED_EDGE ( 'NONE', *, *, #31650, .T. ) ;
#32543=VECTOR ( 'NONE', #46144, 1000.000000000000000 ) ;
#32546=FACE_OUTER_BOUND ( 'NONE', #49249, .T. ) ;
#32548=PLANE ( 'NONE',  #27108 ) ;
#32552=CARTESIAN_POINT ( 'NONE',  ( -330.4913330509368166, -115.7716958700755470, -59.50019592636139265 ) ) ;
#32553=ORIENTED_EDGE ( 'NONE', *, *, #11391, .T. ) ;
#32554=VECTOR ( 'NONE', #25240, 1000.000000000000114 ) ;
#32555=VERTEX_POINT ( 'NONE', #7107 ) ;
#32558=EDGE_CURVE ( 'NONE', #5960, #34734, #8859, .T. ) ;
#32563=SHAPE_DEFINITION_REPRESENTATION ( #46172, #33116 ) ;
#32565=DIRECTION ( 'NONE',  ( -0.000000000000000000, 0.9350162426854194964, 0.3546048870425235200 ) ) ;
#32567=FACE_OUTER_BOUND ( 'NONE', #12045, .T. ) ;
#32568=EDGE_LOOP ( 'NONE', ( #36731, #20533, #41139, #35099 ) ) ;
#32570=EDGE_LOOP ( 'NONE', ( #16617, #9260, #34246, #24694 ) ) ;
#32574=CARTESIAN_POINT ( 'NONE',  ( 0.000000000000000000, -130.6116641350635064, 58.56982357178529242 ) ) ;
#32580=DIRECTION ( 'NONE',  ( -0.000000000000000000, -0.1205366802553268363, -0.9927088740980534176 ) ) ;
#32581=CARTESIAN_POINT ( 'NONE',  ( -305.0000000000000568, -76.88706545914891421, 37.77875505479673279 ) ) ;
#32583=LINE ( 'NONE', #12605, #24523 ) ;
#32585=EDGE_CURVE ( 'NONE', #13145, #42367, #38388, .T. ) ;
#32589=VECTOR ( 'NONE', #23115, 1000.000000000000000 ) ;
#32596=EDGE_CURVE ( 'NONE', #11859, #44930, #35214, .T. ) ;
#32601=DIRECTION ( 'NONE',  ( -1.000000000000000000, -6.921107616850733752E-15, 7.812315528781911911E-15 ) ) ;
#32602=EDGE_LOOP ( 'NONE', ( #17736, #22658, #527, #45696 ) ) ;
#32605=VECTOR ( 'NONE', #46506, 1000.000000000000227 ) ;
#32608=DIRECTION ( 'NONE',  ( 0.000000000000000000, -0.6631226582407863113, 0.7485107481711089639 ) ) ;
#32609=LINE ( 'NONE', #28394, #21596 ) ;
#32610=CIRCLE ( 'NONE', #3207, 15.24495751795539000 ) ;
#32615=CARTESIAN_POINT ( 'NONE',  ( -336.3521761649654422, -76.43926241122620979, -35.68215131113738181 ) ) ;
#32618=LINE ( 'NONE', #5035, #11420 ) ;
#32621=ORIENTED_EDGE ( 'NONE', *, *, #9538, .F. ) ;
#32623=DIRECTION ( 'NONE',  ( -1.000000000000000000, 0.000000000000000000, 0.000000000000000000 ) ) ;
#32624=DIRECTION ( 'NONE',  ( 0.000000000000000000, 0.7485107481710999711, -0.6631226582407964143 ) ) ;
#32628=AXIS2_PLACEMENT_3D ( 'NONE', #41147, #4369, #8560 ) ;
#32631=ORIENTED_EDGE ( 'NONE', *, *, #35550, .F. ) ;
#32632=DIRECTION ( 'NONE',  ( -0.000000000000000000, 0.6631226582408039638, 0.7485107481710934207 ) ) ;
#32638=VECTOR ( 'NONE', #32580, 1000.000000000000227 ) ;
#32640=DIRECTION ( 'NONE',  ( 0.000000000000000000, 0.8854560256532093554, -0.4647231720437695057 ) ) ;
#32641=CARTESIAN_POINT ( 'NONE',  ( -339.1964088526558498, -115.8919814278862503, 58.50955523165745831 ) ) ;
#32644=ORIENTED_EDGE ( 'NONE', *, *, #38355, .T. ) ;
#32650=AXIS2_PLACEMENT_3D ( 'NONE', #42203, #22238, #34333 ) ;
#32656=CARTESIAN_POINT ( 'NONE',  ( -339.1964088526558498, -143.9541802141663709, 55.34326076196097688 ) ) ;
#32657=ORIENTED_EDGE ( 'NONE', *, *, #25379, .F. ) ;
#32661=CARTESIAN_POINT ( 'NONE',  ( -332.3517673607765914, -146.8829211657874794, -54.23253582808848705 ) ) ;
#32662=DIRECTION ( 'NONE',  ( 0.000000000000000000, 0.000000000000000000, -1.000000000000000000 ) ) ;
#32664=EDGE_LOOP ( 'NONE', ( #4349, #38658, #4382, #44802 ) ) ;
#32668=ORIENTED_EDGE ( 'NONE', *, *, #12429, .T. ) ;
#32670=ADVANCED_FACE ( 'NONE', ( #44662 ), #40692, .T. ) ;
#32678=DIRECTION ( 'NONE',  ( -1.000000000000000000, 0.000000000000000000, 0.000000000000000000 ) ) ;
#32679=VECTOR ( 'NONE', #36387, 1000.000000000000000 ) ;
#32680=ORIENTED_EDGE ( 'NONE', *, *, #24044, .F. ) ;
#32685=PLANE ( 'NONE',  #6622 ) ;
#32686=CARTESIAN_POINT ( 'NONE',  ( -339.1964088526558498, -143.9541802141663709, 55.34326076196097688 ) ) ;
#32690=VERTEX_POINT ( 'NONE', #43620 ) ;
#32691=CARTESIAN_POINT ( 'NONE',  ( -332.3517673607765914, -91.32752733096738496, -49.48329383994654052 ) ) ;
#32709=LINE ( 'NONE', #9069, #27393 ) ;
#32712=LINE ( 'NONE', #4597, #10037 ) ;
#32715=LINE ( 'NONE', #8792, #41545 ) ;
#32716=EDGE_CURVE ( 'NONE', #12665, #37026, #19694, .T. ) ;
#32717=ORIENTED_EDGE ( 'NONE', *, *, #16409, .F. ) ;
#32725=EDGE_CURVE ( 'NONE', #23338, #50146, #11806, .T. ) ;
#32728=CARTESIAN_POINT ( 'NONE',  ( -330.4913330509368166, -144.8891964568517778, 54.98865587491845730 ) ) ;
#32729=EDGE_CURVE ( 'NONE', #7333, #21574, #51784, .T. ) ;
#32730=DIRECTION ( 'NONE',  ( -1.000000000000000000, 0.000000000000000000, 0.000000000000000000 ) ) ;
#32731=FACE_BOUND ( 'NONE', #11678, .T. ) ;
#32732=CARTESIAN_POINT ( 'NONE',  ( -339.1964088526558498, -109.6270296344155923, 58.37414404713457117 ) ) ;
#32734=ADVANCED_FACE ( 'NONE', ( #32038 ), #12331, .T. ) ;
#32740=VERTEX_POINT ( 'NONE', #39914 ) ;
#32743=CARTESIAN_POINT ( 'NONE',  ( -339.1964088526558498, -182.5000000000000568, -0.4999999999999543698 ) ) ;
#32746=LINE ( 'NONE', #36415, #36837 ) ;
#32748=CARTESIAN_POINT ( 'NONE',  ( -336.3521761649654422, -65.24746378767824240, -9.724760635741734660 ) ) ;
#32752=ORIENTED_EDGE ( 'NONE', *, *, #5806, .F. ) ;
#32754=AXIS2_PLACEMENT_3D ( 'NONE', #48298, #12283, #12798 ) ;
#32766=EDGE_LOOP ( 'NONE', ( #36236, #18806, #27531, #27679 ) ) ;
#32768=ORIENTED_EDGE ( 'NONE', *, *, #28055, .F. ) ;
#32773=DIRECTION ( 'NONE',  ( -1.000000000000000000, -0.000000000000000000, -0.000000000000000000 ) ) ;
#32775=CIRCLE ( 'NONE', #50314, 60.00000000000000000 ) ;
#32780=CARTESIAN_POINT ( 'NONE',  ( -330.4913330509368166, -123.5000000000000284, 0.000000000000000000 ) ) ;
#32783=LINE ( 'NONE', #24135, #11769 ) ;
#32784=EDGE_LOOP ( 'NONE', ( #33818, #48973, #8182, #4081 ) ) ;
#32785=ORIENTED_EDGE ( 'NONE', *, *, #27363, .T. ) ;
#32786=CARTESIAN_POINT ( 'NONE',  ( -180.0000000000000568, -123.5000000000000284, 0.000000000000000000 ) ) ;
#32788=VECTOR ( 'NONE', #21412, 1000.000000000000000 ) ;
#32791=DIRECTION ( 'NONE',  ( -1.000000000000000000, 0.000000000000000000, 0.000000000000000000 ) ) ;
#32793=ADVANCED_FACE ( 'NONE', ( #40972 ), #22929, .T. ) ;
#32796=EDGE_LOOP ( 'NONE', ( #9142, #15251, #18263, #23317 ) ) ;
#32797=CARTESIAN_POINT ( 'NONE',  ( -339.1964088526558498, -66.09477493971894546, 13.63415328425207917 ) ) ;
#32798=( NAMED_UNIT ( * ) SI_UNIT ( $, .STERADIAN. ) SOLID_ANGLE_UNIT ( ) );
#32799=VERTEX_POINT ( 'NONE', #26859 ) ;
#32800=ORIENTED_EDGE ( 'NONE', *, *, #5076, .F. ) ;
#32801=LINE ( 'NONE', #24925, #8877 ) ;
#32807=ORIENTED_EDGE ( 'NONE', *, *, #9246, .T. ) ;
#32810=EDGE_LOOP ( 'NONE', ( #18367, #9638, #44391, #28352 ) ) ;
#32812=VERTEX_POINT ( 'NONE', #15062 ) ;
#32816=DIRECTION ( 'NONE',  ( 0.000000000000000000, -0.9927088740980548609, -0.1205366802553164696 ) ) ;
#32817=ORIENTED_EDGE ( 'NONE', *, *, #30878, .T. ) ;
#32821=CARTESIAN_POINT ( 'NONE',  ( -336.3521761649654422, -72.48138011061176655, -29.74944317415788930 ) ) ;
#32822=DIRECTION ( 'NONE',  ( 0.000000000000000000, -0.9709418174260544543, -0.2393156642875482742 ) ) ;
#32823=EDGE_LOOP ( 'NONE', ( #4926, #48768, #50852, #36388 ) ) ;
#32824=ORIENTED_EDGE ( 'NONE', *, *, #14943, .T. ) ;
#32828=LINE ( 'NONE', #40977, #37172 ) ;
#32832=VERTEX_POINT ( 'NONE', #50795 ) ;
#32834=CARTESIAN_POINT ( 'NONE',  ( -330.4913330509368166, -63.87926739338325888, 6.735595255825880479 ) ) ;
#32839=DIRECTION ( 'NONE',  ( 0.000000000000000000, -0.4647231720437573488, 0.8854560256532157947 ) ) ;
#32840=LINE ( 'NONE', #20766, #34408 ) ;
#32842=DIRECTION ( 'NONE',  ( 0.000000000000000000, 0.7485107481710977506, -0.6631226582407989678 ) ) ;
#32843=VERTEX_POINT ( 'NONE', #22419 ) ;
#32845=ORIENTED_EDGE ( 'NONE', *, *, #50656, .F. ) ;
#32849=LINE ( 'NONE', #40214, #41671 ) ;
#32850=DIRECTION ( 'NONE',  ( -0.000000000000000000, -0.2393156642875482742, 0.9709418174260544543 ) ) ;
#32851=CARTESIAN_POINT ( 'NONE',  ( -332.3517673607765914, -113.7752393642576720, 58.25253621232167944 ) ) ;
#32852=ORIENTED_EDGE ( 'NONE', *, *, #35002, .T. ) ;
#32857=CARTESIAN_POINT ( 'NONE',  ( -332.3517673607765914, -111.9361751271348879, -57.91551518289410438 ) ) ;
#32860=LINE ( 'NONE', #24997, #10753 ) ;
#32866=DIRECTION ( 'NONE',  ( -0.000000000000000000, 1.000000000000000000, -0.000000000000000000 ) ) ;
#32868=VERTEX_POINT ( 'NONE', #7156 ) ;
#32870=AXIS2_PLACEMENT_3D ( 'NONE', #22861, #6588, #31251 ) ;
#32874=AXIS2_PLACEMENT_3D ( 'NONE', #27661, #11635, #3735 ) ;
#32875=ADVANCED_FACE ( 'NONE', ( #46860 ), #10844, .F. ) ;
#32882=FACE_OUTER_BOUND ( 'NONE', #47633, .T. ) ;
#32888=EDGE_CURVE ( 'NONE', #38482, #42654, #31319, .T. ) ;
#32895=FACE_OUTER_BOUND ( 'NONE', #23001, .T. ) ;
#32906=VERTEX_POINT ( 'NONE', #6655 ) ;
#32912=ORIENTED_EDGE ( 'NONE', *, *, #38701, .T. ) ;
#32918=VECTOR ( 'NONE', #21610, 1000.000000000000000 ) ;
#32920=ORIENTED_EDGE ( 'NONE', *, *, #48824, .T. ) ;
#32922=ORIENTED_EDGE ( 'NONE', *, *, #20495, .T. ) ;
#32928=CARTESIAN_POINT ( 'NONE',  ( -336.3521761649654422, -140.1754235130667610, -56.65561927338005432 ) ) ;
#32934=ORIENTED_EDGE ( 'NONE', *, *, #44071, .T. ) ;
#32942=DIRECTION ( 'NONE',  ( 0.000000000000000000, -1.216619397818400625E-13, 1.000000000000000000 ) ) ;
#32943=LINE ( 'NONE', #9054, #567 ) ;
#32944=EDGE_CURVE ( 'NONE', #8829, #22651, #38439, .T. ) ;
#32950=ORIENTED_EDGE ( 'NONE', *, *, #9758, .F. ) ;
#32955=ORIENTED_EDGE ( 'NONE', *, *, #11621, .T. ) ;
#32961=LINE ( 'NONE', #2133, #8407 ) ;
#32965=CARTESIAN_POINT ( 'NONE',  ( -332.3517673607765914, -73.44864141332200802, 31.34948880313848107 ) ) ;
#32968=DIRECTION ( 'NONE',  ( 0.000000000000000000, 0.4647231720437724478, 0.8854560256532078011 ) ) ;
#32969=VECTOR ( 'NONE', #48817, 1000.000000000000000 ) ;
#32970=DIRECTION ( 'NONE',  ( 0.000000000000000000, -0.4647231720437724478, -0.8854560256532078011 ) ) ;
#32971=DIRECTION ( 'NONE',  ( 1.000000000000000000, -7.719741424018524829E-17, -4.051632851310624584E-17 ) ) ;
#32975=LINE ( 'NONE', #45353, #41696 ) ;
#32977=FACE_OUTER_BOUND ( 'NONE', #25114, .T. ) ;
#32979=DIRECTION ( 'NONE',  ( 0.000000000000000000, -0.8229838658936613482, -0.5680647467311485954 ) ) ;
#32985=ORIENTED_EDGE ( 'NONE', *, *, #3406, .T. ) ;
#32987=CARTESIAN_POINT ( 'NONE',  ( -336.3521761649654422, -87.81784868886214213, 47.06073758877343494 ) ) ;
#32990=LINE ( 'NONE', #29316, #39666 ) ;
#32995=FACE_OUTER_BOUND ( 'NONE', #49100, .T. ) ;
#32996=ORIENTED_EDGE ( 'NONE', *, *, #12762, .T. ) ;
#33006=CARTESIAN_POINT ( 'NONE',  ( -336.3521761649654422, -136.0347666902908372, 57.67619951860663718 ) ) ;
#33010=CARTESIAN_POINT ( 'NONE',  ( -332.3517673607765914, -177.7325358280884586, 23.38292116578760726 ) ) ;
#33023=CIRCLE ( 'NONE', #10370, 60.00000000000000000 ) ;
#33029=ADVANCED_FACE ( 'NONE', ( #24225 ), #27645, .T. ) ;
#33030=CIRCLE ( 'NONE', #39720, 60.00000000000000000 ) ;
#33032=LINE ( 'NONE', #5195, #30965 ) ;
#33033=DIRECTION ( 'NONE',  ( -1.000000000000000000, 0.000000000000000000, 0.000000000000000000 ) ) ;
#33037=EDGE_CURVE ( 'NONE', #43333, #22832, #44457, .T. ) ;
#33041=FACE_BOUND ( 'NONE', #21613, .T. ) ;
#33048=DIRECTION ( 'NONE',  ( 0.000000000000000000, -0.8229838658936494689, 0.5680647467311658039 ) ) ;
#33051=DIRECTION ( 'NONE',  ( 0.000000000000000000, -0.9709418174260534551, -0.2393156642875516327 ) ) ;
#33052=ORIENTED_EDGE ( 'NONE', *, *, #30168, .F. ) ;
#33056=LINE ( 'NONE', #9670, #37338 ) ;
#33057=AXIS2_PLACEMENT_3D ( 'NONE', #29136, #45198, #25720 ) ;
#33059=VECTOR ( 'NONE', #10924, 1000.000000000000000 ) ;
#33062=EDGE_CURVE ( 'NONE', #12928, #33549, #33422, .T. ) ;
#33063=ADVANCED_FACE ( 'NONE', ( #5302 ), #49700, .F. ) ;
#33069=EDGE_CURVE ( 'NONE', #1251, #38255, #1855, .T. ) ;
#33071=LINE ( 'NONE', #16807, #6111 ) ;
#33072=CARTESIAN_POINT ( 'NONE',  ( -332.3517673607765914, -160.6539403396202772, 45.90766452162722544 ) ) ;
#33080=VECTOR ( 'NONE', #27220, 1000.000000000000114 ) ;
#33085=VERTEX_POINT ( 'NONE', #1342 ) ;
#33086=ADVANCED_FACE ( 'NONE', ( #48923 ), #26036, .F. ) ;
#33089=PLANE ( 'NONE',  #38733 ) ;
#33091=ORIENTED_EDGE ( 'NONE', *, *, #29231, .F. ) ;
#33092=ORIENTED_EDGE ( 'NONE', *, *, #14379, .T. ) ;
#33098=AXIS2_PLACEMENT_3D ( 'NONE', #21633, #29752, #30026 ) ;
#33100=VECTOR ( 'NONE', #22087, 1000.000000000000000 ) ;
#33106=ORIENTED_EDGE ( 'NONE', *, *, #19483, .F. ) ;
#33108=EDGE_LOOP ( 'NONE', ( #12932, #5715, #6020, #11092 ) ) ;
#33112=DIRECTION ( 'NONE',  ( -0.000000000000000000, -0.8229838658936596829, -0.5680647467311510379 ) ) ;
#33114=LINE ( 'NONE', #28906, #9036 ) ;
#33116=SHAPE_REPRESENTATION ( 'Center Pivot Base Stud', ( #31742 ), #3199 ) ;
#33120=DIRECTION ( 'NONE',  ( 1.043714542225393697E-14, 0.8854560256532044704, -0.4647231720437789981 ) ) ;
#33123=ADVANCED_FACE ( 'NONE', ( #825 ), #37615, .F. ) ;
#33125=CARTESIAN_POINT ( 'NONE',  ( -336.3521761649654422, -178.0871407151310279, 22.44790492310219676 ) ) ;
#33126=DIRECTION ( 'NONE',  ( -0.000000000000000000, 0.4647231720437664526, -0.8854560256532110207 ) ) ;
#33127=ORIENTED_EDGE ( 'NONE', *, *, #6044, .F. ) ;
#33145=DIRECTION ( 'NONE',  ( 0.000000000000000000, 0.000000000000000000, -1.000000000000000000 ) ) ;
#33149=AXIS2_PLACEMENT_3D ( 'NONE', #49013, #44297, #16441 ) ;
#33152=VECTOR ( 'NONE', #28452, 1000.000000000000000 ) ;
#33163=ORIENTED_EDGE ( 'NONE', *, *, #14637, .T. ) ;
#33170=DIRECTION ( 'NONE',  ( -0.000000000000000000, -0.2393156642875615969, -0.9709418174260511236 ) ) ;
#33173=VECTOR ( 'NONE', #49588, 1000.000000000000000 ) ;
#33174=EDGE_CURVE ( 'NONE', #48781, #44562, #28251, .T. ) ;
#33178=AXIS2_PLACEMENT_3D ( 'NONE', #28273, #16459, #44564 ) ;
#33179=AXIS2_PLACEMENT_3D ( 'NONE', #2602, #5798, #2355 ) ;
#33186=VECTOR ( 'NONE', #29693, 1000.000000000000000 ) ;
#33190=ORIENTED_EDGE ( 'NONE', *, *, #38328, .F. ) ;
#33195=EDGE_LOOP ( 'NONE', ( #30665, #14764, #38694, #18000 ) ) ;
#33200=CARTESIAN_POINT ( 'NONE',  ( -332.3517673607765914, -75.87119766449505676, -34.85916744524372746 ) ) ;
#33205=PLANE ( 'NONE',  #23705 ) ;
#33208=VERTEX_POINT ( 'NONE', #26283 ) ;
#33214=CARTESIAN_POINT ( 'NONE',  ( -330.4913330509368166, -123.5000000000000284, 0.000000000000000000 ) ) ;
#33216=CARTESIAN_POINT ( 'NONE',  ( -330.4913330509368166, -116.7644047441735182, -59.62073260661671270 ) ) ;
#33219=VECTOR ( 'NONE', #2240, 1000.000000000000000 ) ;
#33220=PLANE ( 'NONE',  #36942 ) ;
#33223=AXIS2_PLACEMENT_3D ( 'NONE', #24294, #35338, #51390 ) ;
#33225=LINE ( 'NONE', #40844, #45877 ) ;
#33241=EDGE_CURVE ( 'NONE', #45545, #32138, #34939, .T. ) ;
#33242=DIRECTION ( 'NONE',  ( 0.000000000000000000, 0.000000000000000000, -1.000000000000000000 ) ) ;
#33243=FACE_OUTER_BOUND ( 'NONE', #14790, .T. ) ;
#33245=VECTOR ( 'NONE', #35925, 1000.000000000000000 ) ;
#33246=CIRCLE ( 'NONE', #40774, 60.00000000000000000 ) ;
#33249=EDGE_LOOP ( 'NONE', ( #8383, #11181, #25043, #31543 ) ) ;
#33253=EDGE_CURVE ( 'NONE', #15864, #10230, #18420, .T. ) ;
#33261=AXIS2_PLACEMENT_3D ( 'NONE', #29538, #12984, #12724 ) ;
#33262=DIRECTION ( 'NONE',  ( 1.000000000000000000, -0.000000000000000000, 0.000000000000000000 ) ) ;
#33265=DIRECTION ( 'NONE',  ( -1.000000000000000000, 0.000000000000000000, 0.000000000000000000 ) ) ;
#33271=VERTEX_POINT ( 'NONE', #3154 ) ;
#33282=CARTESIAN_POINT ( 'NONE',  ( -305.0000000000000568, -123.9999999999993747, 59.99791663049644086 ) ) ;
#33287=CARTESIAN_POINT ( 'NONE',  ( -305.0000000000000568, -82.50558083279611310, 43.81161486573607533 ) ) ;
#33289=AXIS2_PLACEMENT_3D ( 'NONE', #12384, #40233, #20270 ) ;
#33292=PLANE ( 'NONE',  #48968 ) ;
#33295=VECTOR ( 'NONE', #47107, 1000.000000000000000 ) ;
#33298=CARTESIAN_POINT ( 'NONE',  ( 0.000000000000000000, -157.0158200571384555, -48.55604808772557845 ) ) ;
#33299=EDGE_LOOP ( 'NONE', ( #34824, #11957, #22927, #15168 ) ) ;
#33300=VECTOR ( 'NONE', #16131, 1000.000000000000000 ) ;
#33304=AXIS2_PLACEMENT_3D ( 'NONE', #34777, #2221, #14840 ) ;
#33306=ORIENTED_EDGE ( 'NONE', *, *, #41392, .T. ) ;
#33314=ADVANCED_FACE ( 'NONE', ( #34183, #6599 ), #2891, .F. ) ;
#33315=LINE ( 'NONE', #4678, #36231 ) ;
#33320=DIRECTION ( 'NONE',  ( -0.000000000000000000, -0.6631226582407911962, 0.7485107481711046340 ) ) ;
#33321=LINE ( 'NONE', #21492, #51661 ) ;
#33323=FACE_OUTER_BOUND ( 'NONE', #27914, .T. ) ;
#33324=CARTESIAN_POINT ( 'NONE',  ( -336.3521761649654422, -113.7752393642576720, 58.25253621232167944 ) ) ;
#33328=VECTOR ( 'NONE', #48936, 999.9999999999998863 ) ;
#33329=EDGE_CURVE ( 'NONE', #27048, #36669, #11025, .T. ) ;
#33330=VERTEX_POINT ( 'NONE', #7101 ) ;
#33332=EDGE_LOOP ( 'NONE', ( #36127, #46238, #8144, #38963 ) ) ;
#33333=AXIS2_PLACEMENT_3D ( 'NONE', #5854, #36587, #49209 ) ;
#33334=EDGE_CURVE ( 'NONE', #23304, #13064, #23132, .T. ) ;
#33343=CARTESIAN_POINT ( 'NONE',  ( -332.3517673607765914, -123.5000000000000284, 0.000000000000000000 ) ) ;
#33353=VECTOR ( 'NONE', #23991, 1000.000000000000227 ) ;
#33354=CARTESIAN_POINT ( 'NONE',  ( -332.3517673607765914, -67.40061919120938683, 18.46045550523129819 ) ) ;
#33359=EDGE_LOOP ( 'NONE', ( #45374, #11690, #19667, #64 ) ) ;
#33360=DIRECTION ( 'NONE',  ( -0.000000000000000000, 0.000000000000000000, -1.000000000000000000 ) ) ;
#33369=DIRECTION ( 'NONE',  ( -1.000000000000000000, 0.000000000000000000, 0.000000000000000000 ) ) ;
#33370=CARTESIAN_POINT ( 'NONE',  ( -339.1964088526558498, -68.15673923803930734, -20.45418021416698551 ) ) ;
#33379=ORIENTED_EDGE ( 'NONE', *, *, #13723, .F. ) ;
#33381=CARTESIAN_POINT ( 'NONE',  ( -330.4913330509368166, -176.8578783931340581, -27.43969411971497152 ) ) ;
#33383=DIRECTION ( 'NONE',  ( -8.718379230999707126E-17, 0.8229838658936575735, 0.5680647467311540355 ) ) ;
#33385=VECTOR ( 'NONE', #32601, 1000.000000000000000 ) ;
#33389=CIRCLE ( 'NONE', #42602, 60.00000000000000000 ) ;
#33390=ORIENTED_EDGE ( 'NONE', *, *, #41256, .T. ) ;
#33391=AXIS2_PLACEMENT_3D ( 'NONE', #24416, #8900, #20464 ) ;
#33392=EDGE_CURVE ( 'NONE', #31250, #4273, #46196, .T. ) ;
#33399=VERTEX_POINT ( 'NONE', #38794 ) ;
#33405=ADVANCED_FACE ( 'NONE', ( #2301 ), #18338, .F. ) ;
#33406=CARTESIAN_POINT ( 'NONE',  ( -339.1964088526558498, -95.63860483659040312, 52.00954392751717847 ) ) ;
#33409=EDGE_LOOP ( 'NONE', ( #49215, #26199, #620, #21837 ) ) ;
#33422=LINE ( 'NONE', #13181, #49244 ) ;
#33426=CARTESIAN_POINT ( 'NONE',  ( -330.4913330509368166, -123.5000000000000284, 0.000000000000000000 ) ) ;
#33427=EDGE_CURVE ( 'NONE', #32311, #46014, #43009, .T. ) ;
#33437=DIRECTION ( 'NONE',  ( -1.000000000000000000, 0.000000000000000000, 0.000000000000000000 ) ) ;
#33439=VERTEX_POINT ( 'NONE', #18831 ) ;
#33440=ORIENTED_EDGE ( 'NONE', *, *, #44543, .F. ) ;
#33448=VERTEX_POINT ( 'NONE', #43780 ) ;
#33453=AXIS2_PLACEMENT_3D ( 'NONE', #29739, #45789, #48952 ) ;
#33455=CARTESIAN_POINT ( 'NONE',  ( -332.3517673607765914, -123.5000000000000284, 0.000000000000000000 ) ) ;
#33456=ORIENTED_EDGE ( 'NONE', *, *, #35981, .T. ) ;
#33458=VECTOR ( 'NONE', #42214, 999.9999999999998863 ) ;
#33460=ORIENTED_EDGE ( 'NONE', *, *, #34651, .F. ) ;
#33463=ORIENTED_EDGE ( 'NONE', *, *, #18868, .T. ) ;
#33468=FACE_OUTER_BOUND ( 'NONE', #47674, .T. ) ;
#33469=EDGE_CURVE ( 'NONE', #17674, #27996, #8045, .T. ) ;
#33470=VECTOR ( 'NONE', #14984, 999.9999999999998863 ) ;
#33475=ORIENTED_EDGE ( 'NONE', *, *, #10219, .F. ) ;
#33478=CARTESIAN_POINT ( 'NONE',  ( -336.3521761649654422, -101.0520950768976149, 54.58714071513087873 ) ) ;
#33479=FACE_OUTER_BOUND ( 'NONE', #44386, .T. ) ;
#33480=VERTEX_POINT ( 'NONE', #15167 ) ;
#33496=EDGE_LOOP ( 'NONE', ( #16105, #31770, #8440, #42252 ) ) ;
#33505=LINE ( 'NONE', #37170, #8651 ) ;
#33507=DIRECTION ( 'NONE',  ( -8.718379230999704661E-17, 0.9927088740980544168, 0.1205366802553199113 ) ) ;
#33510=CARTESIAN_POINT ( 'NONE',  ( -330.4913330509368166, -90.39567187580871632, -48.84008046109136814 ) ) ;
#33516=DIRECTION ( 'NONE',  ( -0.000000000000000000, -0.5680647467311596976, -0.8229838658936536877 ) ) ;
#33521=FACE_OUTER_BOUND ( 'NONE', #29544, .T. ) ;
#33528=CARTESIAN_POINT ( 'NONE',  ( -336.3521761649654422, -76.88706545914891421, 37.77875505479673279 ) ) ;
#33532=CARTESIAN_POINT ( 'NONE',  ( -339.1964088526558498, -109.8658467157473666, -57.40522506028092664 ) ) ;
#33536=ORIENTED_EDGE ( 'NONE', *, *, #45292, .F. ) ;
#33539=LINE ( 'NONE', #13031, #32120 ) ;
#33545=CARTESIAN_POINT ( 'NONE',  ( 0.000000000000000000, -180.7855672281372108, -14.11962419296555105 ) ) ;
#33547=DIRECTION ( 'NONE',  ( 0.000000000000000000, -0.2393156642875685636, -0.9709418174260492362 ) ) ;
#33549=VERTEX_POINT ( 'NONE', #51432 ) ;
#33550=VECTOR ( 'NONE', #43758, 1000.000000000000000 ) ;
#33565=EDGE_LOOP ( 'NONE', ( #14689, #41205, #4044, #10398 ) ) ;
#33568=VERTEX_POINT ( 'NONE', #28005 ) ;
#33569=CARTESIAN_POINT ( 'NONE',  ( -332.3517673607765914, -140.1754235130667610, -56.65561927338005432 ) ) ;
#33571=ORIENTED_EDGE ( 'NONE', *, *, #19478, .F. ) ;
#33577=VERTEX_POINT ( 'NONE', #39821 ) ;
#33580=ORIENTED_EDGE ( 'NONE', *, *, #13391, .T. ) ;
#33583=CARTESIAN_POINT ( 'NONE',  ( -330.4913330509368166, -183.1207326066166559, 6.735595255827131922 ) ) ;
#33584=DIRECTION ( 'NONE',  ( 1.000000000000000000, -0.000000000000000000, 0.000000000000000000 ) ) ;
#33593=DIRECTION ( 'NONE',  ( -0.000000000000000000, 0.7485107481711069655, 0.6631226582407885317 ) ) ;
#33597=PLANE ( 'NONE',  #31546 ) ;
#33600=EDGE_CURVE ( 'NONE', #2622, #46969, #34969, .T. ) ;
#33602=PLANE ( 'NONE',  #4390 ) ;
#33604=LINE ( 'NONE', #33354, #3680 ) ;
#33609=ORIENTED_EDGE ( 'NONE', *, *, #5233, .F. ) ;
#33611=CARTESIAN_POINT ( 'NONE',  ( -339.1964088526558498, -182.5000000000000568, -0.4999999999999543698 ) ) ;
#33612=VERTEX_POINT ( 'NONE', #34269 ) ;
#33613=FACE_OUTER_BOUND ( 'NONE', #43804, .T. ) ;
#33616=EDGE_CURVE ( 'NONE', #7764, #6309, #27140, .T. ) ;
#33623=ADVANCED_FACE ( 'NONE', ( #6426 ), #50315, .F. ) ;
#33624=FACE_OUTER_BOUND ( 'NONE', #33359, .T. ) ;
#33631=CARTESIAN_POINT ( 'NONE',  ( -305.0000000000000568, -183.2372378732723632, -5.609136410542876483 ) ) ;
#33635=DIRECTION ( 'NONE',  ( 1.000000000000000000, 0.000000000000000000, 0.000000000000000000 ) ) ;
#33636=DIRECTION ( 'NONE',  ( 0.000000000000000000, 0.000000000000000000, -1.000000000000000000 ) ) ;
#33642=ORIENTED_EDGE ( 'NONE', *, *, #793, .T. ) ;
#33644=VERTEX_POINT ( 'NONE', #6679 ) ;
#33646=DIRECTION ( 'NONE',  ( -1.000000000000000000, -0.000000000000000000, -0.000000000000000000 ) ) ;
#33647=PLANE ( 'NONE',  #29151 ) ;
#33652=FACE_OUTER_BOUND ( 'NONE', #383, .T. ) ;
#33661=ORIENTED_EDGE ( 'NONE', *, *, #49052, .T. ) ;
#33663=DIRECTION ( 'NONE',  ( -1.000000000000000000, 0.000000000000000000, 0.000000000000000000 ) ) ;
#33664=DIRECTION ( 'NONE',  ( -0.9993908270190956511, 4.273955692857142571E-18, -0.03489949670250096919 ) ) ;
#33665=EDGE_CURVE ( 'NONE', #7704, #28470, #22698, .T. ) ;
#33666=CARTESIAN_POINT ( 'NONE',  ( -305.0000000000000568, -168.7406467949206785, -39.41172259083884910 ) ) ;
#33668=DIRECTION ( 'NONE',  ( -0.000000000000000000, -0.9927088740980534176, 0.1205366802553268502 ) ) ;
#33671=CIRCLE ( 'NONE', #20236, 60.00000000000000000 ) ;
#33674=ADVANCED_FACE ( 'NONE', ( #35290 ), #18502, .F. ) ;
#33677=CARTESIAN_POINT ( 'NONE',  ( -336.3521761649654422, -170.5607375887735770, 35.68215131113770155 ) ) ;
#33679=AXIS2_PLACEMENT_3D ( 'NONE', #40062, #374, #23527 ) ;
#33683=ORIENTED_EDGE ( 'NONE', *, *, #27610, .F. ) ;
#33689=LINE ( 'NONE', #21874, #30372 ) ;
#33695=LINE ( 'NONE', #5337, #107 ) ;
#33696=CARTESIAN_POINT ( 'NONE',  ( -339.1964088526558498, -175.5095439275177398, -27.86139516340860212 ) ) ;
#33700=CARTESIAN_POINT ( 'NONE',  ( -332.3517673607765914, -69.26746417191145611, -23.38292116578723068 ) ) ;
#33715=PLANE ( 'NONE',  #48496 ) ;
#33716=ORIENTED_EDGE ( 'NONE', *, *, #10815, .T. ) ;
#33718=ADVANCED_FACE ( 'NONE', ( #43698 ), #43950, .T. ) ;
#33719=EDGE_CURVE ( 'NONE', #1947, #15758, #3487, .T. ) ;
#33727=CARTESIAN_POINT ( 'NONE',  ( -336.3521761649654422, -123.5000000000000284, 0.000000000000000000 ) ) ;
#33729=VECTOR ( 'NONE', #35630, 1000.000000000000000 ) ;
#33736=CARTESIAN_POINT ( 'NONE',  ( -336.3521761649654422, -145.9479049231020440, -54.58714071513102795 ) ) ;
#33738=ORIENTED_EDGE ( 'NONE', *, *, #28506, .F. ) ;
#33739=DIRECTION ( 'NONE',  ( -0.000000000000000000, 0.1205366802553199113, -0.9927088740980544168 ) ) ;
#33746=CYLINDRICAL_SURFACE ( 'NONE', #48378, 5.000000000000001776 ) ;
#33747=AXIS2_PLACEMENT_3D ( 'NONE', #47374, #30825, #6910 ) ;
#33748=EDGE_CURVE ( 'NONE', #8114, #49438, #15859, .T. ) ;
#33751=EDGE_LOOP ( 'NONE', ( #3491, #46309, #35968, #16872 ) ) ;
#33753=ORIENTED_EDGE ( 'NONE', *, *, #1257, .F. ) ;
#33754=PLANE ( 'NONE',  #31722 ) ;
#33757=DIRECTION ( 'NONE',  ( -0.000000000000000000, -0.8854560256532079121, 0.4647231720437724478 ) ) ;
#33759=VECTOR ( 'NONE', #46820, 1000.000000000000000 ) ;
#33760=EDGE_LOOP ( 'NONE', ( #28060, #4464, #39377, #10332 ) ) ;
#33763=CARTESIAN_POINT ( 'NONE',  ( -336.3521761649654422, -182.3871109312487420, -4.498567634386014369 ) ) ;
#33764=DIRECTION ( 'NONE',  ( -0.000000000000000000, -0.6631226582407964143, -0.7485107481710999711 ) ) ;
#33767=LINE ( 'NONE', #21692, #37094 ) ;
#33769=EDGE_LOOP ( 'NONE', ( #20262, #51558, #6109, #22774, #36923 ) ) ;
#33773=ORIENTED_EDGE ( 'NONE', *, *, #22902, .T. ) ;
#33775=PLANE ( 'NONE',  #17437 ) ;
#33778=DIRECTION ( 'NONE',  ( -1.000000000000000000, 0.000000000000000000, -0.000000000000000000 ) ) ;
#33784=CIRCLE ( 'NONE', #32123, 60.00000000000000000 ) ;
#33786=DIRECTION ( 'NONE',  ( -0.000000000000000000, -0.9927088740980530845, 0.1205366802553303057 ) ) ;
#33792=DIRECTION ( 'NONE',  ( -8.718379230999707126E-17, 0.000000000000000000, -1.000000000000000000 ) ) ;
#33793=VECTOR ( 'NONE', #1227, 999.9999999999998863 ) ;
#33794=AXIS2_PLACEMENT_3D ( 'NONE', #1470, #33778, #38233 ) ;
#33795=LINE ( 'NONE', #45903, #11036 ) ;
#33798=AXIS2_PLACEMENT_3D ( 'NONE', #2832, #31729, #39847 ) ;
#33807=ADVANCED_FACE ( 'NONE', ( #23721 ), #27668, .F. ) ;
#33814=LINE ( 'NONE', #13852, #35766 ) ;
#33815=ORIENTED_EDGE ( 'NONE', *, *, #2576, .T. ) ;
#33817=AXIS2_PLACEMENT_3D ( 'NONE', #10097, #12986, #6166 ) ;
#33818=ORIENTED_EDGE ( 'NONE', *, *, #51528, .F. ) ;
#33819=CARTESIAN_POINT ( 'NONE',  ( -336.3521761649654422, -75.66382151296542702, -36.21739951675945690 ) ) ;
#33825=AXIS2_PLACEMENT_3D ( 'NONE', #21325, #33917, #46538 ) ;
#33829=CARTESIAN_POINT ( 'NONE',  ( -339.1964088526558498, -162.9984922102927385, -43.83057281297435992 ) ) ;
#33830=EDGE_LOOP ( 'NONE', ( #19870, #17213, #11906, #42941 ) ) ;
#33831=FACE_OUTER_BOUND ( 'NONE', #13231, .T. ) ;
#33833=VECTOR ( 'NONE', #36845, 1000.000000000000000 ) ;
#33840=ADVANCED_FACE ( 'NONE', ( #48427 ), #39487, .T. ) ;
#33843=ORIENTED_EDGE ( 'NONE', *, *, #1663, .F. ) ;
#33846=VERTEX_POINT ( 'NONE', #36324 ) ;
#33848=DIRECTION ( 'NONE',  ( 1.000000000000000000, 0.000000000000000000, -0.000000000000000000 ) ) ;
#33856=CARTESIAN_POINT ( 'NONE',  ( -336.3521761649654422, -76.43926241122620979, -35.68215131113738181 ) ) ;
#33858=VERTEX_POINT ( 'NONE', #21342 ) ;
#33860=CARTESIAN_POINT ( 'NONE',  ( -336.3521761649654422, -159.1821513111375452, -47.06073758877369073 ) ) ;
#33861=PLANE ( 'NONE',  #17343 ) ;
#33863=EDGE_CURVE ( 'NONE', #50025, #37621, #5060, .T. ) ;
#33872=CARTESIAN_POINT ( 'NONE',  ( -330.4913330509368166, -108.8949048983204904, 57.16590939599316812 ) ) ;
#33873=DIRECTION ( 'NONE',  ( -1.000000000000000000, -1.258058860540533984E-15, -1.036104688092336048E-14 ) ) ;
#33887=DIRECTION ( 'NONE',  ( 0.000000000000000000, 0.9927088740980556381, 0.1205366802553095168 ) ) ;
#33891=ORIENTED_EDGE ( 'NONE', *, *, #52012, .F. ) ;
#33896=ADVANCED_FACE ( 'NONE', ( #48688 ), #1366, .F. ) ;
#33898=LINE ( 'NONE', #814, #3107 ) ;
#33899=DIRECTION ( 'NONE',  ( -1.000000000000000000, -0.000000000000000000, -0.000000000000000000 ) ) ;
#33901=CIRCLE ( 'NONE', #39773, 60.00000000000000000 ) ;
#33905=ORIENTED_EDGE ( 'NONE', *, *, #46090, .T. ) ;
#33912=DIRECTION ( 'NONE',  ( -0.000000000000000000, 0.1205366802553233113, 0.9927088740980539727 ) ) ;
#33915=CARTESIAN_POINT ( 'NONE',  ( -332.3517673607765914, -66.84097189748108292, 19.74220186498880736 ) ) ;
#33916=LINE ( 'NONE', #13698, #19725 ) ;
#33917=DIRECTION ( 'NONE',  ( 1.000000000000000000, -0.000000000000000000, 0.000000000000000000 ) ) ;
#33920=CARTESIAN_POINT ( 'NONE',  ( -336.3521761649654422, -66.84438072661991725, -16.67542351306652648 ) ) ;
#33921=VECTOR ( 'NONE', #17164, 1000.000000000000000 ) ;
#33922=AXIS2_PLACEMENT_3D ( 'NONE', #42831, #35200, #18416 ) ;
#33923=LINE ( 'NONE', #49714, #29396 ) ;
#33924=CARTESIAN_POINT ( 'NONE',  ( -339.1964088526558498, -63.50208336950359467, 0.4999999999999543698 ) ) ;
#33931=VECTOR ( 'NONE', #44037, 1000.000000000000114 ) ;
#33932=CARTESIAN_POINT ( 'NONE',  ( -332.3517673607765914, -77.59233547837267508, 37.15394033962009246 ) ) ;
#33933=CARTESIAN_POINT ( 'NONE',  ( -330.4913330509368166, -137.1341532842523918, 57.40522506028099770 ) ) ;
#33934=ORIENTED_EDGE ( 'NONE', *, *, #4419, .T. ) ;
#33941=CARTESIAN_POINT ( 'NONE',  ( -332.3517673607765914, -183.3224719910990643, -4.612141029301910500 ) ) ;
#33945=LINE ( 'NONE', #42096, #4150 ) ;
#33948=EDGE_LOOP ( 'NONE', ( #20309, #24627, #28822, #14717 ) ) ;
#33953=VERTEX_POINT ( 'NONE', #41558 ) ;
#33962=EDGE_CURVE ( 'NONE', #23668, #12667, #7336, .T. ) ;
#33963=VERTEX_POINT ( 'NONE', #25038 ) ;
#33965=EDGE_LOOP ( 'NONE', ( #10109, #19371, #43963, #44395, #401 ) ) ;
#33967=EDGE_CURVE ( 'NONE', #20840, #8243, #4805, .T. ) ;
#33971=DIRECTION ( 'NONE',  ( 1.000000000000000000, 0.000000000000000000, 0.000000000000000000 ) ) ;
#33973=EDGE_LOOP ( 'NONE', ( #13797, #32201, #29302, #29312 ) ) ;
#33974=FACE_BOUND ( 'NONE', #32256, .T. ) ;
#33981=CARTESIAN_POINT ( 'NONE',  ( -332.3517673607765914, -123.5000000000000284, 0.000000000000000000 ) ) ;
#33984=ORIENTED_EDGE ( 'NONE', *, *, #17724, .T. ) ;
#33986=FACE_OUTER_BOUND ( 'NONE', #9033, .T. ) ;
#33989=ADVANCED_FACE ( 'NONE', ( #37574 ), #21022, .T. ) ;
#33992=ORIENTED_EDGE ( 'NONE', *, *, #22952, .F. ) ;
#33997=AXIS2_PLACEMENT_3D ( 'NONE', #43844, #7844, #40668 ) ;
#33998=VECTOR ( 'NONE', #2574, 1000.000000000000000 ) ;
#34000=VECTOR ( 'NONE', #5956, 1000.000000000000000 ) ;
#34001=EDGE_CURVE ( 'NONE', #26732, #8616, #23284, .T. ) ;
#34008=DIRECTION ( 'NONE',  ( 1.043714542225393381E-14, 0.9350162426854107256, -0.3546048870425463906 ) ) ;
#34015=AXIS2_PLACEMENT_3D ( 'NONE', #23437, #19999, #23178 ) ;
#34016=CARTESIAN_POINT ( 'NONE',  ( -332.3517673607765914, -123.5000000000000284, 0.000000000000000000 ) ) ;
#34017=VERTEX_POINT ( 'NONE', #513 ) ;
#34018=VERTEX_POINT ( 'NONE', #789 ) ;
#34020=VERTEX_POINT ( 'NONE', #17613 ) ;
#34024=ADVANCED_FACE ( 'NONE', ( #4475 ), #37303, .F. ) ;
#34025=EDGE_CURVE ( 'NONE', #23542, #19699, #32499, .T. ) ;
#34027=CARTESIAN_POINT ( 'NONE',  ( -336.3521761649654422, -114.7679482383557144, 58.37307289257701370 ) ) ;
#34029=ADVANCED_FACE ( 'NONE', ( #33624 ), #25226, .T. ) ;
#34034=CARTESIAN_POINT ( 'NONE',  ( -336.3521761649654422, -65.82380048139334860, 12.53476669029061519 ) ) ;
#34041=EDGE_CURVE ( 'NONE', #7787, #22679, #40454, .T. ) ;
#34048=VERTEX_POINT ( 'NONE', #29936 ) ;
#34049=FACE_OUTER_BOUND ( 'NONE', #35808, .T. ) ;
#34056=CARTESIAN_POINT ( 'NONE',  ( -336.3521761649654422, -155.6724726690323450, 49.48329383994676078 ) ) ;
#34061=VECTOR ( 'NONE', #5089, 999.9999999999998863 ) ;
#34063=CARTESIAN_POINT ( 'NONE',  ( -339.1964088526558498, -75.22798428563942252, 33.92731199008440512 ) ) ;
#34064=ORIENTED_EDGE ( 'NONE', *, *, #8092, .F. ) ;
#34066=DIRECTION ( 'NONE',  ( 0.000000000000000000, 0.4647231720437631775, -0.8854560256532126861 ) ) ;
#34067=ORIENTED_EDGE ( 'NONE', *, *, #1981, .T. ) ;
#34074=VECTOR ( 'NONE', #33593, 999.9999999999998863 ) ;
#34076=EDGE_CURVE ( 'NONE', #30532, #50591, #41775, .T. ) ;
#34077=ADVANCED_FACE ( 'NONE', ( #30701 ), #45719, .F. ) ;
#34078=CARTESIAN_POINT ( 'NONE',  ( -332.3517673607765914, -123.5000000000000284, 0.000000000000000000 ) ) ;
#34080=ORIENTED_EDGE ( 'NONE', *, *, #44948, .T. ) ;
#34081=EDGE_LOOP ( 'NONE', ( #32955, #29901, #44613, #44478 ) ) ;
#34082=VERTEX_POINT ( 'NONE', #41776 ) ;
#34083=LINE ( 'NONE', #50134, #20010 ) ;
#34086=DIRECTION ( 'NONE',  ( 1.000000000000000000, -8.654812430365565511E-17, 1.050884489711754678E-17 ) ) ;
#34089=CARTESIAN_POINT ( 'NONE',  ( -339.1964088526558498, -150.4759391377560576, -52.47426709956116042 ) ) ;
#34091=VECTOR ( 'NONE', #2379, 1000.000000000000000 ) ;
#34099=ADVANCED_FACE ( 'NONE', ( #9984 ), #26767, .F. ) ;
#34105=VERTEX_POINT ( 'NONE', #39553 ) ;
#34110=CARTESIAN_POINT ( 'NONE',  ( -339.1964088526558498, -73.83865025250327108, -33.67120938215323633 ) ) ;
#34113=AXIS2_PLACEMENT_3D ( 'NONE', #23571, #39586, #28289 ) ;
#34116=DIRECTION ( 'NONE',  ( -0.000000000000000000, -0.8854560256532062468, 0.4647231720437755564 ) ) ;
#34119=LINE ( 'NONE', #9435, #48986 ) ;
#34120=DIRECTION ( 'NONE',  ( -0.000000000000000000, 0.4647231720437789981, 0.8854560256532044704 ) ) ;
#34121=ORIENTED_EDGE ( 'NONE', *, *, #21491, .T. ) ;
#34122=FACE_OUTER_BOUND ( 'NONE', #1689, .T. ) ;
#34127=AXIS2_PLACEMENT_3D ( 'NONE', #8247, #32417, #25320 ) ;
#34129=CARTESIAN_POINT ( 'NONE',  ( -336.3521761649654422, -173.5513585866778214, -31.34948880313881503 ) ) ;
#34135=AXIS2_PLACEMENT_3D ( 'NONE', #34016, #17744, #38481 ) ;
#34139=DIRECTION ( 'NONE',  ( 0.000000000000000000, 0.000000000000000000, -1.000000000000000000 ) ) ;
#34142=EDGE_CURVE ( 'NONE', #16904, #1525, #22306, .T. ) ;
#34143=DIRECTION ( 'NONE',  ( 0.000000000000000000, 0.1205366802553095307, -0.9927088740980556381 ) ) ;
#34144=EDGE_LOOP ( 'NONE', ( #45957, #15299, #29605, #3265 ) ) ;
#34149=ORIENTED_EDGE ( 'NONE', *, *, #50526, .F. ) ;
#34151=VECTOR ( 'NONE', #42915, 1000.000000000000000 ) ;
#34159=CIRCLE ( 'NONE', #11495, 60.00000000000000000 ) ;
#34160=EDGE_CURVE ( 'NONE', #30471, #17498, #22052, .T. ) ;
#34162=LINE ( 'NONE', #30220, #4644 ) ;
#34163=VECTOR ( 'NONE', #12389, 1000.000000000000000 ) ;
#34164=ORIENTED_EDGE ( 'NONE', *, *, #23749, .F. ) ;
#34169=LINE ( 'NONE', #22333, #43402 ) ;
#34170=FACE_OUTER_BOUND ( 'NONE', #39713, .T. ) ;
#34171=ORIENTED_EDGE ( 'NONE', *, *, #11651, .F. ) ;
#34177=PLANE ( 'NONE',  #17329 ) ;
#34183=FACE_BOUND ( 'NONE', #2119, .T. ) ;
#34186=LINE ( 'NONE', #42838, #51716 ) ;
#34192=CARTESIAN_POINT ( 'NONE',  ( -339.1964088526558498, -66.33409060400650503, 14.60509510167813474 ) ) ;
#34197=DIRECTION ( 'NONE',  ( 0.000000000000000000, -0.9927088740980544168, -0.1205366802553199113 ) ) ;
#34200=VECTOR ( 'NONE', #51543, 1000.000000000000000 ) ;
#34203=DIRECTION ( 'NONE',  ( 0.000000000000000000, 0.2393156642875482742, -0.9709418174260544543 ) ) ;
#34205=ORIENTED_EDGE ( 'NONE', *, *, #11407, .T. ) ;
#34206=ADVANCED_FACE ( 'NONE', ( #38335 ), #5794, .F. ) ;
#34209=EDGE_CURVE ( 'NONE', #11713, #27333, #18382, .T. ) ;
#34211=CARTESIAN_POINT ( 'NONE',  ( -330.4913330509368166, -182.0095552316576573, -7.608018572112656308 ) ) ;
#34215=ADVANCED_FACE ( 'NONE', ( #19593 ), #50445, .F. ) ;
#34217=PLANE ( 'NONE',  #40144 ) ;
#34222=CARTESIAN_POINT ( 'NONE',  ( -180.0000000000000568, -123.5000000000000284, 15.24495751795539000 ) ) ;
#34223=VECTOR ( 'NONE', #22988, 1000.000000000000000 ) ;
#34224=DIRECTION ( 'NONE',  ( -0.000000000000000000, -0.8229838658936536877, 0.5680647467311596976 ) ) ;
#34226=VECTOR ( 'NONE', #51760, 1000.000000000000000 ) ;
#34229=ORIENTED_EDGE ( 'NONE', *, *, #43483, .F. ) ;
#34232=ORIENTED_EDGE ( 'NONE', *, *, #22387, .T. ) ;
#34233=DIRECTION ( 'NONE',  ( -0.000000000000000000, 0.9709418174260553425, 0.2393156642875449158 ) ) ;
#34235=LINE ( 'NONE', #15051, #48393 ) ;
#34236=VECTOR ( 'NONE', #38718, 1000.000000000000000 ) ;
#34239=PLANE ( 'NONE',  #1507 ) ;
#34240=ORIENTED_EDGE ( 'NONE', *, *, #40350, .T. ) ;
#34242=ORIENTED_EDGE ( 'NONE', *, *, #39785, .F. ) ;
#34243=FACE_BOUND ( 'NONE', #35571, .T. ) ;
#34246=ORIENTED_EDGE ( 'NONE', *, *, #7819, .F. ) ;
#34247=CARTESIAN_POINT ( 'NONE',  ( -339.1964088526558498, -64.50000000000000000, 0.4999999999999543698 ) ) ;
#34250=CARTESIAN_POINT ( 'NONE',  ( -336.3521761649654422, -78.25545813661345562, 37.90245108779119931 ) ) ;
#34252=DIRECTION ( 'NONE',  ( 0.000000000000000000, 0.8854560256532110207, 0.4647231720437664526 ) ) ;
#34254=CARTESIAN_POINT ( 'NONE',  ( -330.4913330509368166, -180.9052250602807703, 13.63415328425337236 ) ) ;
#34258=FACE_OUTER_BOUND ( 'NONE', #47545, .T. ) ;
#34259=EDGE_LOOP ( 'NONE', ( #10161, #2202, #31026, #14841 ) ) ;
#34261=VECTOR ( 'NONE', #28784, 1000.000000000000114 ) ;
#34265=DIRECTION ( 'NONE',  ( 0.000000000000000000, -1.000000000000000000, 1.047444401652940007E-14 ) ) ;
#34269=CARTESIAN_POINT ( 'NONE',  ( -332.3517673607765914, -104.1045282520827300, -55.74477592174792306 ) ) ;
#34278=CARTESIAN_POINT ( 'NONE',  ( -330.4913330509368166, -109.8658467157464571, 57.40522506028071348 ) ) ;
#34281=DIRECTION ( 'NONE',  ( 1.043714542225393381E-14, -0.1205366802553233113, -0.9927088740980539727 ) ) ;
#34282=FACE_OUTER_BOUND ( 'NONE', #8591, .T. ) ;
#34284=VERTEX_POINT ( 'NONE', #44026 ) ;
#34287=DIRECTION ( 'NONE',  ( -1.000000000000000000, 0.000000000000000000, 0.000000000000000000 ) ) ;
#34292=DIRECTION ( 'NONE',  ( -0.000000000000000000, 0.9709418174260553425, 0.2393156642875449158 ) ) ;
#34303=ORIENTED_EDGE ( 'NONE', *, *, #33665, .T. ) ;
#34305=ORIENTED_EDGE ( 'NONE', *, *, #38644, .T. ) ;
#34307=ORIENTED_EDGE ( 'NONE', *, *, #45261, .F. ) ;
#34308=PLANE ( 'NONE',  #15370 ) ;
#34310=CARTESIAN_POINT ( 'NONE',  ( -305.0000000000000568, -79.68838513426354098, -40.99441916720346057 ) ) ;
#34318=DIRECTION ( 'NONE',  ( -0.000000000000000000, -0.1205366802553268363, -0.9927088740980534176 ) ) ;
#34319=EDGE_CURVE ( 'NONE', #27371, #24196, #15750, .T. ) ;
#34322=EDGE_LOOP ( 'NONE', ( #13956, #45498, #7726, #26582 ) ) ;
#34324=CARTESIAN_POINT ( 'NONE',  ( -339.1964088526558498, -172.3400804610910200, 33.10432812419180948 ) ) ;
#34325=ORIENTED_EDGE ( 'NONE', *, *, #22174, .F. ) ;
#34326=ORIENTED_EDGE ( 'NONE', *, *, #2238, .F. ) ;
#34333=DIRECTION ( 'NONE',  ( 0.000000000000000000, 0.000000000000000000, 1.000000000000000000 ) ) ;
#34334=DIRECTION ( 'NONE',  ( 0.000000000000000000, -6.383782391594650107E-14, -1.000000000000000000 ) ) ;
#34339=FACE_OUTER_BOUND ( 'NONE', #38928, .T. ) ;
#34342=ORIENTED_EDGE ( 'NONE', *, *, #3741, .F. ) ;
#34343=ADVANCED_FACE ( 'NONE', ( #1959 ), #9078, .F. ) ;
#34344=VERTEX_POINT ( 'NONE', #45855 ) ;
#34347=VECTOR ( 'NONE', #8855, 1000.000000000000000 ) ;
#34350=DIRECTION ( 'NONE',  ( -1.000000000000000000, 0.000000000000000000, 0.000000000000000000 ) ) ;
#34351=LINE ( 'NONE', #30146, #33080 ) ;
#34357=DIRECTION ( 'NONE',  ( 1.000000000000000000, -0.000000000000000000, -0.000000000000000000 ) ) ;
#34359=ORIENTED_EDGE ( 'NONE', *, *, #41431, .F. ) ;
#34361=ORIENTED_EDGE ( 'NONE', *, *, #23749, .T. ) ;
#34366=ORIENTED_EDGE ( 'NONE', *, *, #30117, .F. ) ;
#34367=FACE_OUTER_BOUND ( 'NONE', #46770, .T. ) ;
#34368=ORIENTED_EDGE ( 'NONE', *, *, #3903, .T. ) ;
#34371=FACE_OUTER_BOUND ( 'NONE', #18003, .T. ) ;
#34374=DIRECTION ( 'NONE',  ( 0.000000000000000000, 0.000000000000000000, 1.000000000000000000 ) ) ;
#34375=VERTEX_POINT ( 'NONE', #49802 ) ;
#34377=CIRCLE ( 'NONE', #50226, 60.00000000000000000 ) ;
#34378=DIRECTION ( 'NONE',  ( -1.000000000000000000, 0.000000000000000000, 0.000000000000000000 ) ) ;
#34379=EDGE_CURVE ( 'NONE', #20132, #50151, #41123, .T. ) ;
#34385=DIRECTION ( 'NONE',  ( -1.000000000000000000, 0.000000000000000000, 0.000000000000000000 ) ) ;
#34389=ORIENTED_EDGE ( 'NONE', *, *, #40074, .F. ) ;
#34390=CARTESIAN_POINT ( 'NONE',  ( -339.1964088526558498, -79.66942718702553350, -39.49849221029258928 ) ) ;
#34391=DIRECTION ( 'NONE',  ( 0.000000000000000000, 0.000000000000000000, 1.000000000000000000 ) ) ;
#34396=DIRECTION ( 'NONE',  ( 0.000000000000000000, 0.6631226582407964143, 0.7485107481710999711 ) ) ;
#34401=CARTESIAN_POINT ( 'NONE',  ( -336.3521761649654422, -182.5000000000000568, 2.632288850093980503 ) ) ;
#34408=VECTOR ( 'NONE', #44426, 1000.000000000000000 ) ;
#34410=DIRECTION ( 'NONE',  ( 1.000000000000000000, -0.000000000000000000, -0.000000000000000000 ) ) ;
#34412=DIRECTION ( 'NONE',  ( -0.000000000000000000, -0.8854560256532062468, 0.4647231720437755564 ) ) ;
#34413=VERTEX_POINT ( 'NONE', #25605 ) ;
#34418=ORIENTED_EDGE ( 'NONE', *, *, #49191, .T. ) ;
#34419=LINE ( 'NONE', #10247, #6286 ) ;
#34436=DIRECTION ( 'NONE',  ( 0.000000000000000000, 0.8229838658936634577, 0.5680647467311457088 ) ) ;
#34437=DIRECTION ( 'NONE',  ( -1.000000000000000000, 0.000000000000000000, -0.000000000000000000 ) ) ;
#34438=VERTEX_POINT ( 'NONE', #12993 ) ;
#34442=LINE ( 'NONE', #33666, #39695 ) ;
#34452=CARTESIAN_POINT ( 'NONE',  ( -339.1964088526558498, -116.8846903019852164, -58.63009191191289915 ) ) ;
#34453=EDGE_CURVE ( 'NONE', #34970, #17341, #37434, .T. ) ;
#34455=LINE ( 'NONE', #30771, #33759 ) ;
#34456=ORIENTED_EDGE ( 'NONE', *, *, #45162, .F. ) ;
#34458=AXIS2_PLACEMENT_3D ( 'NONE', #1051, #13152, #28640 ) ;
#34464=CARTESIAN_POINT ( 'NONE',  ( -332.3517673607765914, -64.61288906875131488, 4.498567634385603142 ) ) ;
#34465=ADVANCED_FACE ( 'NONE', ( #17494 ), #25873, .F. ) ;
#34466=CARTESIAN_POINT ( 'NONE',  ( -336.3521761649654422, -76.43926241122620979, -35.68215131113738181 ) ) ;
#34468=VERTEX_POINT ( 'NONE', #42148 ) ;
#34470=DIRECTION ( 'NONE',  ( -1.000000000000000000, -0.000000000000000000, -0.000000000000000000 ) ) ;
#34471=LINE ( 'NONE', #26841, #45980 ) ;
#34474=VECTOR ( 'NONE', #13791, 1000.000000000000000 ) ;
#34476=ORIENTED_EDGE ( 'NONE', *, *, #30958, .T. ) ;
#34477=FACE_OUTER_BOUND ( 'NONE', #7595, .T. ) ;
#34482=ADVANCED_FACE ( 'NONE', ( #6173 ), #37954, .F. ) ;
#34492=FACE_BOUND ( 'NONE', #9532, .T. ) ;
#34493=CARTESIAN_POINT ( 'NONE',  ( -339.1964088526558498, -167.9936954712156592, -38.74998146212110584 ) ) ;
#34494=VECTOR ( 'NONE', #12063, 1000.000000000000000 ) ;
#34496=DIRECTION ( 'NONE',  ( -0.000000000000000000, 0.8854560256532093554, -0.4647231720437695057 ) ) ;
#34497=ORIENTED_EDGE ( 'NONE', *, *, #46571, .T. ) ;
#34508=DIRECTION ( 'NONE',  ( 1.000000000000000000, 0.000000000000000000, -0.000000000000000000 ) ) ;
#34509=EDGE_CURVE ( 'NONE', #4643, #8311, #42414, .T. ) ;
#34511=LINE ( 'NONE', #10346, #2693 ) ;
#34519=LINE ( 'NONE', #51110, #40939 ) ;
#34522=CARTESIAN_POINT ( 'NONE',  ( -339.1964088526558498, -116.7644047441736035, -59.62073260661671981 ) ) ;
#34523=CARTESIAN_POINT ( 'NONE',  ( -336.3521761649654422, -177.7325358280884586, 23.38292116578760726 ) ) ;
#34526=EDGE_LOOP ( 'NONE', ( #45816, #46691, #42442, #3812 ) ) ;
#34530=FACE_OUTER_BOUND ( 'NONE', #10311, .T. ) ;
#34533=ORIENTED_EDGE ( 'NONE', *, *, #51573, .T. ) ;
#34540=DIRECTION ( 'NONE',  ( -1.000000000000000000, 0.000000000000000000, -0.000000000000000000 ) ) ;
#34543=LINE ( 'NONE', #49825, #40081 ) ;
#34544=DIRECTION ( 'NONE',  ( 0.000000000000000000, 0.000000000000000000, 1.000000000000000000 ) ) ;
#34549=EDGE_CURVE ( 'NONE', #42116, #19264, #19293, .T. ) ;
#34550=EDGE_LOOP ( 'NONE', ( #17553, #50901, #13038, #6237 ) ) ;
#34553=DIRECTION ( 'NONE',  ( -1.000000000000000000, 0.000000000000000000, 0.000000000000000000 ) ) ;
#34562=VECTOR ( 'NONE', #12657, 999.9999999999998863 ) ;
#34563=DIRECTION ( 'NONE',  ( 1.043714542225393223E-14, 0.9709418174260493473, -0.2393156642875685913 ) ) ;
#34569=VERTEX_POINT ( 'NONE', #23232 ) ;
#34571=DIRECTION ( 'NONE',  ( 1.000000000000000000, -0.000000000000000000, 0.000000000000000000 ) ) ;
#34576=CARTESIAN_POINT ( 'NONE',  ( -332.3517673607765914, -73.21199843436539823, 32.72792230702598459 ) ) ;
#34579=LINE ( 'NONE', #47461, #898 ) ;
#34581=ORIENTED_EDGE ( 'NONE', *, *, #23081, .T. ) ;
#34582=VERTEX_POINT ( 'NONE', #38477 ) ;
#34584=DIRECTION ( 'NONE',  ( 0.000000000000000000, -0.8229838658936613482, -0.5680647467311485954 ) ) ;
#34588=CARTESIAN_POINT ( 'NONE',  ( -336.3521761649654422, -140.1754235130667610, -56.65561927338005432 ) ) ;
#34590=ORIENTED_EDGE ( 'NONE', *, *, #41611, .T. ) ;
#34596=CARTESIAN_POINT ( 'NONE',  ( -336.3521761649654422, -73.44864141332200802, 31.34948880313848107 ) ) ;
#34599=ORIENTED_EDGE ( 'NONE', *, *, #12917, .F. ) ;
#34602=CARTESIAN_POINT ( 'NONE',  ( -336.3521761649654422, -135.0638248728647852, 57.91551518289418254 ) ) ;
#34605=DIRECTION ( 'NONE',  ( 0.000000000000000000, 0.000000000000000000, -1.000000000000000000 ) ) ;
#34606=DIRECTION ( 'NONE',  ( -1.000000000000000000, -0.000000000000000000, -0.000000000000000000 ) ) ;
#34608=ORIENTED_EDGE ( 'NONE', *, *, #49412, .T. ) ;
#34620=ADVANCED_FACE ( 'NONE', ( #12142 ), #48435, .T. ) ;
#34623=DIRECTION ( 'NONE',  ( 1.000000000000000000, 0.000000000000000000, -0.000000000000000000 ) ) ;
#34625=ADVANCED_FACE ( 'NONE', ( #39736 ), #16115, .F. ) ;
#34627=CARTESIAN_POINT ( 'NONE',  ( -336.3521761649654422, -100.1170788342122080, 54.23253582808833073 ) ) ;
#34633=CARTESIAN_POINT ( 'NONE',  ( -330.4913330509368166, -180.9052250602809693, -13.63415328425256945 ) ) ;
#34636=EDGE_LOOP ( 'NONE', ( #48502, #14920, #26508, #15272 ) ) ;
#34649=DIRECTION ( 'NONE',  ( 0.000000000000000000, -6.245004513516505540E-15, -1.000000000000000000 ) ) ;
#34651=EDGE_CURVE ( 'NONE', #3375, #34970, #19523, .T. ) ;
#34654=ORIENTED_EDGE ( 'NONE', *, *, #19407, .T. ) ;
#34656=EDGE_CURVE ( 'NONE', #29379, #8048, #39496, .T. ) ;
#34659=AXIS2_PLACEMENT_3D ( 'NONE', #24311, #15660, #47721 ) ;
#34662=CARTESIAN_POINT ( 'NONE',  ( -332.3517673607765914, -169.4076645216271402, -37.15394033962039089 ) ) ;
#34673=PLANE ( 'NONE',  #22452 ) ;
#34678=ORIENTED_EDGE ( 'NONE', *, *, #21985, .T. ) ;
#34680=DIRECTION ( 'NONE',  ( 0.000000000000000000, -0.9350162426854107256, 0.3546048870425463906 ) ) ;
#34681=EDGE_CURVE ( 'NONE', #23911, #21654, #27676, .T. ) ;
#34682=ORIENTED_EDGE ( 'NONE', *, *, #6024, .T. ) ;
#34686=DIRECTION ( 'NONE',  ( 1.000000000000000000, -2.086444717177606589E-17, -8.465038975556385201E-17 ) ) ;
#34693=ADVANCED_FACE ( 'NONE', ( #23730 ), #24258, .F. ) ;
#34701=ORIENTED_EDGE ( 'NONE', *, *, #35601, .F. ) ;
#34702=EDGE_CURVE ( 'NONE', #19264, #7764, #40006, .T. ) ;
#34703=LINE ( 'NONE', #26817, #2735 ) ;
#34711=CARTESIAN_POINT ( 'NONE',  ( -336.3521761649654422, -182.5000000000000568, 2.632288850093980503 ) ) ;
#34722=LINE ( 'NONE', #26585, #798 ) ;
#34723=CARTESIAN_POINT ( 'NONE',  ( -336.3521761649654422, -170.5607375887735770, 35.68215131113770155 ) ) ;
#34727=CARTESIAN_POINT ( 'NONE',  ( -336.3521761649654422, -68.38646289696045244, -23.71704087764494062 ) ) ;
#34730=ORIENTED_EDGE ( 'NONE', *, *, #3949, .T. ) ;
#34731=CARTESIAN_POINT ( 'NONE',  ( -339.1964088526558498, -101.7569374291128526, -55.92172413327835301 ) ) ;
#34734=VERTEX_POINT ( 'NONE', #36594 ) ;
#34741=VECTOR ( 'NONE', #1209, 999.9999999999998863 ) ;
#34742=CARTESIAN_POINT ( 'NONE',  ( 0.000000000000000000, -178.6659583184396354, -20.92168833550928042 ) ) ;
#34743=VECTOR ( 'NONE', #44122, 1000.000000000000000 ) ;
#34745=CARTESIAN_POINT ( 'NONE',  ( -305.0000000000000568, -123.5000000000000284, 0.000000000000000000 ) ) ;
#34749=ORIENTED_EDGE ( 'NONE', *, *, #31389, .F. ) ;
#34753=DIRECTION ( 'NONE',  ( -0.000000000000000000, 0.3546048870425331789, -0.9350162426854158326 ) ) ;
#34756=DIRECTION ( 'NONE',  ( -1.000000000000000000, -0.000000000000000000, 0.000000000000000000 ) ) ;
#34757=LINE ( 'NONE', #6668, #15663 ) ;
#34758=CIRCLE ( 'NONE', #37314, 60.00000000000000000 ) ;
#34764=ORIENTED_EDGE ( 'NONE', *, *, #7972, .F. ) ;
#34768=ORIENTED_EDGE ( 'NONE', *, *, #8602, .F. ) ;
#34777=CARTESIAN_POINT ( 'NONE',  ( -339.1964088526558498, -64.86990808808717190, -6.615309698015097162 ) ) ;
#34781=ORIENTED_EDGE ( 'NONE', *, *, #15904, .F. ) ;
#34782=DIRECTION ( 'NONE',  ( -0.000000000000000000, -0.7485107481711046340, -0.6631226582407911962 ) ) ;
#34786=DIRECTION ( 'NONE',  ( 1.000000000000000000, 0.000000000000000000, 0.000000000000000000 ) ) ;
#34791=VERTEX_POINT ( 'NONE', #9523 ) ;
#34793=LINE ( 'NONE', #46922, #18940 ) ;
#34795=LINE ( 'NONE', #7217, #45158 ) ;
#34801=DIRECTION ( 'NONE',  ( -0.000000000000000000, 0.7485107481711089639, 0.6631226582407863113 ) ) ;
#34802=ORIENTED_EDGE ( 'NONE', *, *, #49157, .T. ) ;
#34804=VECTOR ( 'NONE', #48725, 1000.000000000000000 ) ;
#34805=LINE ( 'NONE', #17770, #15259 ) ;
#34806=ORIENTED_EDGE ( 'NONE', *, *, #21477, .F. ) ;
#34813=VECTOR ( 'NONE', #31210, 1000.000000000000000 ) ;
#34815=VERTEX_POINT ( 'NONE', #25046 ) ;
#34817=CARTESIAN_POINT ( 'NONE',  ( -339.1964088526558498, -67.22367097967892846, 20.80804632820117916 ) ) ;
#34824=ORIENTED_EDGE ( 'NONE', *, *, #41683, .T. ) ;
#34828=EDGE_LOOP ( 'NONE', ( #48146, #6357, #28379, #26648 ) ) ;
#34829=DIRECTION ( 'NONE',  ( 0.000000000000000000, -0.9709418174260502354, 0.2393156642875652051 ) ) ;
#34834=DIRECTION ( 'NONE',  ( 1.000000000000000000, 0.000000000000000000, 0.000000000000000000 ) ) ;
#34835=CARTESIAN_POINT ( 'NONE',  ( -305.0000000000000568, -75.06648993880729392, -35.41461708323759439 ) ) ;
#34847=DIRECTION ( 'NONE',  ( 1.000000000000000000, 6.525800561034990492E-17, 5.781354811211851654E-17 ) ) ;
#34848=LINE ( 'NONE', #47225, #26397 ) ;
#34850=VECTOR ( 'NONE', #15844, 1000.000000000000000 ) ;
#34858=VECTOR ( 'NONE', #34357, 1000.000000000000000 ) ;
#34867=VECTOR ( 'NONE', #50587, 999.9999999999998863 ) ;
#34872=VERTEX_POINT ( 'NONE', #17431 ) ;
#34873=CARTESIAN_POINT ( 'NONE',  ( -339.1964088526558498, -150.4759391377552618, 52.47426709956155122 ) ) ;
#34875=FACE_OUTER_BOUND ( 'NONE', #46094, .T. ) ;
#34880=CARTESIAN_POINT ( 'NONE',  ( -339.1964088526558498, -178.4886558749184076, -21.38919645685194837 ) ) ;
#34883=DIRECTION ( 'NONE',  ( -0.000000000000000000, -0.9927088740980548609, -0.1205366802553164696 ) ) ;
#34898=ADVANCED_FACE ( 'NONE', ( #12929 ), #13721, .T. ) ;
#34904=AXIS2_PLACEMENT_3D ( 'NONE', #50335, #8882, #49097 ) ;
#34905=FACE_OUTER_BOUND ( 'NONE', #9223, .T. ) ;
#34910=LINE ( 'NONE', #3125, #49440 ) ;
#34917=VECTOR ( 'NONE', #43799, 1000.000000000000000 ) ;
#34921=CARTESIAN_POINT ( 'NONE',  ( -490.0000000000001137, -78.50000000000002842, 0.000000000000000000 ) ) ;
#34922=ORIENTED_EDGE ( 'NONE', *, *, #10032, .F. ) ;
#34925=VERTEX_POINT ( 'NONE', #6360 ) ;
#34936=FACE_OUTER_BOUND ( 'NONE', #37019, .T. ) ;
#34939=LINE ( 'NONE', #38108, #4746 ) ;
#34945=AXIS2_PLACEMENT_3D ( 'NONE', #42108, #45303, #5613 ) ;
#34947=DIRECTION ( 'NONE',  ( -0.000000000000000000, 0.000000000000000000, -1.000000000000000000 ) ) ;
#34953=ADVANCED_FACE ( 'NONE', ( #38916 ), #34217, .T. ) ;
#34954=CARTESIAN_POINT ( 'NONE',  ( -332.3517673607765914, -174.9833430614318388, 28.86398714850502856 ) ) ;
#34955=EDGE_CURVE ( 'NONE', #39674, #8221, #22900, .T. ) ;
#34958=EDGE_CURVE ( 'NONE', #44807, #39299, #51916, .T. ) ;
#34964=CARTESIAN_POINT ( 'NONE',  ( -339.1964088526558498, -84.00150778970767362, -43.83057281297470098 ) ) ;
#34965=EDGE_CURVE ( 'NONE', #27624, #30532, #46566, .T. ) ;
#34966=LINE ( 'NONE', #38396, #2648 ) ;
#34969=CIRCLE ( 'NONE', #4787, 60.00000000000000000 ) ;
#34970=VERTEX_POINT ( 'NONE', #39183 ) ;
#34971=EDGE_CURVE ( 'NONE', #6765, #27048, #50767, .T. ) ;
#34973=ADVANCED_FACE ( 'NONE', ( #22129 ), #30268, .F. ) ;
#34976=VECTOR ( 'NONE', #42372, 999.9999999999998863 ) ;
#34977=EDGE_LOOP ( 'NONE', ( #48554, #9094, #14004, #40002 ) ) ;
#34978=EDGE_CURVE ( 'NONE', #7704, #44807, #46313, .T. ) ;
#34979=VECTOR ( 'NONE', #12320, 1000.000000000000114 ) ;
#34980=ORIENTED_EDGE ( 'NONE', *, *, #428, .T. ) ;
#34981=LINE ( 'NONE', #34464, #25047 ) ;
#34987=ORIENTED_EDGE ( 'NONE', *, *, #19525, .F. ) ;
#34989=VECTOR ( 'NONE', #9228, 1000.000000000000000 ) ;
#34993=FACE_OUTER_BOUND ( 'NONE', #19359, .T. ) ;
#34996=ORIENTED_EDGE ( 'NONE', *, *, #44320, .T. ) ;
#35002=EDGE_CURVE ( 'NONE', #45545, #4141, #34981, .T. ) ;
#35004=EDGE_CURVE ( 'NONE', #27368, #18178, #42092, .T. ) ;
#35009=LINE ( 'NONE', #30036, #687 ) ;
#35015=FACE_BOUND ( 'NONE', #31351, .T. ) ;
#35016=DIRECTION ( 'NONE',  ( 1.043714542225393539E-14, -0.6631226582407911962, 0.7485107481711046340 ) ) ;
#35019=ORIENTED_EDGE ( 'NONE', *, *, #37052, .T. ) ;
#35025=AXIS2_PLACEMENT_3D ( 'NONE', #7541, #23562, #23820 ) ;
#35028=CARTESIAN_POINT ( 'NONE',  ( -490.0000000000001137, -168.5000000000000284, 0.000000000000000000 ) ) ;
#35031=AXIS2_PLACEMENT_3D ( 'NONE', #44713, #32623, #48667 ) ;
#35036=EDGE_CURVE ( 'NONE', #36520, #3787, #32317, .T. ) ;
#35039=DIRECTION ( 'NONE',  ( 0.000000000000000000, -0.9709418174260502354, 0.2393156642875652051 ) ) ;
#35044=ORIENTED_EDGE ( 'NONE', *, *, #5314, .F. ) ;
#35046=CIRCLE ( 'NONE', #48497, 60.00000000000000000 ) ;
#35051=DIRECTION ( 'NONE',  ( -0.000000000000000000, 0.1205366802553199113, -0.9927088740980544168 ) ) ;
#35055=CARTESIAN_POINT ( 'NONE',  ( -339.1964088526558498, -84.00150778970699150, 43.83057281297409702 ) ) ;
#35056=EDGE_LOOP ( 'NONE', ( #34205, #41105, #15008, #17049 ) ) ;
#35063=LINE ( 'NONE', #47407, #30780 ) ;
#35067=ORIENTED_EDGE ( 'NONE', *, *, #16665, .T. ) ;
#35075=FACE_OUTER_BOUND ( 'NONE', #32602, .T. ) ;
#35085=ORIENTED_EDGE ( 'NONE', *, *, #42692, .T. ) ;
#35087=CARTESIAN_POINT ( 'NONE',  ( -339.1964088526558498, -84.75001853787875916, -44.49369547121548862 ) ) ;
#35094=DIRECTION ( 'NONE',  ( 1.000000000000000000, -1.050884489711724171E-17, -8.654812430365567976E-17 ) ) ;
#35099=ORIENTED_EDGE ( 'NONE', *, *, #43846, .T. ) ;
#35103=DIRECTION ( 'NONE',  ( 0.000000000000000000, -0.2393156642875652051, -0.9709418174260502354 ) ) ;
#35113=PLANE ( 'NONE',  #44371 ) ;
#35114=CARTESIAN_POINT ( 'NONE',  ( -336.3521761649654422, -160.6539403396202772, 45.90766452162722544 ) ) ;
#35115=VECTOR ( 'NONE', #29767, 1000.000000000000000 ) ;
#35117=ADVANCED_FACE ( 'NONE', ( #23920 ), #23662, .F. ) ;
#35123=EDGE_CURVE ( 'NONE', #24837, #43547, #27347, .T. ) ;
#35127=ORIENTED_EDGE ( 'NONE', *, *, #38154, .T. ) ;
#35129=ORIENTED_EDGE ( 'NONE', *, *, #14388, .T. ) ;
#35139=ORIENTED_EDGE ( 'NONE', *, *, #25886, .T. ) ;
#35140=PLANE ( 'NONE',  #191 ) ;
#35150=DIRECTION ( 'NONE',  ( 0.000000000000000000, -0.9350162426854121689, 0.3546048870425426158 ) ) ;
#35153=ORIENTED_EDGE ( 'NONE', *, *, #24704, .T. ) ;
#35156=VECTOR ( 'NONE', #5520, 1000.000000000000000 ) ;
#35160=DIRECTION ( 'NONE',  ( 0.000000000000000000, 0.6631226582407885317, -0.7485107481711069655 ) ) ;
#35162=VECTOR ( 'NONE', #16153, 1000.000000000000000 ) ;
#35166=ORIENTED_EDGE ( 'NONE', *, *, #1457, .F. ) ;
#35168=DIRECTION ( 'NONE',  ( 0.000000000000000000, 0.2393156642875582940, 0.9709418174260519008 ) ) ;
#35172=DIRECTION ( 'NONE',  ( 1.000000000000000000, 0.000000000000000000, 0.000000000000000000 ) ) ;
#35173=ORIENTED_EDGE ( 'NONE', *, *, #25595, .T. ) ;
#35174=CARTESIAN_POINT ( 'NONE',  ( -330.4913330509368166, -64.99044476834235695, 7.608018572112246858 ) ) ;
#35175=EDGE_CURVE ( 'NONE', #38308, #10671, #3249, .T. ) ;
#35181=EDGE_LOOP ( 'NONE', ( #23440, #34608, #49104, #9726 ) ) ;
#35185=CARTESIAN_POINT ( 'NONE',  ( -305.0000000000000568, -67.99860710409808462, -22.79463504017392950 ) ) ;
#35186=AXIS2_PLACEMENT_3D ( 'NONE', #398, #26068, #12228 ) ;
#35188=EDGE_CURVE ( 'NONE', #14029, #2008, #15, .T. ) ;
#35189=EDGE_CURVE ( 'NONE', #49231, #49368, #11311, .T. ) ;
#35190=DIRECTION ( 'NONE',  ( -1.000000000000000000, 0.000000000000000000, -0.000000000000000000 ) ) ;
#35196=ORIENTED_EDGE ( 'NONE', *, *, #19015, .T. ) ;
#35198=CARTESIAN_POINT ( 'NONE',  ( -332.3517673607765914, -120.8677111499054320, 59.00000000000000000 ) ) ;
#35200=DIRECTION ( 'NONE',  ( 0.000000000000000000, 0.8229838658936536877, -0.5680647467311596976 ) ) ;
#35202=DIRECTION ( 'NONE',  ( -1.000000000000000000, -0.000000000000000000, 0.000000000000000000 ) ) ;
#35204=ORIENTED_EDGE ( 'NONE', *, *, #5580, .F. ) ;
#35214=LINE ( 'NONE', #11287, #49171 ) ;
#35219=ORIENTED_EDGE ( 'NONE', *, *, #15003, .F. ) ;
#35222=DIRECTION ( 'NONE',  ( -0.000000000000000000, -0.2393156642875482742, 0.9709418174260544543 ) ) ;
#35225=DIRECTION ( 'NONE',  ( 1.000000000000000000, -0.000000000000000000, -0.000000000000000000 ) ) ;
#35226=DIRECTION ( 'NONE',  ( -1.000000000000000000, -0.000000000000000000, 0.000000000000000000 ) ) ;
#35230=ORIENTED_EDGE ( 'NONE', *, *, #8282, .T. ) ;
#35231=ORIENTED_EDGE ( 'NONE', *, *, #9138, .T. ) ;
#35234=DIRECTION ( 'NONE',  ( -0.000000000000000000, 0.8854560256532157947, 0.4647231720437573488 ) ) ;
#35237=AXIS2_PLACEMENT_3D ( 'NONE', #7176, #26877, #30312 ) ;
#35241=FACE_OUTER_BOUND ( 'NONE', #11054, .T. ) ;
#35249=EDGE_CURVE ( 'NONE', #37592, #26366, #32610, .T. ) ;
#35256=DIRECTION ( 'NONE',  ( 1.000000000000000000, 0.000000000000000000, 0.000000000000000000 ) ) ;
#35265=ORIENTED_EDGE ( 'NONE', *, *, #681, .F. ) ;
#35266=FACE_BOUND ( 'NONE', #1475, .T. ) ;
#35267=EDGE_CURVE ( 'NONE', #22193, #40543, #12876, .T. ) ;
#35270=ORIENTED_EDGE ( 'NONE', *, *, #39866, .T. ) ;
#35282=CIRCLE ( 'NONE', #9302, 60.00000000000000000 ) ;
#35284=CARTESIAN_POINT ( 'NONE',  ( -336.3521761649654422, -154.8494888031386836, 50.05135858667791382 ) ) ;
#35285=CARTESIAN_POINT ( 'NONE',  ( -336.3521761649654422, -123.5000000000000284, 0.000000000000000000 ) ) ;
#35287=CARTESIAN_POINT ( 'NONE',  ( -336.3521761649654422, -123.5000000000000284, 0.000000000000000000 ) ) ;
#35288=VERTEX_POINT ( 'NONE', #41505 ) ;
#35290=FACE_OUTER_BOUND ( 'NONE', #39725, .T. ) ;
#35301=LINE ( 'NONE', #4034, #33353 ) ;
#35302=ORIENTED_EDGE ( 'NONE', *, *, #15654, .F. ) ;
#35307=DIRECTION ( 'NONE',  ( 0.000000000000000000, -0.3546048870425331789, 0.9350162426854158326 ) ) ;
#35318=EDGE_CURVE ( 'NONE', #15872, #22804, #14196, .T. ) ;
#35319=AXIS2_PLACEMENT_3D ( 'NONE', #36003, #23899, #16035 ) ;
#35326=PLANE ( 'NONE',  #4752 ) ;
#35327=PLANE ( 'NONE',  #11948 ) ;
#35328=CARTESIAN_POINT ( 'NONE',  ( -330.4913330509368166, -175.5095439275173419, 27.86139516340933042 ) ) ;
#35329=ORIENTED_EDGE ( 'NONE', *, *, #33062, .T. ) ;
#35332=CARTESIAN_POINT ( 'NONE',  ( -330.4913330509368166, -171.7720157143599238, 33.92731199008539278 ) ) ;
#35335=CARTESIAN_POINT ( 'NONE',  ( -330.4913330509368166, -123.5000000000000284, 0.000000000000000000 ) ) ;
#35337=EDGE_CURVE ( 'NONE', #32161, #49023, #50261, .T. ) ;
#35338=DIRECTION ( 'NONE',  ( 0.000000000000000000, -0.9927088740980527515, 0.1205366802553337890 ) ) ;
#35345=EDGE_LOOP ( 'NONE', ( #46075, #49002, #49669, #20869 ) ) ;
#35346=DIRECTION ( 'NONE',  ( 0.000000000000000000, 0.9709418174260553425, 0.2393156642875449158 ) ) ;
#35347=DIRECTION ( 'NONE',  ( 1.000000000000000000, 0.000000000000000000, -0.000000000000000000 ) ) ;
#35349=AXIS2_PLACEMENT_3D ( 'NONE', #12779, #4923, #8842 ) ;
#35350=ORIENTED_EDGE ( 'NONE', *, *, #39691, .F. ) ;
#35351=CARTESIAN_POINT ( 'NONE',  ( -339.1964088526558498, -178.8432607619606358, 20.45418021416736565 ) ) ;
#35352=AXIS2_PLACEMENT_3D ( 'NONE', #2199, #14297, #42134 ) ;
#35354=ORIENTED_EDGE ( 'NONE', *, *, #31996, .F. ) ;
#35362=VECTOR ( 'NONE', #9443, 1000.000000000000114 ) ;
#35366=LINE ( 'NONE', #7528, #37760 ) ;
#35368=DIRECTION ( 'NONE',  ( 0.000000000000000000, 0.4647231720437695057, 0.8854560256532093554 ) ) ;
#35370=CARTESIAN_POINT ( 'NONE',  ( -330.4913330509368166, -123.0000000000002700, -59.00000000000002132 ) ) ;
#35375=ORIENTED_EDGE ( 'NONE', *, *, #18496, .T. ) ;
#35376=DIRECTION ( 'NONE',  ( -0.000000000000000000, 0.9709418174260553425, 0.2393156642875449158 ) ) ;
#35379=DIRECTION ( 'NONE',  ( 0.000000000000000000, -0.9709418174260544543, -0.2393156642875482465 ) ) ;
#35386=AXIS2_PLACEMENT_3D ( 'NONE', #26686, #18540, #49835 ) ;
#35388=AXIS2_PLACEMENT_3D ( 'NONE', #47901, #7692, #23216 ) ;
#35389=ORIENTED_EDGE ( 'NONE', *, *, #20563, .T. ) ;
#35392=EDGE_CURVE ( 'NONE', #4433, #10455, #9993, .T. ) ;
#35398=ORIENTED_EDGE ( 'NONE', *, *, #18619, .F. ) ;
#35404=ORIENTED_EDGE ( 'NONE', *, *, #10035, .F. ) ;
#35407=DIRECTION ( 'NONE',  ( 0.000000000000000000, 0.9927088740980534176, -0.1205366802553268502 ) ) ;
#35408=CARTESIAN_POINT ( 'NONE',  ( -336.3521761649654422, -182.3871109312487420, -4.498567634386014369 ) ) ;
#35410=CARTESIAN_POINT ( 'NONE',  ( -332.3517673607765914, -65.58448481710581746, 11.56382487286456140 ) ) ;
#35411=EDGE_CURVE ( 'NONE', #6696, #44669, #8309, .T. ) ;
#35416=EDGE_LOOP ( 'NONE', ( #36046, #31416, #41904, #51527 ) ) ;
#35420=AXIS2_PLACEMENT_3D ( 'NONE', #42534, #6555, #22581 ) ;
#35423=DIRECTION ( 'NONE',  ( -1.000000000000000000, 0.000000000000000000, 0.000000000000000000 ) ) ;
#35432=CARTESIAN_POINT ( 'NONE',  ( -332.3517673607765914, -159.1821513111375452, -47.06073758877369073 ) ) ;
#35433=SURFACE_STYLE_USAGE ( .BOTH. , #19411 ) ;
#35438=EDGE_LOOP ( 'NONE', ( #34240, #31377, #42062, #31585 ) ) ;
#35445=DIRECTION ( 'NONE',  ( -0.000000000000000000, 0.000000000000000000, -1.000000000000000000 ) ) ;
#35447=CARTESIAN_POINT ( 'NONE',  ( -305.0000000000000568, -153.6873197461136442, -51.85292399224849191 ) ) ;
#35455=VERTEX_POINT ( 'NONE', #39110 ) ;
#35465=CARTESIAN_POINT ( 'NONE',  ( -336.3521761649654422, -180.3949349376675855, 15.70448169564087770 ) ) ;
#35466=ORIENTED_EDGE ( 'NONE', *, *, #50823, .F. ) ;
#35467=ORIENTED_EDGE ( 'NONE', *, *, #48807, .T. ) ;
#35476=ORIENTED_EDGE ( 'NONE', *, *, #31346, .F. ) ;
#35477=ADVANCED_FACE ( 'NONE', ( #23365 ), #35960, .F. ) ;
#35492=CARTESIAN_POINT ( 'NONE',  ( -339.1964088526558498, -182.5000000000000568, 0.5000000000000457412 ) ) ;
#35494=LINE ( 'NONE', #47089, #34200 ) ;
#35495=EDGE_LOOP ( 'NONE', ( #21119, #17745 ) ) ;
#35502=CARTESIAN_POINT ( 'NONE',  ( -330.4913330509368166, -108.8949048983204904, 57.16590939599316812 ) ) ;
#35506=AXIS2_PLACEMENT_3D ( 'NONE', #1021, #32822, #13115 ) ;
#35518=PLANE ( 'NONE',  #35712 ) ;
#35520=FACE_OUTER_BOUND ( 'NONE', #38766, .T. ) ;
#35521=ORIENTED_EDGE ( 'NONE', *, *, #39344, .T. ) ;
#35522=DIRECTION ( 'NONE',  ( 0.000000000000000000, -0.9709418174260502354, 0.2393156642875652051 ) ) ;
#35524=VECTOR ( 'NONE', #1861, 1000.000000000000000 ) ;
#35535=VERTEX_POINT ( 'NONE', #11517 ) ;
#35537=ADVANCED_FACE ( 'NONE', ( #11771 ), #31757, .F. ) ;
#35538=CARTESIAN_POINT ( 'NONE',  ( -339.1964088526558498, -109.8658467157464571, 57.40522506028071348 ) ) ;
#35541=DIRECTION ( 'NONE',  ( 1.000000000000000000, -0.000000000000000000, 0.000000000000000000 ) ) ;
#35543=CIRCLE ( 'NONE', #1113, 60.00000000000000000 ) ;
#35548=DIRECTION ( 'NONE',  ( 0.000000000000000000, -0.9709418174260535661, -0.2393156642875516327 ) ) ;
#35550=EDGE_CURVE ( 'NONE', #36303, #29857, #51479, .T. ) ;
#35561=CARTESIAN_POINT ( 'NONE',  ( -336.3521761649654422, -180.3949349376675855, 15.70448169564087770 ) ) ;
#35564=VERTEX_POINT ( 'NONE', #4168 ) ;
#35569=VECTOR ( 'NONE', #29585, 1000.000000000000000 ) ;
#35571=EDGE_LOOP ( 'NONE', ( #17954, #29286, #32845, #45733 ) ) ;
#35576=CARTESIAN_POINT ( 'NONE',  ( -330.4913330509368166, -95.63860483659122735, -52.00954392751761191 ) ) ;
#35578=CARTESIAN_POINT ( 'NONE',  ( -332.3517673607765914, -105.0395444947681369, -56.09938080879045685 ) ) ;
#35580=CARTESIAN_POINT ( 'NONE',  ( -336.3521761649654422, -154.8494888031386836, 50.05135858667791382 ) ) ;
#35583=ORIENTED_EDGE ( 'NONE', *, *, #22659, .T. ) ;
#35584=DIRECTION ( 'NONE',  ( 0.000000000000000000, 0.000000000000000000, 1.000000000000000000 ) ) ;
#35588=CARTESIAN_POINT ( 'NONE',  ( -330.4913330509368166, -178.8432607619609200, -20.45418021416661247 ) ) ;
#35592=LINE ( 'NONE', #28233, #13561 ) ;
#35596=FACE_OUTER_BOUND ( 'NONE', #49574, .T. ) ;
#35601=EDGE_CURVE ( 'NONE', #50590, #8376, #17291, .T. ) ;
#35605=FACE_OUTER_BOUND ( 'NONE', #8403, .T. ) ;
#35609=FACE_OUTER_BOUND ( 'NONE', #9550, .T. ) ;
#35611=CARTESIAN_POINT ( 'NONE',  ( -336.3521761649654422, -81.08339623743702873, -41.09453333279329712 ) ) ;
#35617=EDGE_CURVE ( 'NONE', #49368, #25876, #17038, .T. ) ;
#35618=PLANE ( 'NONE',  #17694 ) ;
#35621=ORIENTED_EDGE ( 'NONE', *, *, #16377, .F. ) ;
#35624=ORIENTED_EDGE ( 'NONE', *, *, #4843, .T. ) ;
#35628=PLANE ( 'NONE',  #19270 ) ;
#35630=DIRECTION ( 'NONE',  ( -0.000000000000000000, 0.4647231720437664526, -0.8854560256532110207 ) ) ;
#35636=ORIENTED_EDGE ( 'NONE', *, *, #41082, .T. ) ;
#35643=AXIS2_PLACEMENT_3D ( 'NONE', #28081, #43611, #39396 ) ;
#35650=ADVANCED_FACE ( 'NONE', ( #10690 ), #9654, .F. ) ;
#35653=PLANE ( 'NONE',  #407 ) ;
#35661=AXIS2_PLACEMENT_3D ( 'NONE', #11136, #7206, #51883 ) ;
#35662=CARTESIAN_POINT ( 'NONE',  ( -339.1964088526558498, -176.8578783931341150, -27.43969411971490047 ) ) ;
#35664=DIRECTION ( 'NONE',  ( -0.000000000000000000, 0.000000000000000000, -1.000000000000000000 ) ) ;
#35668=EDGE_CURVE ( 'NONE', #24027, #20203, #42481, .T. ) ;
#35669=ORIENTED_EDGE ( 'NONE', *, *, #16274, .T. ) ;
#35670=EDGE_CURVE ( 'NONE', #16559, #8474, #18058, .T. ) ;
#35673=LINE ( 'NONE', #30694, #4978 ) ;
#35674=AXIS2_PLACEMENT_3D ( 'NONE', #47889, #19496, #20021 ) ;
#35679=AXIS2_PLACEMENT_3D ( 'NONE', #31726, #23832, #8067 ) ;
#35682=AXIS2_PLACEMENT_3D ( 'NONE', #15724, #3880, #7812 ) ;
#35693=VECTOR ( 'NONE', #1770, 1000.000000000000000 ) ;
#35694=DIRECTION ( 'NONE',  ( -0.000000000000000000, 0.5680647467311656929, 0.8229838658936495799 ) ) ;
#35695=DIRECTION ( 'NONE',  ( -0.000000000000000000, 0.1205366802553199113, -0.9927088740980544168 ) ) ;
#35699=ORIENTED_EDGE ( 'NONE', *, *, #28544, .F. ) ;
#35700=LINE ( 'NONE', #30719, #49148 ) ;
#35704=LINE ( 'NONE', #3390, #33470 ) ;
#35707=DIRECTION ( 'NONE',  ( 1.000000000000000000, 0.000000000000000000, 0.000000000000000000 ) ) ;
#35708=ORIENTED_EDGE ( 'NONE', *, *, #25963, .F. ) ;
#35712=AXIS2_PLACEMENT_3D ( 'NONE', #11862, #44460, #28149 ) ;
#35715=DIRECTION ( 'NONE',  ( 0.000000000000000000, 0.1205366802553164696, -0.9927088740980548609 ) ) ;
#35717=CIRCLE ( 'NONE', #4666, 60.00000000000000000 ) ;
#35719=VECTOR ( 'NONE', #45765, 1000.000000000000114 ) ;
#35724=LINE ( 'NONE', #18931, #32133 ) ;
#35728=VECTOR ( 'NONE', #11607, 1000.000000000000000 ) ;
#35729=VECTOR ( 'NONE', #14692, 1000.000000000000000 ) ;
#35733=ADVANCED_FACE ( 'NONE', ( #13859 ), #25938, .T. ) ;
#35739=CARTESIAN_POINT ( 'NONE',  ( -305.0000000000000568, -97.07224986041923387, -53.86626052140510978 ) ) ;
#35745=ORIENTED_EDGE ( 'NONE', *, *, #24571, .T. ) ;
#35747=EDGE_LOOP ( 'NONE', ( #17037, #3285, #37994, #25231 ) ) ;
#35757=ORIENTED_EDGE ( 'NONE', *, *, #41383, .F. ) ;
#35760=CARTESIAN_POINT ( 'NONE',  ( -305.0000000000000568, -123.5000000000000284, -60.00000000000000000 ) ) ;
#35761=AXIS2_PLACEMENT_3D ( 'NONE', #9748, #41273, #22088 ) ;
#35763=LINE ( 'NONE', #12091, #23897 ) ;
#35764=VERTEX_POINT ( 'NONE', #14375 ) ;
#35766=VECTOR ( 'NONE', #7000, 1000.000000000000114 ) ;
#35767=CARTESIAN_POINT ( 'NONE',  ( -305.0000000000000568, -179.7763290203206452, 20.80804632820241551 ) ) ;
#35770=EDGE_LOOP ( 'NONE', ( #5009, #6868, #8197, #5891 ) ) ;
#35774=( LENGTH_UNIT ( ) NAMED_UNIT ( * ) SI_UNIT ( .MILLI., .METRE. ) );
#35775=ORIENTED_EDGE ( 'NONE', *, *, #4476, .F. ) ;
#35779=EDGE_CURVE ( 'NONE', #19701, #32359, #18575, .T. ) ;
#35782=DIRECTION ( 'NONE',  ( 0.000000000000000000, 0.9350162426854194964, 0.3546048870425235200 ) ) ;
#35784=ORIENTED_EDGE ( 'NONE', *, *, #33600, .T. ) ;
#35785=DIRECTION ( 'NONE',  ( 1.000000000000000000, -0.000000000000000000, 0.000000000000000000 ) ) ;
#35786=ORIENTED_EDGE ( 'NONE', *, *, #15389, .F. ) ;
#35788=AXIS2_PLACEMENT_3D ( 'NONE', #46106, #25334, #41350 ) ;
#35795=EDGE_CURVE ( 'NONE', #40543, #39339, #14206, .T. ) ;
#35796=EDGE_CURVE ( 'NONE', #26067, #43448, #2297, .T. ) ;
#35797=CARTESIAN_POINT ( 'NONE',  ( -339.1964088526558498, -64.99044476834248485, -7.608018572113150135 ) ) ;
#35800=AXIS2_PLACEMENT_3D ( 'NONE', #20058, #51121, #19537 ) ;
#35802=CARTESIAN_POINT ( 'NONE',  ( -330.4913330509368166, -79.66942718702493664, 39.49849221029193558 ) ) ;
#35804=ORIENTED_EDGE ( 'NONE', *, *, #39774, .T. ) ;
#35806=VECTOR ( 'NONE', #48874, 1000.000000000000000 ) ;
#35808=EDGE_LOOP ( 'NONE', ( #31412, #6694, #16195, #1152 ) ) ;
#35811=VECTOR ( 'NONE', #344, 1000.000000000000000 ) ;
#35813=VERTEX_POINT ( 'NONE', #27743 ) ;
#35814=ORIENTED_EDGE ( 'NONE', *, *, #30449, .F. ) ;
#35816=EDGE_CURVE ( 'NONE', #34017, #18494, #42217, .T. ) ;
#35817=LINE ( 'NONE', #44952, #49369 ) ;
#35818=CARTESIAN_POINT ( 'NONE',  ( -336.3521761649654422, -69.26746417191145611, -23.38292116578723068 ) ) ;
#35822=ORIENTED_EDGE ( 'NONE', *, *, #50823, .T. ) ;
#35823=ORIENTED_EDGE ( 'NONE', *, *, #49465, .F. ) ;
#35828=VECTOR ( 'NONE', #9255, 1000.000000000000000 ) ;
#35831=EDGE_LOOP ( 'NONE', ( #51901, #7577, #39442, #21671 ) ) ;
#35837=EDGE_LOOP ( 'NONE', ( #50574, #34781, #19409, #38674 ) ) ;
#35840=CARTESIAN_POINT ( 'NONE',  ( -336.3521761649654422, -126.1322888500942270, -59.00000000000001421 ) ) ;
#35845=VECTOR ( 'NONE', #3707, 1000.000000000000114 ) ;
#35848=ADVANCED_FACE ( 'NONE', ( #31173 ), #35628, .T. ) ;
#35853=VECTOR ( 'NONE', #29698, 1000.000000000000000 ) ;
#35858=ORIENTED_EDGE ( 'NONE', *, *, #9901, .F. ) ;
#35859=CARTESIAN_POINT ( 'NONE',  ( -330.4913330509368166, -123.5000000000000284, 0.000000000000000000 ) ) ;
#35867=ORIENTED_EDGE ( 'NONE', *, *, #37150, .F. ) ;
#35870=AXIS2_PLACEMENT_3D ( 'NONE', #31247, #47300, #50990 ) ;
#35872=DIRECTION ( 'NONE',  ( -0.000000000000000000, -0.3546048870425267951, 0.9350162426854181641 ) ) ;
#35874=VERTEX_POINT ( 'NONE', #27490 ) ;
#35878=DIRECTION ( 'NONE',  ( -0.000000000000000000, -0.8229838658936596829, -0.5680647467311510379 ) ) ;
#35881=ORIENTED_EDGE ( 'NONE', *, *, #38701, .F. ) ;
#35882=CARTESIAN_POINT ( 'NONE',  ( 0.000000000000000000, -180.7855672281370119, 14.11962419296635396 ) ) ;
#35883=VECTOR ( 'NONE', #43901, 1000.000000000000000 ) ;
#35888=AXIS2_PLACEMENT_3D ( 'NONE', #37725, #25626, #50339 ) ;
#35889=VECTOR ( 'NONE', #43609, 1000.000000000000000 ) ;
#35893=ORIENTED_EDGE ( 'NONE', *, *, #25013, .T. ) ;
#35894=ORIENTED_EDGE ( 'NONE', *, *, #8774, .T. ) ;
#35895=VECTOR ( 'NONE', #4749, 1000.000000000000114 ) ;
#35898=CARTESIAN_POINT ( 'NONE',  ( -305.0000000000000568, -89.82879061784676367, -49.66134974749672182 ) ) ;
#35899=CARTESIAN_POINT ( 'NONE',  ( -332.3517673607765914, -169.4076645216271402, -37.15394033962039089 ) ) ;
#35900=DIRECTION ( 'NONE',  ( -1.000000000000000000, -0.000000000000000000, -0.000000000000000000 ) ) ;
#35904=ORIENTED_EDGE ( 'NONE', *, *, #10225, .F. ) ;
#35906=EDGE_LOOP ( 'NONE', ( #29737, #11364, #47150, #9753 ) ) ;
#35915=EDGE_CURVE ( 'NONE', #8372, #34970, #16765, .T. ) ;
#35919=CARTESIAN_POINT ( 'NONE',  ( -180.0000000000000568, -123.5000000000000284, -15.24495751795539000 ) ) ;
#35925=DIRECTION ( 'NONE',  ( 1.000000000000000000, -1.050884489711542826E-17, 8.654812430365590163E-17 ) ) ;
#35926=CARTESIAN_POINT ( 'NONE',  ( -336.3521761649654422, -65.24746378767824240, -9.724760635741734660 ) ) ;
#35927=CARTESIAN_POINT ( 'NONE',  ( -332.3517673607765914, -67.75522407825191351, 19.39547174791671935 ) ) ;
#35928=CARTESIAN_POINT ( 'NONE',  ( -339.1964088526558498, -68.51134412508183402, -21.38919645685240312 ) ) ;
#35933=EDGE_CURVE ( 'NONE', #12706, #46515, #33945, .T. ) ;
#35937=EDGE_CURVE ( 'NONE', #28874, #3974, #24327, .T. ) ;
#35945=EDGE_CURVE ( 'NONE', #27120, #32525, #32472, .T. ) ;
#35947=LINE ( 'NONE', #8350, #20073 ) ;
#35949=CIRCLE ( 'NONE', #42663, 60.00000000000000000 ) ;
#35955=VERTEX_POINT ( 'NONE', #40865 ) ;
#35958=VECTOR ( 'NONE', #37763, 1000.000000000000000 ) ;
#35960=PLANE ( 'NONE',  #39354 ) ;
#35967=CARTESIAN_POINT ( 'NONE',  ( -305.0000000000000568, -162.9117225908391333, -45.24064679492040852 ) ) ;
#35968=ORIENTED_EDGE ( 'NONE', *, *, #9969, .T. ) ;
#35975=ADVANCED_FACE ( 'NONE', ( #36403 ), #10054, .F. ) ;
#35980=ORIENTED_EDGE ( 'NONE', *, *, #34025, .T. ) ;
#35981=EDGE_CURVE ( 'NONE', #33577, #40405, #41131, .T. ) ;
#35985=LINE ( 'NONE', #35447, #48910 ) ;
#35986=VECTOR ( 'NONE', #48476, 1000.000000000000114 ) ;
#35990=PLANE ( 'NONE',  #26545 ) ;
#35994=ORIENTED_EDGE ( 'NONE', *, *, #36263, .F. ) ;
#36003=CARTESIAN_POINT ( 'NONE',  ( -305.0000000000000568, -123.5000000000000284, 0.000000000000000000 ) ) ;
#36009=VECTOR ( 'NONE', #44836, 1000.000000000000000 ) ;
#36011=PLANE ( 'NONE',  #17807 ) ;
#36014=ORIENTED_EDGE ( 'NONE', *, *, #22486, .F. ) ;
#36015=DIRECTION ( 'NONE',  ( 1.000000000000000000, 0.000000000000000000, -0.000000000000000000 ) ) ;
#36021=DIRECTION ( 'NONE',  ( 0.000000000000000000, 0.000000000000000000, -1.000000000000000000 ) ) ;
#36024=FACE_OUTER_BOUND ( 'NONE', #20399, .T. ) ;
#36026=LINE ( 'NONE', #40216, #51847 ) ;
#36027=ORIENTED_EDGE ( 'NONE', *, *, #20670, .F. ) ;
#36030=CARTESIAN_POINT ( 'NONE',  ( -336.3521761649654422, -69.26746417191145611, -23.38292116578723068 ) ) ;
#36033=CARTESIAN_POINT ( 'NONE',  ( -336.3521761649654422, -165.9166037625627439, 41.09453333279358134 ) ) ;
#36042=VERTEX_POINT ( 'NONE', #44559 ) ;
#36046=ORIENTED_EDGE ( 'NONE', *, *, #7472, .T. ) ;
#36048=LINE ( 'NONE', #48406, #39044 ) ;
#36052=AXIS2_PLACEMENT_3D ( 'NONE', #2779, #34571, #10930 ) ;
#36053=CARTESIAN_POINT ( 'NONE',  ( -332.3517673607765914, -171.1288023355047585, 34.85916744524404720 ) ) ;
#36054=DIRECTION ( 'NONE',  ( 0.000000000000000000, -1.137978600240785454E-13, -1.000000000000000000 ) ) ;
#36058=CARTESIAN_POINT ( 'NONE',  ( -330.4913330509368166, -171.7720157143604069, -33.92731199008473197 ) ) ;
#36059=ADVANCED_FACE ( 'NONE', ( #32977, #4613 ), #2150, .T. ) ;
#36071=VERTEX_POINT ( 'NONE', #30790 ) ;
#36081=ADVANCED_FACE ( 'NONE', ( #50516 ), #51046, .F. ) ;
#36086=CARTESIAN_POINT ( 'NONE',  ( -330.4913330509368166, -79.00630452878421295, 38.74998146212088557 ) ) ;
#36089=CARTESIAN_POINT ( 'NONE',  ( -339.1964088526558498, -116.8846903019852164, -58.63009191191289915 ) ) ;
#36093=DIRECTION ( 'NONE',  ( 1.000000000000000000, 0.000000000000000000, 0.000000000000000000 ) ) ;
#36095=ORIENTED_EDGE ( 'NONE', *, *, #2799, .F. ) ;
#36096=EDGE_CURVE ( 'NONE', #22268, #11734, #34722, .T. ) ;
#36099=DIRECTION ( 'NONE',  ( -0.000000000000000000, 0.9927088740980538617, -0.1205366802553232974 ) ) ;
#36103=EDGE_CURVE ( 'NONE', #26805, #28748, #14515, .T. ) ;
#36105=ORIENTED_EDGE ( 'NONE', *, *, #916, .F. ) ;
#36108=VECTOR ( 'NONE', #42845, 999.9999999999998863 ) ;
#36111=ORIENTED_EDGE ( 'NONE', *, *, #39812, .T. ) ;
#36117=DIRECTION ( 'NONE',  ( 1.000000000000000000, -0.000000000000000000, 0.000000000000000000 ) ) ;
#36118=CARTESIAN_POINT ( 'NONE',  ( -336.3521761649654422, -70.49953203435293858, 25.97334715265942151 ) ) ;
#36125=DIRECTION ( 'NONE',  ( 0.000000000000000000, 0.9927088740980556381, 0.1205366802553095168 ) ) ;
#36127=ORIENTED_EDGE ( 'NONE', *, *, #48297, .F. ) ;
#36128=VERTEX_POINT ( 'NONE', #31039 ) ;
#36132=DIRECTION ( 'NONE',  ( 0.000000000000000000, -0.8229838658936536877, 0.5680647467311596976 ) ) ;
#36134=ORIENTED_EDGE ( 'NONE', *, *, #2143, .T. ) ;
#36135=CARTESIAN_POINT ( 'NONE',  ( -330.4913330509368166, -175.5095439275177398, -27.86139516340860212 ) ) ;
#36136=CARTESIAN_POINT ( 'NONE',  ( -336.3521761649654422, -123.5000000000000284, 0.000000000000000000 ) ) ;
#36137=VECTOR ( 'NONE', #29521, 999.9999999999998863 ) ;
#36140=CARTESIAN_POINT ( 'NONE',  ( -330.4913330509368166, -84.08827740916123616, -45.24064679492067853 ) ) ;
#36148=LINE ( 'NONE', #16451, #5034 ) ;
#36150=FACE_BOUND ( 'NONE', #2469, .T. ) ;
#36160=EDGE_CURVE ( 'NONE', #41614, #35813, #34377, .T. ) ;
#36163=CARTESIAN_POINT ( 'NONE',  ( 0.000000000000000000, -144.4216883355098844, -55.16595831843940090 ) ) ;
#36168=ORIENTED_EDGE ( 'NONE', *, *, #35411, .F. ) ;
#36169=ORIENTED_EDGE ( 'NONE', *, *, #22462, .F. ) ;
#36176=ORIENTED_EDGE ( 'NONE', *, *, #1927, .T. ) ;
#36189=LINE ( 'NONE', #24626, #48926 ) ;
#36191=ADVANCED_FACE ( 'NONE', ( #50771 ), #31296, .F. ) ;
#36193=ADVANCED_FACE ( 'NONE', ( #46833 ), #10820, .F. ) ;
#36194=DIRECTION ( 'NONE',  ( 0.000000000000000000, 0.5680647467311596976, 0.8229838658936536877 ) ) ;
#36203=DIRECTION ( 'NONE',  ( -1.000000000000000000, 0.000000000000000000, 0.000000000000000000 ) ) ;
#36208=VECTOR ( 'NONE', #1359, 1000.000000000000000 ) ;
#36210=LINE ( 'NONE', #206, #11348 ) ;
#36217=LINE ( 'NONE', #25187, #8059 ) ;
#36218=ORIENTED_EDGE ( 'NONE', *, *, #21985, .F. ) ;
#36221=ADVANCED_FACE ( 'NONE', ( #16588 ), #36271, .F. ) ;
#36226=ORIENTED_EDGE ( 'NONE', *, *, #29400, .F. ) ;
#36227=AXIS2_PLACEMENT_3D ( 'NONE', #4019, #37097, #39990 ) ;
#36229=DIRECTION ( 'NONE',  ( -0.000000000000000000, -0.9927088740980530845, 0.1205366802553303057 ) ) ;
#36231=VECTOR ( 'NONE', #23428, 1000.000000000000000 ) ;
#36233=CARTESIAN_POINT ( 'NONE',  ( -336.3521761649654422, -120.8677111499054320, 59.00000000000000000 ) ) ;
#36236=ORIENTED_EDGE ( 'NONE', *, *, #11875, .T. ) ;
#36241=PLANE ( 'NONE',  #40524 ) ;
#36242=ORIENTED_EDGE ( 'NONE', *, *, #22462, .T. ) ;
#36246=DIRECTION ( 'NONE',  ( 0.000000000000000000, -0.8854560256532044704, 0.4647231720437789981 ) ) ;
#36252=EDGE_CURVE ( 'NONE', #26962, #20303, #48114, .T. ) ;
#36256=ORIENTED_EDGE ( 'NONE', *, *, #34076, .T. ) ;
#36259=EDGE_CURVE ( 'NONE', #51089, #46182, #4227, .T. ) ;
#36260=FACE_OUTER_BOUND ( 'NONE', #1165, .T. ) ;
#36263=EDGE_CURVE ( 'NONE', #8885, #50347, #4488, .T. ) ;
#36264=ORIENTED_EDGE ( 'NONE', *, *, #19516, .F. ) ;
#36267=ORIENTED_EDGE ( 'NONE', *, *, #19334, .T. ) ;
#36270=EDGE_LOOP ( 'NONE', ( #45682, #21736, #26496, #42392 ) ) ;
#36271=PLANE ( 'NONE',  #40140 ) ;
#36272=PLANE ( 'NONE',  #18522 ) ;
#36273=DIRECTION ( 'NONE',  ( -0.000000000000000000, 0.2393156642875547968, -0.9709418174260527890 ) ) ;
#36278=EDGE_LOOP ( 'NONE', ( #8320, #15862 ) ) ;
#36280=VECTOR ( 'NONE', #43352, 1000.000000000000000 ) ;
#36283=CARTESIAN_POINT ( 'NONE',  ( -336.3521761649654422, -67.75522407825191351, 19.39547174791671935 ) ) ;
#36295=FACE_OUTER_BOUND ( 'NONE', #10675, .T. ) ;
#36298=CARTESIAN_POINT ( 'NONE',  ( -336.3521761649654422, -181.0704707379907745, 16.90091414705587525 ) ) ;
#36300=FACE_OUTER_BOUND ( 'NONE', #42999, .T. ) ;
#36303=VERTEX_POINT ( 'NONE', #3436 ) ;
#36308=CARTESIAN_POINT ( 'NONE',  ( -330.4913330509368166, -182.1300919119129560, -6.615309698014691264 ) ) ;
#36309=CARTESIAN_POINT ( 'NONE',  ( -336.3521761649654422, -65.92952926200918284, -16.90091414705545247 ) ) ;
#36311=DIRECTION ( 'NONE',  ( 0.000000000000000000, 0.8229838658936536877, -0.5680647467311596976 ) ) ;
#36313=VECTOR ( 'NONE', #13124, 1000.000000000000000 ) ;
#36316=CARTESIAN_POINT ( 'NONE',  ( -305.0000000000000568, -118.8878589706978914, -59.82247199109903590 ) ) ;
#36317=DIRECTION ( 'NONE',  ( -1.000000000000000000, -0.000000000000000000, 0.000000000000000000 ) ) ;
#36323=ADVANCED_FACE ( 'NONE', ( #45476 ), #36805, .F. ) ;
#36324=CARTESIAN_POINT ( 'NONE',  ( -330.0000000000000568, -123.5000000000000284, -31.65769145387501027 ) ) ;
#36331=DIRECTION ( 'NONE',  ( 0.000000000000000000, 0.2393156642875685636, 0.9709418174260492362 ) ) ;
#36333=VECTOR ( 'NONE', #50742, 1000.000000000000000 ) ;
#36337=ORIENTED_EDGE ( 'NONE', *, *, #49078, .T. ) ;
#36339=LINE ( 'NONE', #333, #42824 ) ;
#36346=ORIENTED_EDGE ( 'NONE', *, *, #41565, .F. ) ;
#36348=VECTOR ( 'NONE', #22513, 1000.000000000000000 ) ;
#36352=EDGE_CURVE ( 'NONE', #37026, #31066, #1313, .T. ) ;
#36354=VERTEX_POINT ( 'NONE', #21820 ) ;
#36357=CARTESIAN_POINT ( 'NONE',  ( -305.0000000000000568, -108.6560878169898956, 58.13482838284708976 ) ) ;
#36360=VECTOR ( 'NONE', #18422, 1000.000000000000000 ) ;
#36362=ORIENTED_EDGE ( 'NONE', *, *, #29996, .T. ) ;
#36369=FACE_OUTER_BOUND ( 'NONE', #36429, .T. ) ;
#36370=ORIENTED_EDGE ( 'NONE', *, *, #852, .T. ) ;
#36375=CARTESIAN_POINT ( 'NONE',  ( -332.3517673607765914, -65.24746378767824240, -9.724760635741734660 ) ) ;
#36376=ORIENTED_EDGE ( 'NONE', *, *, #41980, .T. ) ;
#36377=CARTESIAN_POINT ( 'NONE',  ( -339.1964088526558498, -130.1153096980144426, 58.63009191191295599 ) ) ;
#36387=DIRECTION ( 'NONE',  ( -1.000000000000000000, -0.000000000000000000, 0.000000000000000000 ) ) ;
#36388=ORIENTED_EDGE ( 'NONE', *, *, #14346, .T. ) ;
#36389=LINE ( 'NONE', #40319, #7967 ) ;
#36391=LINE ( 'NONE', #43517, #26659 ) ;
#36393=AXIS2_PLACEMENT_3D ( 'NONE', #5506, #9185, #17076 ) ;
#36394=CARTESIAN_POINT ( 'NONE',  ( -339.1964088526558498, -156.6043281241909426, 48.84008046109164525 ) ) ;
#36395=CARTESIAN_POINT ( 'NONE',  ( -339.1964088526558498, -151.3613951634084742, 52.00954392751779665 ) ) ;
#36403=FACE_OUTER_BOUND ( 'NONE', #33973, .T. ) ;
#36404=FACE_BOUND ( 'NONE', #24962, .T. ) ;
#36405=CARTESIAN_POINT ( 'NONE',  ( -336.3521761649654422, -98.41210887299327226, -53.46519113769058151 ) ) ;
#36406=ORIENTED_EDGE ( 'NONE', *, *, #25497, .T. ) ;
#36407=VECTOR ( 'NONE', #49866, 1000.000000000000000 ) ;
#36415=CARTESIAN_POINT ( 'NONE',  ( -305.0000000000000568, -84.08827740916102300, -45.24064679492050089 ) ) ;
#36418=VERTEX_POINT ( 'NONE', #46007 ) ;
#36419=ORIENTED_EDGE ( 'NONE', *, *, #18012, .T. ) ;
#36429=EDGE_LOOP ( 'NONE', ( #26971, #31690, #33609, #30330 ) ) ;
#36430=DIRECTION ( 'NONE',  ( -1.000000000000000000, 0.000000000000000000, 0.000000000000000000 ) ) ;
#36432=CIRCLE ( 'NONE', #7047, 60.00000000000000000 ) ;
#36441=EDGE_CURVE ( 'NONE', #32906, #32186, #9469, .T. ) ;
#36443=ORIENTED_EDGE ( 'NONE', *, *, #41068, .F. ) ;
#36444=ADVANCED_FACE ( 'NONE', ( #9994 ), #37054, .T. ) ;
#36445=DIRECTION ( 'NONE',  ( 0.000000000000000000, 0.8854560256532110207, 0.4647231720437664526 ) ) ;
#36446=EDGE_CURVE ( 'NONE', #37128, #10115, #35949, .T. ) ;
#36453=CARTESIAN_POINT ( 'NONE',  ( -336.3521761649654422, -104.7054247829104412, -56.98038208374145341 ) ) ;
#36456=CARTESIAN_POINT ( 'NONE',  ( -336.3521761649654422, -139.2044816956407089, -56.89493493766761389 ) ) ;
#36458=DIRECTION ( 'NONE',  ( 0.000000000000000000, 0.000000000000000000, -1.000000000000000000 ) ) ;
#36459=VECTOR ( 'NONE', #40683, 1000.000000000000114 ) ;
#36463=DIRECTION ( 'NONE',  ( 1.000000000000000000, 0.000000000000000000, 0.000000000000000000 ) ) ;
#36464=DIRECTION ( 'NONE',  ( 1.000000000000000000, 0.000000000000000000, 0.000000000000000000 ) ) ;
#36470=PLANE ( 'NONE',  #37371 ) ;
#36479=EDGE_LOOP ( 'NONE', ( #38176, #10846, #5516, #3106 ) ) ;
#36481=DIRECTION ( 'NONE',  ( -1.000000000000000000, 0.000000000000000000, 0.000000000000000000 ) ) ;
#36484=CARTESIAN_POINT ( 'NONE',  ( -305.0000000000000568, -123.5000000000000284, 20.00000000000000355 ) ) ;
#36489=PLANE ( 'NONE',  #41291 ) ;
#36490=LINE ( 'NONE', #45977, #9549 ) ;
#36497=EDGE_CURVE ( 'NONE', #7901, #18571, #14972, .T. ) ;
#36500=PLANE ( 'NONE',  #13499 ) ;
#36501=CARTESIAN_POINT ( 'NONE',  ( -336.3521761649654422, -164.5945333327934463, -42.41660376256285048 ) ) ;
#36505=ORIENTED_EDGE ( 'NONE', *, *, #18240, .T. ) ;
#36506=VECTOR ( 'NONE', #36311, 1000.000000000000114 ) ;
#36508=LINE ( 'NONE', #4730, #15072 ) ;
#36510=DIRECTION ( 'NONE',  ( 0.000000000000000000, -0.3546048870425426158, -0.9350162426854120579 ) ) ;
#36512=DIRECTION ( 'NONE',  ( 0.000000000000000000, -0.4647231720437664526, 0.8854560256532110207 ) ) ;
#36514=AXIS2_PLACEMENT_3D ( 'NONE', #42145, #6169, #1956 ) ;
#36520=VERTEX_POINT ( 'NONE', #38348 ) ;
#36522=VERTEX_POINT ( 'NONE', #2362 ) ;
#36525=DIRECTION ( 'NONE',  ( 0.000000000000000000, 0.000000000000000000, 1.000000000000000000 ) ) ;
#36526=CARTESIAN_POINT ( 'NONE',  ( -339.1964088526558498, -178.4886558749180949, 21.38919645685277970 ) ) ;
#36532=AXIS2_PLACEMENT_3D ( 'NONE', #11090, #42381, #50799 ) ;
#36536=CARTESIAN_POINT ( 'NONE',  ( -339.1964088526558498, -151.3613951634092700, -52.00954392751739164 ) ) ;
#36537=DIRECTION ( 'NONE',  ( 0.000000000000000000, 0.4647231720437789981, 0.8854560256532044704 ) ) ;
#36542=LINE ( 'NONE', #39959, #4808 ) ;
#36546=DIRECTION ( 'NONE',  ( 1.000000000000000000, -0.000000000000000000, 0.000000000000000000 ) ) ;
#36550=CIRCLE ( 'NONE', #28964, 60.00000000000000000 ) ;
#36552=CARTESIAN_POINT ( 'NONE',  ( -336.3521761649654422, -114.7679482383557144, 58.37307289257701370 ) ) ;
#36553=AXIS2_PLACEMENT_3D ( 'NONE', #42539, #26771, #34649 ) ;
#36555=ADVANCED_FACE ( 'NONE', ( #6817 ), #38859, .F. ) ;
#36557=EDGE_CURVE ( 'NONE', #31094, #23911, #34910, .T. ) ;
#36558=ORIENTED_EDGE ( 'NONE', *, *, #5807, .F. ) ;
#36564=EDGE_LOOP ( 'NONE', ( #49131, #9547, #32216, #25375 ) ) ;
#36566=EDGE_LOOP ( 'NONE', ( #49946, #31663, #34922, #13553 ) ) ;
#36567=LINE ( 'NONE', #569, #39050 ) ;
#36569=CARTESIAN_POINT ( 'NONE',  ( -339.1964088526558498, -150.9396941197155968, -53.35787839313373127 ) ) ;
#36572=CARTESIAN_POINT ( 'NONE',  ( -330.4913330509368166, -70.60684477890951882, 28.32515014536777542 ) ) ;
#36573=ADVANCED_FACE ( 'NONE', ( #39113 ), #43067, .F. ) ;
#36578=CARTESIAN_POINT ( 'NONE',  ( -330.4913330509368166, -144.8891964568525452, -54.98865587491815177 ) ) ;
#36579=LINE ( 'NONE', #11362, #1204 ) ;
#36585=EDGE_CURVE ( 'NONE', #46182, #8223, #39879, .T. ) ;
#36587=DIRECTION ( 'NONE',  ( 1.043714542225393539E-14, -0.8854560256532110207, -0.4647231720437664526 ) ) ;
#36591=VERTEX_POINT ( 'NONE', #27288 ) ;
#36593=ORIENTED_EDGE ( 'NONE', *, *, #1695, .F. ) ;
#36594=CARTESIAN_POINT ( 'NONE',  ( -332.3517673607765914, -175.3529239922484351, 30.18731974611377211 ) ) ;
#36595=VECTOR ( 'NONE', #51637, 1000.000000000000000 ) ;
#36598=LINE ( 'NONE', #32656, #36682 ) ;
#36599=ORIENTED_EDGE ( 'NONE', *, *, #17683, .F. ) ;
#36601=ADVANCED_FACE ( 'NONE', ( #7339 ), #8366, .T. ) ;
#36602=EDGE_CURVE ( 'NONE', #24982, #5217, #43328, .T. ) ;
#36604=DIRECTION ( 'NONE',  ( -0.000000000000000000, 0.3546048870425331789, -0.9350162426854158326 ) ) ;
#36606=DIRECTION ( 'NONE',  ( 0.000000000000000000, 0.000000000000000000, 1.000000000000000000 ) ) ;
#36608=CARTESIAN_POINT ( 'NONE',  ( -336.3521761649654422, -123.5000000000000284, 0.000000000000000000 ) ) ;
#36617=VECTOR ( 'NONE', #18547, 1000.000000000000000 ) ;
#36618=ORIENTED_EDGE ( 'NONE', *, *, #12192, .T. ) ;
#36619=CARTESIAN_POINT ( 'NONE',  ( -332.3517673607765914, -181.3443148879387081, 15.93848283698911317 ) ) ;
#36623=FACE_OUTER_BOUND ( 'NONE', #46419, .T. ) ;
#36625=CARTESIAN_POINT ( 'NONE',  ( -336.3521761649654422, -120.8677111499054178, 59.94223098458771659 ) ) ;
#36626=EDGE_CURVE ( 'NONE', #32221, #6345, #3907, .T. ) ;
#36627=EDGE_CURVE ( 'NONE', #46318, #43845, #8102, .T. ) ;
#36628=EDGE_LOOP ( 'NONE', ( #46000, #41195, #6653, #37114 ) ) ;
#36629=DIRECTION ( 'NONE',  ( 0.000000000000000000, -0.5680647467311485954, 0.8229838658936613482 ) ) ;
#36631=EDGE_CURVE ( 'NONE', #38201, #16449, #40157, .T. ) ;
#36632=ADVANCED_FACE ( 'NONE', ( #4420 ), #3634, .T. ) ;
#36643=DIRECTION ( 'NONE',  ( 1.000000000000000000, -0.000000000000000000, -0.000000000000000000 ) ) ;
#36644=VECTOR ( 'NONE', #33757, 999.9999999999998863 ) ;
#36645=DIRECTION ( 'NONE',  ( 0.000000000000000000, -1.047444401652940007E-14, -1.000000000000000000 ) ) ;
#36646=ORIENTED_EDGE ( 'NONE', *, *, #44570, .F. ) ;
#36647=DIRECTION ( 'NONE',  ( 0.000000000000000000, -0.4647231720437755564, -0.8854560256532062468 ) ) ;
#36652=DIRECTION ( 'NONE',  ( 0.000000000000000000, -0.8854560256532043594, 0.4647231720437789981 ) ) ;
#36654=ORIENTED_EDGE ( 'NONE', *, *, #51284, .T. ) ;
#36656=CARTESIAN_POINT ( 'NONE',  ( -332.3517673607765914, -77.59233547837267508, 37.15394033962009246 ) ) ;
#36659=AXIS2_PLACEMENT_3D ( 'NONE', #40834, #40306, #36645 ) ;
#36661=ORIENTED_EDGE ( 'NONE', *, *, #1208, .F. ) ;
#36663=VERTEX_POINT ( 'NONE', #20185 ) ;
#36664=PLANE ( 'NONE',  #18304 ) ;
#36666=VECTOR ( 'NONE', #12135, 1000.000000000000114 ) ;
#36669=VERTEX_POINT ( 'NONE', #16518 ) ;
#36675=CIRCLE ( 'NONE', #24898, 60.00000000000000000 ) ;
#36678=FACE_BOUND ( 'NONE', #38657, .T. ) ;
#36681=EDGE_LOOP ( 'NONE', ( #10730, #21877, #25489, #38393 ) ) ;
#36682=VECTOR ( 'NONE', #48700, 1000.000000000000000 ) ;
#36685=PLANE ( 'NONE',  #44093 ) ;
#36693=DIRECTION ( 'NONE',  ( -1.000000000000000000, 0.000000000000000000, 0.000000000000000000 ) ) ;
#36695=CARTESIAN_POINT ( 'NONE',  ( -339.1964088526558498, -102.1108035431470427, 54.98865587491797413 ) ) ;
#36696=EDGE_LOOP ( 'NONE', ( #32752, #41869, #37106, #33738 ) ) ;
#36700=VECTOR ( 'NONE', #8989, 1000.000000000000000 ) ;
#36704=VECTOR ( 'NONE', #49917, 1000.000000000000000 ) ;
#36708=ORIENTED_EDGE ( 'NONE', *, *, #3184, .F. ) ;
#36709=DIRECTION ( 'NONE',  ( -1.000000000000000000, 0.000000000000000000, 0.000000000000000000 ) ) ;
#36721=ORIENTED_EDGE ( 'NONE', *, *, #24518, .F. ) ;
#36723=AXIS2_PLACEMENT_3D ( 'NONE', #32284, #32816, #35715 ) ;
#36725=CARTESIAN_POINT ( 'NONE',  ( -330.4913330509368166, -167.9936954712156023, -38.74998146212117689 ) ) ;
#36726=DIRECTION ( 'NONE',  ( 0.000000000000000000, 0.000000000000000000, 1.000000000000000000 ) ) ;
#36727=DIRECTION ( 'NONE',  ( 1.000000000000000000, 0.000000000000000000, 0.000000000000000000 ) ) ;
#36730=ORIENTED_EDGE ( 'NONE', *, *, #30628, .T. ) ;
#36731=ORIENTED_EDGE ( 'NONE', *, *, #4181, .T. ) ;
#36733=DIRECTION ( 'NONE',  ( 0.000000000000000000, 0.000000000000000000, 1.000000000000000000 ) ) ;
#36736=CIRCLE ( 'NONE', #14090, 60.00000000000000000 ) ;
#36737=ADVANCED_FACE ( 'NONE', ( #9661 ), #45168, .T. ) ;
#36738=VERTEX_POINT ( 'NONE', #48585 ) ;
#36746=VERTEX_POINT ( 'NONE', #4682 ) ;
#36748=DIRECTION ( 'NONE',  ( 0.000000000000000000, -0.3546048870425267951, 0.9350162426854181641 ) ) ;
#36749=ORIENTED_EDGE ( 'NONE', *, *, #49963, .F. ) ;
#36754=ORIENTED_EDGE ( 'NONE', *, *, #51100, .T. ) ;
#36760=CARTESIAN_POINT ( 'NONE',  ( -339.1964088526558498, -108.8949048983204051, 57.16590939599314680 ) ) ;
#36761=ORIENTED_EDGE ( 'NONE', *, *, #50938, .F. ) ;
#36763=AXIS2_PLACEMENT_3D ( 'NONE', #39623, #12028, #208 ) ;
#36768=CARTESIAN_POINT ( 'NONE',  ( -336.3521761649654422, -135.0638248728647852, 57.91551518289418254 ) ) ;
#36769=DIRECTION ( 'NONE',  ( 1.000000000000000000, 4.952603889764026625E-17, 7.175085443855094401E-17 ) ) ;
#36771=CARTESIAN_POINT ( 'NONE',  ( -336.3521761649654422, -107.7955183043589500, 56.89493493766750731 ) ) ;
#36783=AXIS2_PLACEMENT_3D ( 'NONE', #12081, #24447, #36525 ) ;
#36786=VERTEX_POINT ( 'NONE', #21755 ) ;
#36789=AXIS2_PLACEMENT_3D ( 'NONE', #39613, #35423, #19157 ) ;
#36791=CARTESIAN_POINT ( 'NONE',  ( -339.1964088526558498, -64.86990808808704401, 6.615309698014191220 ) ) ;
#36803=EDGE_CURVE ( 'NONE', #44752, #39919, #5215, .T. ) ;
#36804=EDGE_CURVE ( 'NONE', #6572, #51893, #49612, .T. ) ;
#36805=PLANE ( 'NONE',  #22638 ) ;
#36820=LINE ( 'NONE', #48913, #14948 ) ;
#36821=CARTESIAN_POINT ( 'NONE',  ( -330.4913330509368166, -162.9117225908385365, 45.24064679492094143 ) ) ;
#36824=ADVANCED_FACE ( 'NONE', ( #29622 ), #8879, .F. ) ;
#36834=EDGE_CURVE ( 'NONE', #42669, #47727, #25433, .T. ) ;
#36837=VECTOR ( 'NONE', #36693, 1000.000000000000000 ) ;
#36840=CARTESIAN_POINT ( 'NONE',  ( -336.3521761649654422, -72.01665693856799066, -28.86398714850468039 ) ) ;
#36844=FACE_OUTER_BOUND ( 'NONE', #945, .T. ) ;
#36845=DIRECTION ( 'NONE',  ( -1.000000000000000000, 0.000000000000000000, -0.000000000000000000 ) ) ;
#36847=DIRECTION ( 'NONE',  ( -0.9063077870366494926, 5.175581015019669255E-17, -0.4226182617407002740 ) ) ;
#36862=EDGE_CURVE ( 'NONE', #42377, #20555, #36508, .T. ) ;
#36864=DIRECTION ( 'NONE',  ( 0.000000000000000000, 0.3546048870425300148, -0.9350162426854169428 ) ) ;
#36867=ORIENTED_EDGE ( 'NONE', *, *, #35945, .T. ) ;
#36870=DIRECTION ( 'NONE',  ( 1.000000000000000000, -0.000000000000000000, 0.000000000000000000 ) ) ;
#36872=EDGE_LOOP ( 'NONE', ( #42835, #12324, #47735, #51464 ) ) ;
#36873=ADVANCED_FACE ( 'NONE', ( #32305 ), #4212, .F. ) ;
#36875=ORIENTED_EDGE ( 'NONE', *, *, #27407, .F. ) ;
#36877=ORIENTED_EDGE ( 'NONE', *, *, #23117, .T. ) ;
#36878=CARTESIAN_POINT ( 'NONE',  ( -332.3517673607765914, -161.4024510877913485, 45.24454186338643780 ) ) ;
#36879=EDGE_CURVE ( 'NONE', #51152, #22837, #17087, .T. ) ;
#36888=VECTOR ( 'NONE', #26169, 1000.000000000000000 ) ;
#36890=DIRECTION ( 'NONE',  ( 1.000000000000000000, -0.000000000000000000, 0.000000000000000000 ) ) ;
#36900=EDGE_LOOP ( 'NONE', ( #28366, #50617, #23606, #8519 ) ) ;
#36906=FACE_OUTER_BOUND ( 'NONE', #48958, .T. ) ;
#36909=EDGE_LOOP ( 'NONE', ( #25194, #26022, #39295, #7185 ) ) ;
#36910=DIRECTION ( 'NONE',  ( -0.000000000000000000, 0.000000000000000000, 1.000000000000000000 ) ) ;
#36912=ORIENTED_EDGE ( 'NONE', *, *, #31391, .F. ) ;
#36913=FACE_OUTER_BOUND ( 'NONE', #2820, .T. ) ;
#36914=LINE ( 'NONE', #49006, #18614 ) ;
#36918=EDGE_CURVE ( 'NONE', #42898, #47538, #12862, .T. ) ;
#36919=CARTESIAN_POINT ( 'NONE',  ( -305.0000000000000568, -65.12585595286530804, -13.87297036558380725 ) ) ;
#36923=ORIENTED_EDGE ( 'NONE', *, *, #1105, .F. ) ;
#36926=EDGE_CURVE ( 'NONE', #49023, #49872, #21015, .T. ) ;
#36929=DIRECTION ( 'NONE',  ( 0.000000000000000000, 0.8229838658936556861, -0.5680647467311569221 ) ) ;
#36934=ORIENTED_EDGE ( 'NONE', *, *, #18127, .T. ) ;
#36936=PLANE ( 'NONE',  #10087 ) ;
#36938=FACE_BOUND ( 'NONE', #36696, .T. ) ;
#36939=DIRECTION ( 'NONE',  ( 0.000000000000000000, -0.8854560256532062468, 0.4647231720437755564 ) ) ;
#36941=AXIS2_PLACEMENT_3D ( 'NONE', #1708, #49291, #45096 ) ;
#36942=AXIS2_PLACEMENT_3D ( 'NONE', #21669, #29786, #45586 ) ;
#36947=ADVANCED_FACE ( 'NONE', ( #18379 ), #14431, .T. ) ;
#36954=PLANE ( 'NONE',  #45203 ) ;
#36958=CARTESIAN_POINT ( 'NONE',  ( -339.1964088526558498, -64.99044476834235695, 7.608018572112245970 ) ) ;
#36961=CARTESIAN_POINT ( 'NONE',  ( -336.3521761649654422, -67.40061919120938683, 18.46045550523129819 ) ) ;
#36972=PLANE ( 'NONE',  #20240 ) ;
#36976=VECTOR ( 'NONE', #37055, 1000.000000000000000 ) ;
#36979=FACE_OUTER_BOUND ( 'NONE', #11662, .T. ) ;
#36980=DIRECTION ( 'NONE',  ( -1.000000000000000000, 0.000000000000000000, -0.000000000000000000 ) ) ;
#36982=EDGE_CURVE ( 'NONE', #13514, #17674, #37295, .T. ) ;
#36996=LINE ( 'NONE', #16251, #23103 ) ;
#36998=PLANE ( 'NONE',  #34904 ) ;
#36999=CARTESIAN_POINT ( 'NONE',  ( -330.4913330509368166, -123.5000000000000284, 0.000000000000000000 ) ) ;
#37001=ORIENTED_EDGE ( 'NONE', *, *, #20080, .F. ) ;
#37005=CARTESIAN_POINT ( 'NONE',  ( -332.3517673607765914, -123.5000000000000284, 0.000000000000000000 ) ) ;
#37008=CARTESIAN_POINT ( 'NONE',  ( 0.000000000000000000, -167.6621341420952547, -39.12423683620669124 ) ) ;
#37010=DIRECTION ( 'NONE',  ( 1.000000000000000000, -0.000000000000000000, -0.000000000000000000 ) ) ;
#37011=ORIENTED_EDGE ( 'NONE', *, *, #8357, .T. ) ;
#37014=ORIENTED_EDGE ( 'NONE', *, *, #27919, .F. ) ;
#37017=CARTESIAN_POINT ( 'NONE',  ( -336.3521761649654422, -173.5513585866778214, -31.34948880313881503 ) ) ;
#37019=EDGE_LOOP ( 'NONE', ( #3530, #17939, #50280, #43449 ) ) ;
#37020=LINE ( 'NONE', #44654, #4591 ) ;
#37022=CARTESIAN_POINT ( 'NONE',  ( -339.1964088526558498, -96.06030588028492900, -53.35787839313396574 ) ) ;
#37023=DIRECTION ( 'NONE',  ( 1.043714542225393065E-14, -0.9709418174260511236, 0.2393156642875615969 ) ) ;
#37026=VERTEX_POINT ( 'NONE', #25737 ) ;
#37027=AXIS2_PLACEMENT_3D ( 'NONE', #44488, #20300, #36331 ) ;
#37029=CARTESIAN_POINT ( 'NONE',  ( -332.3517673607765914, -68.91285928486892942, -22.44790492310182017 ) ) ;
#37038=AXIS2_PLACEMENT_3D ( 'NONE', #31664, #12200, #11422 ) ;
#37040=DIRECTION ( 'NONE',  ( 0.000000000000000000, 0.7485107481711024136, 0.6631226582407937498 ) ) ;
#37041=EDGE_CURVE ( 'NONE', #8674, #33846, #10000, .T. ) ;
#37051=CARTESIAN_POINT ( 'NONE',  ( -336.3521761649654422, -140.1754235130667610, -56.65561927338005432 ) ) ;
#37052=EDGE_CURVE ( 'NONE', #44562, #15649, #49911, .T. ) ;
#37054=PLANE ( 'NONE',  #50334 ) ;
#37055=DIRECTION ( 'NONE',  ( -1.000000000000000000, -9.758900497077161467E-15, -3.701062773504848780E-15 ) ) ;
#37058=ORIENTED_EDGE ( 'NONE', *, *, #49430, .F. ) ;
#37065=CARTESIAN_POINT ( 'NONE',  ( -330.4913330509368166, -102.1108035431478811, -54.98865587491830809 ) ) ;
#37068=ORIENTED_EDGE ( 'NONE', *, *, #5627, .T. ) ;
#37074=CARTESIAN_POINT ( 'NONE',  ( -336.3521761649654422, -110.9652333097088217, -57.67619951860654481 ) ) ;
#37083=PLANE ( 'NONE',  #13695 ) ;
#37084=ORIENTED_EDGE ( 'NONE', *, *, #21867, .F. ) ;
#37091=LINE ( 'NONE', #44207, #5310 ) ;
#37092=EDGE_CURVE ( 'NONE', #1505, #20926, #46240, .T. ) ;
#37094=VECTOR ( 'NONE', #50073, 1000.000000000000114 ) ;
#37097=DIRECTION ( 'NONE',  ( 0.000000000000000000, 0.1205366802553164696, -0.9927088740980548609 ) ) ;
#37101=ADVANCED_FACE ( 'NONE', ( #13646 ), #6282, .F. ) ;
#37103=EDGE_CURVE ( 'NONE', #4967, #2171, #15204, .T. ) ;
#37105=CARTESIAN_POINT ( 'NONE',  ( -330.4913330509368166, -101.7569374291128526, -55.92172413327835301 ) ) ;
#37106=ORIENTED_EDGE ( 'NONE', *, *, #22659, .F. ) ;
#37114=ORIENTED_EDGE ( 'NONE', *, *, #28073, .T. ) ;
#37115=VECTOR ( 'NONE', #5320, 1000.000000000000000 ) ;
#37117=CARTESIAN_POINT ( 'NONE',  ( -332.3517673607765914, -121.8677111499054320, 59.00000000000001421 ) ) ;
#37118=ORIENTED_EDGE ( 'NONE', *, *, #2401, .F. ) ;
#37119=DIRECTION ( 'NONE',  ( -1.000000000000000000, -0.000000000000000000, 0.000000000000000000 ) ) ;
#37121=FACE_OUTER_BOUND ( 'NONE', #18625, .T. ) ;
#37128=VERTEX_POINT ( 'NONE', #7572 ) ;
#37129=VECTOR ( 'NONE', #34120, 1000.000000000000227 ) ;
#37131=AXIS2_PLACEMENT_3D ( 'NONE', #11576, #15261, #7388 ) ;
#37137=ORIENTED_EDGE ( 'NONE', *, *, #35249, .T. ) ;
#37138=DIRECTION ( 'NONE',  ( 0.000000000000000000, -0.6631226582408016323, -0.7485107481710953081 ) ) ;
#37140=DIRECTION ( 'NONE',  ( -0.000000000000000000, -0.9709418174260526779, -0.2393156642875547968 ) ) ;
#37141=ORIENTED_EDGE ( 'NONE', *, *, #45998, .T. ) ;
#37150=EDGE_CURVE ( 'NONE', #28257, #39885, #50686, .T. ) ;
#37152=DIRECTION ( 'NONE',  ( -0.000000000000000000, 0.000000000000000000, 1.000000000000000000 ) ) ;
#37153=EDGE_CURVE ( 'NONE', #2629, #41896, #35673, .T. ) ;
#37154=FACE_OUTER_BOUND ( 'NONE', #47138, .T. ) ;
#37158=ORIENTED_EDGE ( 'NONE', *, *, #9191, .F. ) ;
#37162=EDGE_LOOP ( 'NONE', ( #16671, #37661, #36867, #17891 ) ) ;
#37166=EDGE_CURVE ( 'NONE', #32221, #34468, #23082, .T. ) ;
#37168=CIRCLE ( 'NONE', #29621, 60.00000000000000000 ) ;
#37170=CARTESIAN_POINT ( 'NONE',  ( -339.1964088526558498, -66.09477493971894546, 13.63415328425207917 ) ) ;
#37172=VECTOR ( 'NONE', #49135, 1000.000000000000000 ) ;
#37175=EDGE_CURVE ( 'NONE', #29243, #51040, #43052, .T. ) ;
#37176=DIRECTION ( 'NONE',  ( -0.000000000000000000, 0.1205366802553199113, -0.9927088740980544168 ) ) ;
#37180=EDGE_CURVE ( 'NONE', #51893, #15715, #27269, .T. ) ;
#37181=CARTESIAN_POINT ( 'NONE',  ( -305.0000000000000568, -168.0775241366801254, -40.16023333900968595 ) ) ;
#37186=DIRECTION ( 'NONE',  ( 1.043714542225393381E-14, 0.7485107481711069655, 0.6631226582407885317 ) ) ;
#37188=FACE_BOUND ( 'NONE', #46140, .T. ) ;
#37196=ORIENTED_EDGE ( 'NONE', *, *, #37153, .T. ) ;
#37200=PLANE ( 'NONE',  #9533 ) ;
#37204=VECTOR ( 'NONE', #27227, 1000.000000000000000 ) ;
#37207=ORIENTED_EDGE ( 'NONE', *, *, #428, .F. ) ;
#37209=AXIS2_PLACEMENT_3D ( 'NONE', #49041, #12755, #9358 ) ;
#37210=DIRECTION ( 'NONE',  ( 0.000000000000000000, 0.000000000000000000, 1.000000000000000000 ) ) ;
#37212=EDGE_CURVE ( 'NONE', #13145, #10439, #51466, .T. ) ;
#37215=EDGE_CURVE ( 'NONE', #39568, #43845, #6662, .T. ) ;
#37216=DIRECTION ( 'NONE',  ( -0.000000000000000000, -0.5680647467311596976, -0.8229838658936536877 ) ) ;
#37217=LINE ( 'NONE', #1207, #11951 ) ;
#37220=CARTESIAN_POINT ( 'NONE',  ( -339.1964088526558498, -68.51134412508150717, 21.38919645685156112 ) ) ;
#37221=CARTESIAN_POINT ( 'NONE',  ( -336.3521761649654422, -85.72124494520284088, -46.61293454085073051 ) ) ;
#37226=EDGE_CURVE ( 'NONE', #29243, #44016, #35947, .T. ) ;
#37231=ORIENTED_EDGE ( 'NONE', *, *, #36096, .F. ) ;
#37232=DIRECTION ( 'NONE',  ( 0.000000000000000000, 0.7485107481710977506, -0.6631226582407989678 ) ) ;
#37234=ORIENTED_EDGE ( 'NONE', *, *, #31571, .T. ) ;
#37238=EDGE_CURVE ( 'NONE', #3919, #22737, #972, .T. ) ;
#37239=CARTESIAN_POINT ( 'NONE',  ( -339.1964088526558498, -137.1341532842531876, -57.40522506028080585 ) ) ;
#37240=CARTESIAN_POINT ( 'NONE',  ( -365.0000000000001137, -78.50000000000002842, 10.00000000000000711 ) ) ;
#37244=AXIS2_PLACEMENT_3D ( 'NONE', #22131, #22390, #45535 ) ;
#37246=ORIENTED_EDGE ( 'NONE', *, *, #1812, .F. ) ;
#37252=DIRECTION ( 'NONE',  ( 0.000000000000000000, 0.2393156642875516049, -0.9709418174260534551 ) ) ;
#37257=DIRECTION ( 'NONE',  ( 0.000000000000000000, -0.6631226582407989678, -0.7485107481710977506 ) ) ;
#37259=CARTESIAN_POINT ( 'NONE',  ( -305.0000000000000568, -65.36517161715278235, -14.84391218300951643 ) ) ;
#37269=CARTESIAN_POINT ( 'NONE',  ( -339.1964088526558498, -66.33409060400673241, -14.60509510167901404 ) ) ;
#37275=CARTESIAN_POINT ( 'NONE',  ( -339.1964088526558498, -123.5000000000000284, 0.000000000000000000 ) ) ;
#37277=CARTESIAN_POINT ( 'NONE',  ( -339.1964088526558498, -71.02573290043878274, -26.97593913775585506 ) ) ;
#37284=CARTESIAN_POINT ( 'NONE',  ( -336.3521761649654422, -64.73342574900661361, 5.491276508483657892 ) ) ;
#37286=DIRECTION ( 'NONE',  ( 0.000000000000000000, 0.5680647467311510379, -0.8229838658936596829 ) ) ;
#37289=CARTESIAN_POINT ( 'NONE',  ( -332.3517673607765914, -65.24746378767824240, -9.724760635741734660 ) ) ;
#37292=ORIENTED_EDGE ( 'NONE', *, *, #15006, .F. ) ;
#37293=CARTESIAN_POINT ( 'NONE',  ( -332.3517673607765914, -181.7525362123217292, 9.724760635742144999 ) ) ;
#37295=LINE ( 'NONE', #26236, #13369 ) ;
#37296=PLANE ( 'NONE',  #24507 ) ;
#37301=VERTEX_POINT ( 'NONE', #48566 ) ;
#37303=PLANE ( 'NONE',  #19078 ) ;
#37305=VERTEX_POINT ( 'NONE', #12546 ) ;
#37309=ORIENTED_EDGE ( 'NONE', *, *, #5373, .T. ) ;
#37311=ORIENTED_EDGE ( 'NONE', *, *, #17002, .T. ) ;
#37313=VERTEX_POINT ( 'NONE', #36725 ) ;
#37314=AXIS2_PLACEMENT_3D ( 'NONE', #40335, #35900, #31430 ) ;
#37318=VERTEX_POINT ( 'NONE', #16770 ) ;
#37319=CARTESIAN_POINT ( 'NONE',  ( -330.4913330509368166, -162.2499814621216672, -44.49369547121515467 ) ) ;
#37320=LINE ( 'NONE', #9998, #49102 ) ;
#37322=CARTESIAN_POINT ( 'NONE',  ( -336.3521761649654422, -152.3639871485048900, -51.48334306143194539 ) ) ;
#37327=DIRECTION ( 'NONE',  ( 1.000000000000000000, -0.000000000000000000, -0.000000000000000000 ) ) ;
#37329=ORIENTED_EDGE ( 'NONE', *, *, #3766, .T. ) ;
#37333=DIRECTION ( 'NONE',  ( -1.000000000000000000, -0.000000000000000000, -0.000000000000000000 ) ) ;
#37334=ORIENTED_EDGE ( 'NONE', *, *, #28564, .T. ) ;
#37338=VECTOR ( 'NONE', #49105, 999.9999999999998863 ) ;
#37342=ADVANCED_FACE ( 'NONE', ( #4935 ), #12793, .F. ) ;
#37343=DIRECTION ( 'NONE',  ( -0.000000000000000000, -0.9927088740980534176, 0.1205366802553268502 ) ) ;
#37347=ORIENTED_EDGE ( 'NONE', *, *, #41539, .T. ) ;
#37348=CARTESIAN_POINT ( 'NONE',  ( -330.4913330509368166, -131.1080185721132807, -58.50955523165751515 ) ) ;
#37359=PLANE ( 'NONE',  #46402 ) ;
#37360=PLANE ( 'NONE',  #41289 ) ;
#37364=PLANE ( 'NONE',  #5329 ) ;
#37371=AXIS2_PLACEMENT_3D ( 'NONE', #2747, #37779, #38997 ) ;
#37372=VECTOR ( 'NONE', #12256, 1000.000000000000114 ) ;
#37376=VERTEX_POINT ( 'NONE', #5452 ) ;
#37384=DIRECTION ( 'NONE',  ( 0.000000000000000000, -1.000000000000000000, 1.047444401652940007E-14 ) ) ;
#37385=ORIENTED_EDGE ( 'NONE', *, *, #37938, .F. ) ;
#37389=DIRECTION ( 'NONE',  ( 0.000000000000000000, -0.3546048870425331789, 0.9350162426854158326 ) ) ;
#37397=CARTESIAN_POINT ( 'NONE',  ( -336.3521761649654422, -155.3847370087607374, 50.82679948493869659 ) ) ;
#37398=ORIENTED_EDGE ( 'NONE', *, *, #22999, .F. ) ;
#37402=CARTESIAN_POINT ( 'NONE',  ( -330.4913330509368166, -123.5000000000000284, 0.000000000000000000 ) ) ;
#37406=ADVANCED_FACE ( 'NONE', ( #17544 ), #37491, .F. ) ;
#37409=VERTEX_POINT ( 'NONE', #30128 ) ;
#37413=DIRECTION ( 'NONE',  ( -1.000000000000000000, 1.036104688092337311E-14, 1.258058860540426107E-15 ) ) ;
#37417=ORIENTED_EDGE ( 'NONE', *, *, #8033, .F. ) ;
#37421=CARTESIAN_POINT ( 'NONE',  ( -305.0000000000000568, -106.5990858529439578, 57.57047073799066794 ) ) ;
#37422=CARTESIAN_POINT ( 'NONE',  ( -336.3521761649654422, -83.15397741537739762, 43.07972642080338233 ) ) ;
#37426=DIRECTION ( 'NONE',  ( 0.000000000000000000, 0.000000000000000000, -1.000000000000000000 ) ) ;
#37429=DIRECTION ( 'NONE',  ( -0.000000000000000000, -0.6631226582407885317, 0.7485107481711069655 ) ) ;
#37432=ORIENTED_EDGE ( 'NONE', *, *, #15267, .T. ) ;
#37434=LINE ( 'NONE', #13275, #50192 ) ;
#37436=DIRECTION ( 'NONE',  ( 0.000000000000000000, 0.000000000000000000, -1.000000000000000000 ) ) ;
#37438=EDGE_LOOP ( 'NONE', ( #48089, #41511, #9799, #26400 ) ) ;
#37439=ORIENTED_EDGE ( 'NONE', *, *, #34702, .T. ) ;
#37440=CARTESIAN_POINT ( 'NONE',  ( -339.1964088526558498, -90.39567187580801999, 48.84008046109089918 ) ) ;
#37451=ORIENTED_EDGE ( 'NONE', *, *, #48642, .T. ) ;
#37452=CARTESIAN_POINT ( 'NONE',  ( -332.3517673607765914, -65.58448481710581746, 11.56382487286456140 ) ) ;
#37458=CIRCLE ( 'NONE', #12277, 60.00000000000000000 ) ;
#37459=FACE_OUTER_BOUND ( 'NONE', #24233, .T. ) ;
#37460=VECTOR ( 'NONE', #47260, 999.9999999999998863 ) ;
#37463=LINE ( 'NONE', #33532, #19245 ) ;
#37465=EDGE_CURVE ( 'NONE', #41706, #3626, #46132, .T. ) ;
#37468=ORIENTED_EDGE ( 'NONE', *, *, #44731, .F. ) ;
#37471=EDGE_LOOP ( 'NONE', ( #46767, #2092, #40881, #45429 ) ) ;
#37472=FACE_OUTER_BOUND ( 'NONE', #3951, .T. ) ;
#37473=EDGE_CURVE ( 'NONE', #6572, #29121, #45398, .T. ) ;
#37478=FACE_OUTER_BOUND ( 'NONE', #7004, .T. ) ;
#37481=DIRECTION ( 'NONE',  ( 0.000000000000000000, 0.9350162426854121689, -0.3546048870425426158 ) ) ;
#37483=ORIENTED_EDGE ( 'NONE', *, *, #44292, .F. ) ;
#37484=VECTOR ( 'NONE', #31016, 1000.000000000000227 ) ;
#37485=CIRCLE ( 'NONE', #14013, 60.00000000000000000 ) ;
#37487=AXIS2_PLACEMENT_3D ( 'NONE', #25011, #21059, #16868 ) ;
#37489=CARTESIAN_POINT ( 'NONE',  ( -336.3521761649654422, -164.5945333327934463, -42.41660376256285048 ) ) ;
#37491=PLANE ( 'NONE',  #44465 ) ;
#37493=LINE ( 'NONE', #5964, #18410 ) ;
#37497=VECTOR ( 'NONE', #26597, 1000.000000000000114 ) ;
#37498=AXIS2_PLACEMENT_3D ( 'NONE', #15069, #35785, #39467 ) ;
#37502=VERTEX_POINT ( 'NONE', #9132 ) ;
#37506=DIRECTION ( 'NONE',  ( -1.000000000000000000, 0.000000000000000000, 0.000000000000000000 ) ) ;
#37508=EDGE_LOOP ( 'NONE', ( #28428, #10479, #35699, #46869 ) ) ;
#37520=CARTESIAN_POINT ( 'NONE',  ( -339.1964088526558498, -182.0095552316575152, 7.608018572113563138 ) ) ;
#37524=VECTOR ( 'NONE', #18938, 1000.000000000000000 ) ;
#37530=VECTOR ( 'NONE', #19360, 999.9999999999998863 ) ;
#37533=ORIENTED_EDGE ( 'NONE', *, *, #42577, .T. ) ;
#37534=EDGE_CURVE ( 'NONE', #18800, #16080, #31154, .T. ) ;
#37537=EDGE_CURVE ( 'NONE', #27045, #8870, #31022, .T. ) ;
#37538=VERTEX_POINT ( 'NONE', #42736 ) ;
#37543=VECTOR ( 'NONE', #11318, 1000.000000000000000 ) ;
#37558=VECTOR ( 'NONE', #51759, 1000.000000000000114 ) ;
#37560=VERTEX_POINT ( 'NONE', #27470 ) ;
#37564=CARTESIAN_POINT ( 'NONE',  ( -305.0000000000000568, -74.40671499923421095, -34.49419324804659936 ) ) ;
#37567=VECTOR ( 'NONE', #48468, 1000.000000000000000 ) ;
#37571=DIRECTION ( 'NONE',  ( 0.000000000000000000, -0.8229838658936494689, 0.5680647467311658039 ) ) ;
#37572=LINE ( 'NONE', #49660, #6938 ) ;
#37574=FACE_OUTER_BOUND ( 'NONE', #46984, .T. ) ;
#37578=EDGE_LOOP ( 'NONE', ( #47053, #3431, #47752, #28619 ) ) ;
#37579=LINE ( 'NONE', #13657, #50239 ) ;
#37580=CIRCLE ( 'NONE', #9072, 5.000000000000001776 ) ;
#37583=VECTOR ( 'NONE', #23507, 1000.000000000000000 ) ;
#37584=ADVANCED_FACE ( 'NONE', ( #7248 ), #42463, .F. ) ;
#37585=EDGE_LOOP ( 'NONE', ( #45872, #7272, #45405, #38751 ) ) ;
#37587=ADVANCED_FACE ( 'NONE', ( #39304 ), #3306, .F. ) ;
#37588=AXIS2_PLACEMENT_3D ( 'NONE', #33406, #13419, #8694 ) ;
#37592=VERTEX_POINT ( 'NONE', #30371 ) ;
#37595=EDGE_LOOP ( 'NONE', ( #27461, #14645, #52033, #680 ) ) ;
#37597=ORIENTED_EDGE ( 'NONE', *, *, #25078, .F. ) ;
#37598=FACE_OUTER_BOUND ( 'NONE', #18082, .T. ) ;
#37615=PLANE ( 'NONE',  #37487 ) ;
#37618=CARTESIAN_POINT ( 'NONE',  ( -365.0000000000001137, -78.50000000000002842, -10.00000000000000711 ) ) ;
#37621=VERTEX_POINT ( 'NONE', #44804 ) ;
#37622=VECTOR ( 'NONE', #7947, 1000.000000000000000 ) ;
#37626=PLANE ( 'NONE',  #51792 ) ;
#37634=DIRECTION ( 'NONE',  ( -1.000000000000000000, 0.000000000000000000, 0.000000000000000000 ) ) ;
#37638=EDGE_LOOP ( 'NONE', ( #26261, #28316, #47335, #49771 ) ) ;
#37639=VECTOR ( 'NONE', #37138, 1000.000000000000114 ) ;
#37661=ORIENTED_EDGE ( 'NONE', *, *, #625, .T. ) ;
#37662=EDGE_LOOP ( 'NONE', ( #49376, #37417, #27948, #28240 ) ) ;
#37666=EDGE_CURVE ( 'NONE', #13356, #5376, #40317, .T. ) ;
#37668=ORIENTED_EDGE ( 'NONE', *, *, #42632, .T. ) ;
#37669=LINE ( 'NONE', #33478, #8257 ) ;
#37671=EDGE_CURVE ( 'NONE', #31250, #21618, #16173, .T. ) ;
#37673=CARTESIAN_POINT ( 'NONE',  ( -339.1964088526558498, -115.8919814278871598, -58.50955523165758621 ) ) ;
#37674=VERTEX_POINT ( 'NONE', #7761 ) ;
#37679=LINE ( 'NONE', #2455, #20196 ) ;
#37683=CARTESIAN_POINT ( 'NONE',  ( -339.1964088526558498, -123.5000000000000284, 0.000000000000000000 ) ) ;
#37684=FACE_OUTER_BOUND ( 'NONE', #40738, .T. ) ;
#37688=LINE ( 'NONE', #10090, #1046 ) ;
#37689=ORIENTED_EDGE ( 'NONE', *, *, #44672, .T. ) ;
#37694=ORIENTED_EDGE ( 'NONE', *, *, #44001, .T. ) ;
#37698=DIRECTION ( 'NONE',  ( -0.000000000000000000, -0.1205366802553268363, -0.9927088740980534176 ) ) ;
#37699=ORIENTED_EDGE ( 'NONE', *, *, #1257, .T. ) ;
#37701=ORIENTED_EDGE ( 'NONE', *, *, #13788, .F. ) ;
#37704=EDGE_CURVE ( 'NONE', #36128, #41126, #20359, .T. ) ;
#37705=EDGE_CURVE ( 'NONE', #45751, #47856, #32712, .T. ) ;
#37711=DIRECTION ( 'NONE',  ( 1.000000000000000000, -0.000000000000000000, -0.000000000000000000 ) ) ;
#37713=EDGE_CURVE ( 'NONE', #34468, #33439, #32454, .T. ) ;
#37714=VECTOR ( 'NONE', #48822, 1000.000000000000000 ) ;
#37720=FACE_OUTER_BOUND ( 'NONE', #4394, .T. ) ;
#37722=ORIENTED_EDGE ( 'NONE', *, *, #4594, .T. ) ;
#37723=FACE_OUTER_BOUND ( 'NONE', #27751, .T. ) ;
#37724=ADVANCED_FACE ( 'NONE', ( #35609 ), #40845, .F. ) ;
#37725=CARTESIAN_POINT ( 'NONE',  ( 0.000000000000000000, -144.4216883355098844, -55.16595831843940090 ) ) ;
#37726=DIRECTION ( 'NONE',  ( 0.000000000000000000, 1.669960466207006380E-13, -1.000000000000000000 ) ) ;
#37730=VERTEX_POINT ( 'NONE', #39798 ) ;
#37735=VERTEX_POINT ( 'NONE', #24056 ) ;
#37737=PLANE ( 'NONE',  #43117 ) ;
#37738=CARTESIAN_POINT ( 'NONE',  ( -339.1964088526558498, -178.8432607619606358, 20.45418021416736565 ) ) ;
#37742=ORIENTED_EDGE ( 'NONE', *, *, #7285, .F. ) ;
#37744=DIRECTION ( 'NONE',  ( 1.000000000000000000, -0.000000000000000000, -0.000000000000000000 ) ) ;
#37745=ORIENTED_EDGE ( 'NONE', *, *, #42332, .T. ) ;
#37752=CARTESIAN_POINT ( 'NONE',  ( -336.3521761649653854, -125.1322888500942554, -59.97779283292990016 ) ) ;
#37756=CARTESIAN_POINT ( 'NONE',  ( -305.0000000000000568, -163.6602333390099773, -44.57752413667984825 ) ) ;
#37759=EDGE_CURVE ( 'NONE', #50461, #16663, #32961, .T. ) ;
#37760=VECTOR ( 'NONE', #23548, 1000.000000000000000 ) ;
#37761=CIRCLE ( 'NONE', #20128, 60.00000000000000000 ) ;
#37763=DIRECTION ( 'NONE',  ( -0.000000000000000000, -0.2393156642875615969, -0.9709418174260511236 ) ) ;
#37764=DIRECTION ( 'NONE',  ( -0.000000000000000000, 0.6631226582407863113, -0.7485107481711089639 ) ) ;
#37767=CARTESIAN_POINT ( 'NONE',  ( -332.3517673607765914, -65.82380048139334860, 12.53476669029061519 ) ) ;
#37769=ORIENTED_EDGE ( 'NONE', *, *, #36602, .F. ) ;
#37772=ORIENTED_EDGE ( 'NONE', *, *, #24077, .F. ) ;
#37776=VECTOR ( 'NONE', #44150, 1000.000000000000000 ) ;
#37778=DIRECTION ( 'NONE',  ( -1.000000000000000000, 0.000000000000000000, 0.000000000000000000 ) ) ;
#37779=DIRECTION ( 'NONE',  ( -1.000000000000000000, 0.000000000000000000, 0.000000000000000000 ) ) ;
#37781=DIRECTION ( 'NONE',  ( -1.000000000000000000, 0.000000000000000000, 0.000000000000000000 ) ) ;
#37785=ORIENTED_EDGE ( 'NONE', *, *, #20745, .F. ) ;
#37788=CARTESIAN_POINT ( 'NONE',  ( -339.1964088526558498, -123.0000000000002700, -59.00000000000002132 ) ) ;
#37789=LINE ( 'NONE', #41469, #17997 ) ;
#37796=ORIENTED_EDGE ( 'NONE', *, *, #50629, .T. ) ;
#37803=EDGE_LOOP ( 'NONE', ( #25466, #30385, #10835, #7002 ) ) ;
#37805=ADVANCED_FACE ( 'NONE', ( #49276 ), #14243, .T. ) ;
#37806=DIRECTION ( 'NONE',  ( -1.000000000000000000, -0.000000000000000000, -0.000000000000000000 ) ) ;
#37817=DIRECTION ( 'NONE',  ( -0.000000000000000000, -0.9709418174260534551, -0.2393156642875516327 ) ) ;
#37825=CARTESIAN_POINT ( 'NONE',  ( -339.1964088526558498, -182.0095552316575152, 7.608018572113563138 ) ) ;
#37826=EDGE_LOOP ( 'NONE', ( #43581, #3532, #49988, #50254 ) ) ;
#37832=AXIS2_PLACEMENT_3D ( 'NONE', #17468, #21911, #38696 ) ;
#37833=EDGE_CURVE ( 'NONE', #21855, #10851, #18697, .T. ) ;
#37840=DIRECTION ( 'NONE',  ( 1.000000000000000000, -0.000000000000000000, -0.000000000000000000 ) ) ;
#37841=ORIENTED_EDGE ( 'NONE', *, *, #9974, .T. ) ;
#37842=CARTESIAN_POINT ( 'NONE',  ( -339.1964088526558498, -66.33409060400650503, 14.60509510167813474 ) ) ;
#37843=ORIENTED_EDGE ( 'NONE', *, *, #21576, .F. ) ;
#37845=DIRECTION ( 'NONE',  ( 1.000000000000000000, 0.000000000000000000, 0.000000000000000000 ) ) ;
#37846=DIRECTION ( 'NONE',  ( 1.000000000000000000, 0.000000000000000000, -0.000000000000000000 ) ) ;
#37848=ORIENTED_EDGE ( 'NONE', *, *, #22689, .T. ) ;
#37849=EDGE_CURVE ( 'NONE', #43466, #29051, #30775, .T. ) ;
#37851=CARTESIAN_POINT ( 'NONE',  ( -339.1964088526558498, -145.2430625708868206, 55.92172413327848801 ) ) ;
#37855=VERTEX_POINT ( 'NONE', #46822 ) ;
#37858=CARTESIAN_POINT ( 'NONE',  ( -336.3521761649654422, -65.12692710742291524, -8.732051761643681687 ) ) ;
#37861=CARTESIAN_POINT ( 'NONE',  ( -305.0000000000000568, -176.8578783931339444, -27.43969411971521666 ) ) ;
#37863=EDGE_CURVE ( 'NONE', #35288, #12660, #46305, .T. ) ;
#37870=DIRECTION ( 'NONE',  ( -0.000000000000000000, 0.9927088740980526405, -0.1205366802553337890 ) ) ;
#37873=ADVANCED_FACE ( 'NONE', ( #23655 ), #11050, .F. ) ;
#37880=FACE_OUTER_BOUND ( 'NONE', #14124, .T. ) ;
#37883=VERTEX_POINT ( 'NONE', #6864 ) ;
#37884=VERTEX_POINT ( 'NONE', #31541 ) ;
#37885=EDGE_CURVE ( 'NONE', #12335, #41587, #22894, .T. ) ;
#37891=VECTOR ( 'NONE', #23169, 1000.000000000000000 ) ;
#37892=EDGE_CURVE ( 'NONE', #36591, #22171, #6731, .T. ) ;
#37898=VERTEX_POINT ( 'NONE', #24193 ) ;
#37900=DIRECTION ( 'NONE',  ( 1.000000000000000000, 0.000000000000000000, -0.000000000000000000 ) ) ;
#37916=ORIENTED_EDGE ( 'NONE', *, *, #12211, .T. ) ;
#37917=DIRECTION ( 'NONE',  ( 1.000000000000000000, -0.000000000000000000, -0.000000000000000000 ) ) ;
#37919=VERTEX_POINT ( 'NONE', #260 ) ;
#37921=ORIENTED_EDGE ( 'NONE', *, *, #8216, .F. ) ;
#37922=DIRECTION ( 'NONE',  ( -1.000000000000000000, -0.000000000000000000, -0.000000000000000000 ) ) ;
#37923=AXIS2_PLACEMENT_3D ( 'NONE', #27137, #51581, #23474 ) ;
#37932=DIRECTION ( 'NONE',  ( -1.000000000000000000, 0.000000000000000000, 0.000000000000000000 ) ) ;
#37934=EDGE_CURVE ( 'NONE', #41945, #47761, #47018, .T. ) ;
#37938=EDGE_CURVE ( 'NONE', #32555, #41322, #20238, .T. ) ;
#37940=VERTEX_POINT ( 'NONE', #12346 ) ;
#37941=PLANE ( 'NONE',  #37996 ) ;
#37942=ORIENTED_EDGE ( 'NONE', *, *, #15951, .F. ) ;
#37943=DIRECTION ( 'NONE',  ( 1.000000000000000000, -0.000000000000000000, 0.000000000000000000 ) ) ;
#37946=ORIENTED_EDGE ( 'NONE', *, *, #45131, .T. ) ;
#37948=VECTOR ( 'NONE', #50687, 1000.000000000000000 ) ;
#37949=PLANE ( 'NONE',  #47270 ) ;
#37950=PLANE ( 'NONE',  #36514 ) ;
#37951=EDGE_CURVE ( 'NONE', #39518, #17967, #32840, .T. ) ;
#37954=PLANE ( 'NONE',  #39251 ) ;
#37967=DIRECTION ( 'NONE',  ( 0.000000000000000000, 0.000000000000000000, 1.000000000000000000 ) ) ;
#37968=CARTESIAN_POINT ( 'NONE',  ( -330.4913330509368166, -181.6348283828470755, 14.84391218301019677 ) ) ;
#37969=ORIENTED_EDGE ( 'NONE', *, *, #28632, .F. ) ;
#37970=ORIENTED_EDGE ( 'NONE', *, *, #25103, .T. ) ;
#37971=CARTESIAN_POINT ( 'NONE',  ( -332.3517673607765914, -125.1322888500942270, -59.00000000000002132 ) ) ;
#37975=AXIS2_PLACEMENT_3D ( 'NONE', #37275, #33848, #13619 ) ;
#37976=FACE_OUTER_BOUND ( 'NONE', #20700, .T. ) ;
#37984=CARTESIAN_POINT ( 'NONE',  ( 0.000000000000000000, -123.5000000000002416, -59.00000000000002132 ) ) ;
#37985=ORIENTED_EDGE ( 'NONE', *, *, #29141, .T. ) ;
#37994=ORIENTED_EDGE ( 'NONE', *, *, #25974, .F. ) ;
#37996=AXIS2_PLACEMENT_3D ( 'NONE', #50305, #46357, #49786 ) ;
#38000=PLANE ( 'NONE',  #22110 ) ;
#38001=AXIS2_PLACEMENT_3D ( 'NONE', #49655, #25218, #41227 ) ;
#38005=LINE ( 'NONE', #2007, #12860 ) ;
#38009=PLANE ( 'NONE',  #21886 ) ;
#38010=DIRECTION ( 'NONE',  ( 1.000000000000000000, -0.000000000000000000, -0.000000000000000000 ) ) ;
#38014=ORIENTED_EDGE ( 'NONE', *, *, #264, .F. ) ;
#38015=CARTESIAN_POINT ( 'NONE',  ( -330.4913330509368166, -150.4759391377553186, 52.47426709956150859 ) ) ;
#38017=DIRECTION ( 'NONE',  ( 0.000000000000000000, -0.8229838658936596829, -0.5680647467311510379 ) ) ;
#38018=DIRECTION ( 'NONE',  ( 0.000000000000000000, 0.2393156642875516049, -0.9709418174260534551 ) ) ;
#38022=AXIS2_PLACEMENT_3D ( 'NONE', #47210, #30909, #27206 ) ;
#38026=ORIENTED_EDGE ( 'NONE', *, *, #12004, .F. ) ;
#38028=ORIENTED_EDGE ( 'NONE', *, *, #34025, .F. ) ;
#38033=ADVANCED_FACE ( 'NONE', ( #36260 ), #25227, .F. ) ;
#38042=CARTESIAN_POINT ( 'NONE',  ( -332.3517673607765914, -152.8183901354257159, -52.34913561719022113 ) ) ;
#38043=LINE ( 'NONE', #38816, #43218 ) ;
#38045=FACE_OUTER_BOUND ( 'NONE', #38567, .T. ) ;
#38046=ORIENTED_EDGE ( 'NONE', *, *, #5523, .T. ) ;
#38050=DIRECTION ( 'NONE',  ( -1.000000000000000000, 0.000000000000000000, 0.000000000000000000 ) ) ;
#38057=DIRECTION ( 'NONE',  ( 0.000000000000000000, -0.4647231720437695057, -0.8854560256532093554 ) ) ;
#38058=ORIENTED_EDGE ( 'NONE', *, *, #40118, .T. ) ;
#38065=AXIS2_PLACEMENT_3D ( 'NONE', #22146, #38157, #38931 ) ;
#38067=CARTESIAN_POINT ( 'NONE',  ( -305.0000000000000568, -63.76276212672765809, 5.609136410542458151 ) ) ;
#38068=VECTOR ( 'NONE', #41731, 1000.000000000000000 ) ;
#38071=EDGE_CURVE ( 'NONE', #38337, #40712, #9205, .T. ) ;
#38072=DIRECTION ( 'NONE',  ( -8.718379230999705894E-17, -0.6631226582407863113, 0.7485107481711089639 ) ) ;
#38073=CARTESIAN_POINT ( 'NONE',  ( -336.3521761649654422, -183.3224719910990643, -4.612141029301911388 ) ) ;
#38076=ORIENTED_EDGE ( 'NONE', *, *, #7791, .F. ) ;
#38080=VECTOR ( 'NONE', #7558, 1000.000000000000000 ) ;
#38083=PLANE ( 'NONE',  #28236 ) ;
#38088=DIRECTION ( 'NONE',  ( -0.000000000000000000, -0.7485107481711046340, -0.6631226582407911962 ) ) ;
#38094=CARTESIAN_POINT ( 'NONE',  ( -332.3517673607765914, -82.40546666720629787, 42.41660376256258047 ) ) ;
#38095=DIRECTION ( 'NONE',  ( -0.000000000000000000, -0.7485107481711024136, -0.6631226582407937498 ) ) ;
#38096=LINE ( 'NONE', #50216, #38241 ) ;
#38099=ORIENTED_EDGE ( 'NONE', *, *, #18495, .T. ) ;
#38101=VERTEX_POINT ( 'NONE', #38073 ) ;
#38102=DIRECTION ( 'NONE',  ( -0.000000000000000000, 0.9350162426854146114, -0.3546048870425363986 ) ) ;
#38104=ORIENTED_EDGE ( 'NONE', *, *, #20828, .T. ) ;
#38107=CARTESIAN_POINT ( 'NONE',  ( -305.0000000000000568, -135.2893155068536828, 58.83036664750492406 ) ) ;
#38108=CARTESIAN_POINT ( 'NONE',  ( -336.3521761649654422, -64.61288906875131488, 4.498567634385603142 ) ) ;
#38109=ORIENTED_EDGE ( 'NONE', *, *, #96, .T. ) ;
#38112=LINE ( 'NONE', #10789, #18916 ) ;
#38115=ORIENTED_EDGE ( 'NONE', *, *, #9446, .F. ) ;
#38116=ADVANCED_FACE ( 'NONE', ( #10475 ), #14437, .F. ) ;
#38120=ADVANCED_FACE ( 'NONE', ( #41497 ), #49663, .F. ) ;
#38121=VECTOR ( 'NONE', #6594, 1000.000000000000000 ) ;
#38125=CARTESIAN_POINT ( 'NONE',  ( -336.3521761649654422, -81.08339623743702873, -41.09453333279329712 ) ) ;
#38129=ORIENTED_EDGE ( 'NONE', *, *, #37103, .T. ) ;
#38134=ORIENTED_EDGE ( 'NONE', *, *, #8623, .T. ) ;
#38140=EDGE_LOOP ( 'NONE', ( #26941, #29788, #17817, #46626 ) ) ;
#38147=LINE ( 'NONE', #26845, #28071 ) ;
#38154=EDGE_CURVE ( 'NONE', #38337, #42669, #2599, .T. ) ;
#38157=DIRECTION ( 'NONE',  ( 1.000000000000000000, -0.000000000000000000, 0.000000000000000000 ) ) ;
#38158=FACE_OUTER_BOUND ( 'NONE', #34977, .T. ) ;
#38165=EDGE_CURVE ( 'NONE', #38873, #19813, #830, .T. ) ;
#38168=FACE_BOUND ( 'NONE', #23823, .T. ) ;
#38176=ORIENTED_EDGE ( 'NONE', *, *, #32348, .F. ) ;
#38179=CARTESIAN_POINT ( 'NONE',  ( -339.1964088526558498, -123.5000000000000284, 0.000000000000000000 ) ) ;
#38181=EDGE_CURVE ( 'NONE', #31995, #34413, #25480, .T. ) ;
#38186=EDGE_LOOP ( 'NONE', ( #33815, #42907, #9068, #7755 ) ) ;
#38189=AXIS2_PLACEMENT_3D ( 'NONE', #9552, #49767, #25843 ) ;
#38194=VECTOR ( 'NONE', #5749, 1000.000000000000114 ) ;
#38195=VECTOR ( 'NONE', #41603, 1000.000000000000000 ) ;
#38200=DIRECTION ( 'NONE',  ( -1.000000000000000000, 0.000000000000000000, 0.000000000000000000 ) ) ;
#38201=VERTEX_POINT ( 'NONE', #2849 ) ;
#38203=AXIS2_PLACEMENT_3D ( 'NONE', #15691, #11976, #7785 ) ;
#38212=ORIENTED_EDGE ( 'NONE', *, *, #6717, .T. ) ;
#38217=DIRECTION ( 'NONE',  ( 1.000000000000000000, -0.000000000000000000, -0.000000000000000000 ) ) ;
#38221=ADVANCED_FACE ( 'NONE', ( #3897 ), #47789, .T. ) ;
#38222=CARTESIAN_POINT ( 'NONE',  ( -332.3517673607765914, -135.0638248728647852, 57.91551518289418254 ) ) ;
#38224=EDGE_CURVE ( 'NONE', #33858, #28909, #14964, .T. ) ;
#38226=DIRECTION ( 'NONE',  ( 1.000000000000000000, 0.000000000000000000, 0.000000000000000000 ) ) ;
#38232=AXIS2_PLACEMENT_3D ( 'NONE', #18933, #14740, #30249 ) ;
#38233=DIRECTION ( 'NONE',  ( -0.000000000000000000, 0.000000000000000000, 1.000000000000000000 ) ) ;
#38241=VECTOR ( 'NONE', #29439, 1000.000000000000000 ) ;
#38243=ORIENTED_EDGE ( 'NONE', *, *, #38071, .F. ) ;
#38247=DIRECTION ( 'NONE',  ( 0.000000000000000000, 0.5680647467311485954, -0.8229838658936613482 ) ) ;
#38248=CIRCLE ( 'NONE', #29012, 60.00000000000000000 ) ;
#38249=DIRECTION ( 'NONE',  ( 0.000000000000000000, 0.9709418174260511236, -0.2393156642875615969 ) ) ;
#38255=VERTEX_POINT ( 'NONE', #47013 ) ;
#38259=DIRECTION ( 'NONE',  ( 1.000000000000000000, -0.000000000000000000, -0.000000000000000000 ) ) ;
#38260=VECTOR ( 'NONE', #27001, 1000.000000000000000 ) ;
#38264=ORIENTED_EDGE ( 'NONE', *, *, #13077, .F. ) ;
#38275=VECTOR ( 'NONE', #660, 1000.000000000000000 ) ;
#38280=LINE ( 'NONE', #34089, #7057 ) ;
#38283=VECTOR ( 'NONE', #11547, 1000.000000000000000 ) ;
#38284=AXIS2_PLACEMENT_3D ( 'NONE', #51392, #26934, #51919 ) ;
#38294=DIRECTION ( 'NONE',  ( 0.000000000000000000, -0.9927088740980553050, -0.1205366802553130001 ) ) ;
#38300=ORIENTED_EDGE ( 'NONE', *, *, #50605, .F. ) ;
#38303=DIRECTION ( 'NONE',  ( -0.000000000000000000, 1.047444401652940007E-14, 1.000000000000000000 ) ) ;
#38308=VERTEX_POINT ( 'NONE', #7063 ) ;
#38313=PLANE ( 'NONE',  #28855 ) ;
#38314=DIRECTION ( 'NONE',  ( 0.000000000000000000, -0.8229838658936494689, 0.5680647467311658039 ) ) ;
#38315=VERTEX_POINT ( 'NONE', #51734 ) ;
#38318=DIRECTION ( 'NONE',  ( 0.000000000000000000, 0.8854560256532093554, -0.4647231720437695057 ) ) ;
#38328=EDGE_CURVE ( 'NONE', #24446, #5479, #39867, .T. ) ;
#38329=VECTOR ( 'NONE', #32971, 1000.000000000000000 ) ;
#38332=CARTESIAN_POINT ( 'NONE',  ( -330.4913330509368166, -124.0000000000001990, -59.00000000000002132 ) ) ;
#38335=FACE_OUTER_BOUND ( 'NONE', #30177, .T. ) ;
#38337=VERTEX_POINT ( 'NONE', #14688 ) ;
#38339=EDGE_CURVE ( 'NONE', #19412, #30840, #15740, .T. ) ;
#38341=CARTESIAN_POINT ( 'NONE',  ( -332.3517673607765914, -86.34605966037949543, -45.90766452162698386 ) ) ;
#38344=ORIENTED_EDGE ( 'NONE', *, *, #31761, .T. ) ;
#38348=CARTESIAN_POINT ( 'NONE',  ( -332.3517673607765914, -136.0347666902908372, 57.67619951860663718 ) ) ;
#38351=CARTESIAN_POINT ( 'NONE',  ( -305.0000000000000568, -95.17484985463120495, 52.89315522108991985 ) ) ;
#38353=ORIENTED_EDGE ( 'NONE', *, *, #24088, .T. ) ;
#38355=EDGE_CURVE ( 'NONE', #5823, #37898, #46756, .T. ) ;
#38362=AXIS2_PLACEMENT_3D ( 'NONE', #33455, #8227, #25295 ) ;
#38364=FACE_OUTER_BOUND ( 'NONE', #32361, .T. ) ;
#38367=ORIENTED_EDGE ( 'NONE', *, *, #39404, .F. ) ;
#38368=VECTOR ( 'NONE', #25769, 1000.000000000000114 ) ;
#38370=EDGE_LOOP ( 'NONE', ( #2302, #29632, #43877, #22544 ) ) ;
#38371=FACE_OUTER_BOUND ( 'NONE', #31570, .T. ) ;
#38373=EDGE_LOOP ( 'NONE', ( #22863, #35823, #41588, #13045 ) ) ;
#38375=CARTESIAN_POINT ( 'NONE',  ( -332.3517673607765914, -180.1556192733800117, 16.67542351306693149 ) ) ;
#38378=LINE ( 'NONE', #18672, #49498 ) ;
#38383=CARTESIAN_POINT ( 'NONE',  ( -332.3517673607765914, -159.1821513111375452, -47.06073758877369073 ) ) ;
#38388=LINE ( 'NONE', #39156, #15589 ) ;
#38389=PLANE ( 'NONE',  #31149 ) ;
#38393=ORIENTED_EDGE ( 'NONE', *, *, #20745, .T. ) ;
#38396=CARTESIAN_POINT ( 'NONE',  ( -336.3521761649654422, -106.8245764869328980, 56.65561927337994064 ) ) ;
#38397=CARTESIAN_POINT ( 'NONE',  ( -339.1964088526558498, -182.0095552316576573, -7.608018572112655420 ) ) ;
#38401=EDGE_CURVE ( 'NONE', #48252, #22804, #31994, .T. ) ;
#38406=ORIENTED_EDGE ( 'NONE', *, *, #33392, .F. ) ;
#38407=EDGE_LOOP ( 'NONE', ( #27191, #37311, #15960, #43835 ) ) ;
#38413=EDGE_LOOP ( 'NONE', ( #39246, #8723, #37058, #4208 ) ) ;
#38414=EDGE_CURVE ( 'NONE', #2676, #8596, #12550, .T. ) ;
#38420=DIRECTION ( 'NONE',  ( -8.718379230999705894E-17, 0.6631226582407911962, -0.7485107481711046340 ) ) ;
#38423=ADVANCED_FACE ( 'NONE', ( #28045 ), #49074, .F. ) ;
#38437=VERTEX_POINT ( 'NONE', #5200 ) ;
#38439=LINE ( 'NONE', #30543, #50859 ) ;
#38441=FACE_BOUND ( 'NONE', #48092, .T. ) ;
#38446=ORIENTED_EDGE ( 'NONE', *, *, #35267, .F. ) ;
#38448=DIRECTION ( 'NONE',  ( -0.000000000000000000, -0.8229838658936596829, -0.5680647467311510379 ) ) ;
#38450=LINE ( 'NONE', #38953, #43313 ) ;
#38452=DIRECTION ( 'NONE',  ( 0.000000000000000000, 0.000000000000000000, -1.000000000000000000 ) ) ;
#38455=ORIENTED_EDGE ( 'NONE', *, *, #30458, .T. ) ;
#38459=LINE ( 'NONE', #18749, #1784 ) ;
#38460=PLANE ( 'NONE',  #22653 ) ;
#38461=LINE ( 'NONE', #46113, #22059 ) ;
#38462=ORIENTED_EDGE ( 'NONE', *, *, #10752, .T. ) ;
#38463=VECTOR ( 'NONE', #47859, 1000.000000000000000 ) ;
#38472=VERTEX_POINT ( 'NONE', #29089 ) ;
#38476=CARTESIAN_POINT ( 'NONE',  ( -339.1964088526558498, -71.02573290043838483, 26.97593913775504504 ) ) ;
#38477=CARTESIAN_POINT ( 'NONE',  ( -336.3521761649653854, -182.1255794688777314, -12.76876783163924323 ) ) ;
#38478=EDGE_CURVE ( 'NONE', #16432, #44450, #32783, .T. ) ;
#38479=ADVANCED_FACE ( 'NONE', ( #32252 ), #24905, .F. ) ;
#38481=DIRECTION ( 'NONE',  ( 0.000000000000000000, 0.000000000000000000, -1.000000000000000000 ) ) ;
#38482=VERTEX_POINT ( 'NONE', #44872 ) ;
#38487=DIRECTION ( 'NONE',  ( 0.000000000000000000, 0.000000000000000000, 1.000000000000000000 ) ) ;
#38488=PLANE ( 'NONE',  #5061 ) ;
#38489=EDGE_CURVE ( 'NONE', #23416, #46482, #15987, .T. ) ;
#38496=EDGE_CURVE ( 'NONE', #2507, #26071, #13062, .T. ) ;
#38497=ORIENTED_EDGE ( 'NONE', *, *, #22700, .F. ) ;
#38501=CARTESIAN_POINT ( 'NONE',  ( -330.4913330509368166, -79.00630452878473875, -38.74998146212148953 ) ) ;
#38505=PLANE ( 'NONE',  #32099 ) ;
#38507=EDGE_LOOP ( 'NONE', ( #21980, #12885, #16113, #30522 ) ) ;
#38509=ADVANCED_FACE ( 'NONE', ( #34339 ), #38009, .F. ) ;
#38510=ORIENTED_EDGE ( 'NONE', *, *, #47048, .F. ) ;
#38516=FACE_OUTER_BOUND ( 'NONE', #10669, .T. ) ;
#38521=EDGE_CURVE ( 'NONE', #20194, #24508, #45377, .T. ) ;
#38523=DIRECTION ( 'NONE',  ( 0.000000000000000000, -0.6631226582408016323, -0.7485107481710953081 ) ) ;
#38525=EDGE_CURVE ( 'NONE', #49884, #18723, #50128, .T. ) ;
#38530=VERTEX_POINT ( 'NONE', #30381 ) ;
#38539=VECTOR ( 'NONE', #22780, 1000.000000000000000 ) ;
#38540=CARTESIAN_POINT ( 'NONE',  ( -339.1964088526558498, -157.4273119900853146, -48.27201571435997352 ) ) ;
#38550=CARTESIAN_POINT ( 'NONE',  ( -332.3517673607765914, -75.06648993880729392, -35.41461708323759439 ) ) ;
#38551=ORIENTED_EDGE ( 'NONE', *, *, #24584, .F. ) ;
#38554=VECTOR ( 'NONE', #31903, 1000.000000000000000 ) ;
#38557=CARTESIAN_POINT ( 'NONE',  ( -330.4913330509368166, -84.75001853787810546, 44.49369547121489887 ) ) ;
#38561=ORIENTED_EDGE ( 'NONE', *, *, #42350, .T. ) ;
#38562=DIRECTION ( 'NONE',  ( 0.000000000000000000, -0.9350162426854146114, 0.3546048870425363986 ) ) ;
#38563=CARTESIAN_POINT ( 'NONE',  ( -336.3521761649654422, -64.50000000000000000, -2.632288850093980503 ) ) ;
#38565=EDGE_LOOP ( 'NONE', ( #33642, #16318, #28510, #4028 ) ) ;
#38567=EDGE_LOOP ( 'NONE', ( #46497, #8444, #261, #35375 ) ) ;
#38569=CARTESIAN_POINT ( 'NONE',  ( -305.0000000000000568, -63.67752800890095699, 4.612141029301498385 ) ) ;
#38578=FACE_OUTER_BOUND ( 'NONE', #17929, .T. ) ;
#38580=CARTESIAN_POINT ( 'NONE',  ( 0.000000000000000000, -102.5783116644897888, 55.16595831843925879 ) ) ;
#38581=LINE ( 'NONE', #33860, #22323 ) ;
#38582=CARTESIAN_POINT ( 'NONE',  ( -339.1964088526558498, -123.9999999999993747, 59.99791663049644086 ) ) ;
#38583=EDGE_LOOP ( 'NONE', ( #47563, #42190, #40589, #30924 ) ) ;
#38595=DIRECTION ( 'NONE',  ( -0.000000000000000000, -1.000000000000000000, -0.000000000000000000 ) ) ;
#38598=LINE ( 'NONE', #25998, #28143 ) ;
#38600=CARTESIAN_POINT ( 'NONE',  ( -365.0000000000001137, -78.50000000000002842, 0.000000000000000000 ) ) ;
#38601=AXIS2_PLACEMENT_3D ( 'NONE', #51279, #36015, #51799 ) ;
#38602=ORIENTED_EDGE ( 'NONE', *, *, #48348, .T. ) ;
#38614=LINE ( 'NONE', #10494, #20525 ) ;
#38619=ORIENTED_EDGE ( 'NONE', *, *, #43261, .F. ) ;
#38620=EDGE_LOOP ( 'NONE', ( #6880, #7197, #25573, #35521 ) ) ;
#38624=ORIENTED_EDGE ( 'NONE', *, *, #17702, .F. ) ;
#38628=FACE_OUTER_BOUND ( 'NONE', #21635, .T. ) ;
#38629=CARTESIAN_POINT ( 'NONE',  ( -336.3521761649654422, -65.24746378767824240, -9.724760635741734660 ) ) ;
#38641=PLANE ( 'NONE',  #25273 ) ;
#38643=CARTESIAN_POINT ( 'NONE',  ( -330.4913330509368166, -66.33409060400650503, 14.60509510167813474 ) ) ;
#38644=EDGE_CURVE ( 'NONE', #36738, #35874, #49856, .T. ) ;
#38646=ADVANCED_FACE ( 'NONE', ( #27482 ), #35618, .F. ) ;
#38648=DIRECTION ( 'NONE',  ( 0.000000000000000000, 1.385465816146810017E-13, 1.000000000000000000 ) ) ;
#38649=CARTESIAN_POINT ( 'NONE',  ( -330.4913330509368166, -95.17484985463094915, 52.89315522108979906 ) ) ;
#38656=ORIENTED_EDGE ( 'NONE', *, *, #28920, .T. ) ;
#38657=EDGE_LOOP ( 'NONE', ( #10429, #40912, #7998, #5571 ) ) ;
#38658=ORIENTED_EDGE ( 'NONE', *, *, #26972, .T. ) ;
#38670=EDGE_CURVE ( 'NONE', #22921, #19768, #34579, .T. ) ;
#38673=CARTESIAN_POINT ( 'NONE',  ( -330.4913330509368166, -176.8578783931336602, 27.43969411971572470 ) ) ;
#38674=ORIENTED_EDGE ( 'NONE', *, *, #843, .T. ) ;
#38675=CARTESIAN_POINT ( 'NONE',  ( -336.3521761649654422, -64.61288906875131488, 4.498567634385603142 ) ) ;
#38676=DIRECTION ( 'NONE',  ( 0.000000000000000000, 0.000000000000000000, 1.000000000000000000 ) ) ;
#38677=PLANE ( 'NONE',  #45887 ) ;
#38686=EDGE_CURVE ( 'NONE', #14634, #23542, #15671, .T. ) ;
#38688=FACE_BOUND ( 'NONE', #50465, .T. ) ;
#38690=AXIS2_PLACEMENT_3D ( 'NONE', #51991, #41168, #12270 ) ;
#38692=ORIENTED_EDGE ( 'NONE', *, *, #18836, .T. ) ;
#38694=ORIENTED_EDGE ( 'NONE', *, *, #25022, .F. ) ;
#38696=DIRECTION ( 'NONE',  ( 0.000000000000000000, 0.000000000000000000, 1.000000000000000000 ) ) ;
#38699=CARTESIAN_POINT ( 'NONE',  ( -305.0000000000000568, -168.7406467949202806, 39.41172259083927543 ) ) ;
#38700=DIRECTION ( 'NONE',  ( -1.000000000000000000, -0.000000000000000000, -0.000000000000000000 ) ) ;
#38701=EDGE_CURVE ( 'NONE', #38482, #30451, #19597, .T. ) ;
#38702=EDGE_CURVE ( 'NONE', #15571, #45713, #19094, .T. ) ;
#38711=VERTEX_POINT ( 'NONE', #26959 ) ;
#38712=EDGE_LOOP ( 'NONE', ( #50195, #51116, #26698, #41913 ) ) ;
#38713=CARTESIAN_POINT ( 'NONE',  ( -336.3521761649654422, -68.91285928486892942, -22.44790492310182017 ) ) ;
#38716=DIRECTION ( 'NONE',  ( -1.000000000000000000, -0.000000000000000000, 0.000000000000000000 ) ) ;
#38718=DIRECTION ( 'NONE',  ( -0.000000000000000000, 0.8854560256532157947, 0.4647231720437573488 ) ) ;
#38721=DIRECTION ( 'NONE',  ( -0.000000000000000000, -0.9927088740980530845, 0.1205366802553303057 ) ) ;
#38731=ORIENTED_EDGE ( 'NONE', *, *, #38644, .F. ) ;
#38733=AXIS2_PLACEMENT_3D ( 'NONE', #17848, #41225, #17082 ) ;
#38736=PLANE ( 'NONE',  #22307 ) ;
#38740=PLANE ( 'NONE',  #3182 ) ;
#38743=ADVANCED_FACE ( 'NONE', ( #10682 ), #7522, .F. ) ;
#38747=LINE ( 'NONE', #27178, #25082 ) ;
#38751=ORIENTED_EDGE ( 'NONE', *, *, #26166, .F. ) ;
#38752=EDGE_CURVE ( 'NONE', #17498, #33612, #31419, .T. ) ;
#38754=PLANE ( 'NONE',  #29009 ) ;
#38762=VERTEX_POINT ( 'NONE', #23022 ) ;
#38766=EDGE_LOOP ( 'NONE', ( #47842, #27433, #17507, #6501 ) ) ;
#38770=EDGE_LOOP ( 'NONE', ( #20386, #42885, #11913, #6795 ) ) ;
#38775=VERTEX_POINT ( 'NONE', #36140 ) ;
#38779=LINE ( 'NONE', #2784, #19904 ) ;
#38784=ORIENTED_EDGE ( 'NONE', *, *, #23099, .F. ) ;
#38794=CARTESIAN_POINT ( 'NONE',  ( -339.1964088526558498, -123.5000000000000284, -60.00000000000000000 ) ) ;
#38800=CARTESIAN_POINT ( 'NONE',  ( -332.3517673607765914, -159.7173995167596274, -47.83617848703448772 ) ) ;
#38803=EDGE_CURVE ( 'NONE', #50020, #42079, #4345, .T. ) ;
#38805=EDGE_CURVE ( 'NONE', #42455, #31317, #12996, .T. ) ;
#38809=DIRECTION ( 'NONE',  ( 0.000000000000000000, 0.3546048870425331234, -0.9350162426854158326 ) ) ;
#38811=VECTOR ( 'NONE', #19560, 1000.000000000000000 ) ;
#38812=EDGE_CURVE ( 'NONE', #42898, #3693, #12488, .T. ) ;
#38813=ORIENTED_EDGE ( 'NONE', *, *, #39112, .T. ) ;
#38816=CARTESIAN_POINT ( 'NONE',  ( -339.1964088526558498, -109.8658467157464571, 57.40522506028071348 ) ) ;
#38818=EDGE_CURVE ( 'NONE', #23565, #50532, #136, .T. ) ;
#38821=EDGE_LOOP ( 'NONE', ( #35583, #11400, #46720, #20106 ) ) ;
#38823=DIRECTION ( 'NONE',  ( -8.718379230999705894E-17, 0.9350162426854132791, -0.3546048870425396182 ) ) ;
#38828=VERTEX_POINT ( 'NONE', #15931 ) ;
#38834=EDGE_CURVE ( 'NONE', #35535, #15154, #24835, .T. ) ;
#38835=LINE ( 'NONE', #39599, #4595 ) ;
#38836=VECTOR ( 'NONE', #28019, 1000.000000000000114 ) ;
#38837=CARTESIAN_POINT ( 'NONE',  ( -332.3517673607765914, -123.5000000000000284, 0.000000000000000000 ) ) ;
#38838=EDGE_CURVE ( 'NONE', #16966, #17396, #42055, .T. ) ;
#38839=VERTEX_POINT ( 'NONE', #32198 ) ;
#38842=ADVANCED_FACE ( 'NONE', ( #40084 ), #4882, .T. ) ;
#38844=CARTESIAN_POINT ( 'NONE',  ( -330.4913330509368166, -123.5000000000000284, 0.000000000000000000 ) ) ;
#38847=DIRECTION ( 'NONE',  ( -0.000000000000000000, -0.8229838658936516893, 0.5680647467311626952 ) ) ;
#38849=VECTOR ( 'NONE', #29866, 1000.000000000000227 ) ;
#38850=ADVANCED_FACE ( 'NONE', ( #917 ), #44551, .F. ) ;
#38856=VERTEX_POINT ( 'NONE', #7770 ) ;
#38857=DIRECTION ( 'NONE',  ( -1.000000000000000000, -0.000000000000000000, 0.000000000000000000 ) ) ;
#38859=PLANE ( 'NONE',  #14176 ) ;
#38861=EDGE_LOOP ( 'NONE', ( #30205, #977, #23175, #16927 ) ) ;
#38863=FILL_AREA_STYLE_COLOUR ( '', #39841 ) ;
#38870=EDGE_CURVE ( 'NONE', #3626, #809, #45090, .T. ) ;
#38872=LINE ( 'NONE', #47035, #32589 ) ;
#38873=VERTEX_POINT ( 'NONE', #21153 ) ;
#38875=LINE ( 'NONE', #27303, #2347 ) ;
#38880=CARTESIAN_POINT ( 'NONE',  ( -336.3521761649654422, -154.8494888031386836, 50.05135858667791382 ) ) ;
#38886=CARTESIAN_POINT ( 'NONE',  ( 0.000000000000000000, -175.7419055135395922, -27.41866715058203852 ) ) ;
#38889=ORIENTED_EDGE ( 'NONE', *, *, #30815, .F. ) ;
#38894=EDGE_LOOP ( 'NONE', ( #17793, #29365, #38455, #816 ) ) ;
#38899=CARTESIAN_POINT ( 'NONE',  ( -336.3521761649653854, -77.52356969168074841, 38.55084767037245541 ) ) ;
#38900=LINE ( 'NONE', #3171, #28288 ) ;
#38902=ADVANCED_FACE ( 'NONE', ( #45348 ), #1170, .F. ) ;
#38905=DIRECTION ( 'NONE',  ( 1.000000000000000000, -5.781354811211920680E-17, -6.525800561034928863E-17 ) ) ;
#38907=DIRECTION ( 'NONE',  ( 0.000000000000000000, 0.5680647467311569221, 0.8229838658936556861 ) ) ;
#38915=ORIENTED_EDGE ( 'NONE', *, *, #15429, .F. ) ;
#38916=FACE_OUTER_BOUND ( 'NONE', #41485, .T. ) ;
#38918=CIRCLE ( 'NONE', #37244, 60.00000000000000000 ) ;
#38924=VERTEX_POINT ( 'NONE', #13276 ) ;
#38928=EDGE_LOOP ( 'NONE', ( #3711, #34599, #14111, #49396 ) ) ;
#38931=DIRECTION ( 'NONE',  ( 0.000000000000000000, 0.000000000000000000, -1.000000000000000000 ) ) ;
#38936=CARTESIAN_POINT ( 'NONE',  ( -336.3521761649654422, -127.9985676343858501, 58.88711093124869222 ) ) ;
#38937=EDGE_LOOP ( 'NONE', ( #25287, #22240, #30465, #32852 ) ) ;
#38941=VECTOR ( 'NONE', #12582, 1000.000000000000000 ) ;
#38943=FACE_BOUND ( 'NONE', #7491, .T. ) ;
#38953=CARTESIAN_POINT ( 'NONE',  ( -339.1964088526558498, -79.00630452878473875, -38.74998146212148953 ) ) ;
#38954=PLANE ( 'NONE',  #9627 ) ;
#38957=ORIENTED_EDGE ( 'NONE', *, *, #19130, .F. ) ;
#38961=CARTESIAN_POINT ( 'NONE',  ( -332.3517673607765914, -170.1129345408509153, -37.77875505479703122 ) ) ;
#38962=CARTESIAN_POINT ( 'NONE',  ( -332.3517673607765914, -118.0087234915157381, -58.76657425099333665 ) ) ;
#38963=ORIENTED_EDGE ( 'NONE', *, *, #45998, .F. ) ;
#38969=VERTEX_POINT ( 'NONE', #14061 ) ;
#38970=PLANE ( 'NONE',  #20576 ) ;
#38974=VECTOR ( 'NONE', #18460, 1000.000000000000000 ) ;
#38975=VECTOR ( 'NONE', #23630, 1000.000000000000000 ) ;
#38976=CARTESIAN_POINT ( 'NONE',  ( -336.3521761649654422, -182.2665742509934148, -5.491276508484069119 ) ) ;
#38979=ORIENTED_EDGE ( 'NONE', *, *, #47029, .T. ) ;
#38980=VECTOR ( 'NONE', #41349, 1000.000000000000114 ) ;
#38982=ADVANCED_FACE ( 'NONE', ( #9335 ), #25874, .F. ) ;
#38985=LINE ( 'NONE', #43716, #42523 ) ;
#38991=CARTESIAN_POINT ( 'NONE',  ( -339.1964088526558498, -130.2355952558269507, -59.62073260661665586 ) ) ;
#38997=DIRECTION ( 'NONE',  ( 0.000000000000000000, 0.000000000000000000, 1.000000000000000000 ) ) ;
#38999=LINE ( 'NONE', #35576, #5712 ) ;
#39001=DIRECTION ( 'NONE',  ( -0.000000000000000000, -0.8229838658936596829, -0.5680647467311510379 ) ) ;
#39007=CARTESIAN_POINT ( 'NONE',  ( -305.0000000000000568, -70.60684477890980304, -28.32515014536826214 ) ) ;
#39008=EDGE_CURVE ( 'NONE', #33330, #41587, #10105, .T. ) ;
#39009=ORIENTED_EDGE ( 'NONE', *, *, #23974, .F. ) ;
#39010=CIRCLE ( 'NONE', #30644, 60.00000000000000000 ) ;
#39014=PLANE ( 'NONE',  #42454 ) ;
#39015=DIRECTION ( 'NONE',  ( 0.000000000000000000, 0.000000000000000000, 1.000000000000000000 ) ) ;
#39018=EDGE_LOOP ( 'NONE', ( #8349, #35129, #12609, #24525 ) ) ;
#39019=VECTOR ( 'NONE', #30464, 1000.000000000000114 ) ;
#39023=VECTOR ( 'NONE', #4338, 1000.000000000000000 ) ;
#39024=ORIENTED_EDGE ( 'NONE', *, *, #29275, .T. ) ;
#39026=VECTOR ( 'NONE', #43903, 1000.000000000000000 ) ;
#39028=VECTOR ( 'NONE', #28581, 1000.000000000000000 ) ;
#39034=CARTESIAN_POINT ( 'NONE',  ( -330.4913330509368166, -181.6348283828473029, -14.84391218300937609 ) ) ;
#39041=ORIENTED_EDGE ( 'NONE', *, *, #40962, .F. ) ;
#39043=LINE ( 'NONE', #5975, #10053 ) ;
#39044=VECTOR ( 'NONE', #12387, 1000.000000000000000 ) ;
#39047=LINE ( 'NONE', #15424, #12741 ) ;
#39050=VECTOR ( 'NONE', #32632, 1000.000000000000000 ) ;
#39051=ADVANCED_FACE ( 'NONE', ( #27151 ), #26385, .F. ) ;
#39056=VERTEX_POINT ( 'NONE', #34522 ) ;
#39057=VERTEX_POINT ( 'NONE', #31358 ) ;
#39061=CARTESIAN_POINT ( 'NONE',  ( -330.4913330509368166, -162.9984922102926532, -43.83057281297441676 ) ) ;
#39066=VERTEX_POINT ( 'NONE', #38976 ) ;
#39068=AXIS2_PLACEMENT_3D ( 'NONE', #19247, #35256, #43666 ) ;
#39071=ORIENTED_EDGE ( 'NONE', *, *, #32729, .T. ) ;
#39077=FACE_OUTER_BOUND ( 'NONE', #24194, .T. ) ;
#39089=EDGE_LOOP ( 'NONE', ( #38602, #4929, #33571, #10488 ) ) ;
#39095=AXIS2_PLACEMENT_3D ( 'NONE', #37452, #1717, #49821 ) ;
#39102=DIRECTION ( 'NONE',  ( 1.000000000000000000, 8.654812430365579069E-17, 1.050884489711633576E-17 ) ) ;
#39106=VECTOR ( 'NONE', #19548, 1000.000000000000000 ) ;
#39108=ORIENTED_EDGE ( 'NONE', *, *, #2155, .T. ) ;
#39110=CARTESIAN_POINT ( 'NONE',  ( -365.0000000000001137, -168.5000000000000284, -10.00000000000000711 ) ) ;
#39111=EDGE_CURVE ( 'NONE', #10774, #12239, #15099, .T. ) ;
#39112=EDGE_CURVE ( 'NONE', #3787, #42007, #42090, .T. ) ;
#39113=FACE_OUTER_BOUND ( 'NONE', #36628, .T. ) ;
#39117=DIRECTION ( 'NONE',  ( 1.000000000000000000, 8.151826190875887961E-17, -3.091579882402674147E-17 ) ) ;
#39124=DIRECTION ( 'NONE',  ( -0.000000000000000000, -0.5680647467311485954, 0.8229838658936613482 ) ) ;
#39125=ORIENTED_EDGE ( 'NONE', *, *, #40046, .T. ) ;
#39126=AXIS2_PLACEMENT_3D ( 'NONE', #49460, #46034, #42061 ) ;
#39131=DIRECTION ( 'NONE',  ( -0.000000000000000000, 0.3546048870425463906, 0.9350162426854107256 ) ) ;
#39134=DIRECTION ( 'NONE',  ( 1.000000000000000000, -0.000000000000000000, 0.000000000000000000 ) ) ;
#39140=AXIS2_PLACEMENT_3D ( 'NONE', #3717, #40489, #32624 ) ;
#39143=CARTESIAN_POINT ( 'NONE',  ( -336.3521761649654422, -182.5000000000000568, 2.632288850093980503 ) ) ;
#39146=DIRECTION ( 'NONE',  ( 1.000000000000000000, -8.151826190875929870E-17, -3.091579882402562597E-17 ) ) ;
#39152=DIRECTION ( 'NONE',  ( 0.000000000000000000, 0.000000000000000000, 1.000000000000000000 ) ) ;
#39153=AXIS2_PLACEMENT_3D ( 'NONE', #29758, #21365, #37389 ) ;
#39156=CARTESIAN_POINT ( 'NONE',  ( -336.3521761649654422, -64.50000000000000000, -1.632288850093980725 ) ) ;
#39166=AXIS2_PLACEMENT_3D ( 'NONE', #33736, #41610, #30053 ) ;
#39183=CARTESIAN_POINT ( 'NONE',  ( -339.1964088526558498, -144.3080463282022663, -56.27632902032068785 ) ) ;
#39187=EDGE_LOOP ( 'NONE', ( #7729, #29688, #44010, #5777 ) ) ;
#39189=CARTESIAN_POINT ( 'NONE',  ( -339.1964088526558498, -103.0458197858324496, 55.34326076196052213 ) ) ;
#39190=DIRECTION ( 'NONE',  ( 0.000000000000000000, -0.6631226582407937498, 0.7485107481711024136 ) ) ;
#39194=ADVANCED_FACE ( 'NONE', ( #48176 ), #40522, .T. ) ;
#39198=ORIENTED_EDGE ( 'NONE', *, *, #46223, .F. ) ;
#39200=DIRECTION ( 'NONE',  ( -0.000000000000000000, 0.5680647467311540355, -0.8229838658936575735 ) ) ;
#39201=CARTESIAN_POINT ( 'NONE',  ( -332.3517673607765914, -67.75522407825191351, 19.39547174791671935 ) ) ;
#39206=VECTOR ( 'NONE', #45110, 1000.000000000000000 ) ;
#39210=CARTESIAN_POINT ( 'NONE',  ( -332.3517673607765914, -179.5993808087905279, -18.46045550523168899 ) ) ;
#39212=CARTESIAN_POINT ( 'NONE',  ( -330.4913330509368166, -68.51134412508180560, -21.38919645685231075 ) ) ;
#39214=DIRECTION ( 'NONE',  ( -1.000000000000000000, 1.013386094502325718E-14, 2.497772389992443424E-15 ) ) ;
#39216=FACE_BOUND ( 'NONE', #41952, .T. ) ;
#39217=CARTESIAN_POINT ( 'NONE',  ( 0.000000000000000000, -123.5000000000002416, -59.00000000000002132 ) ) ;
#39226=AXIS2_PLACEMENT_3D ( 'NONE', #1722, #29571, #41654 ) ;
#39235=CARTESIAN_POINT ( 'NONE',  ( -332.3517673607765914, -75.87119766449505676, -34.85916744524372746 ) ) ;
#39237=ORIENTED_EDGE ( 'NONE', *, *, #3538, .T. ) ;
#39238=ORIENTED_EDGE ( 'NONE', *, *, #49912, .T. ) ;
#39241=DIRECTION ( 'NONE',  ( 0.000000000000000000, 0.000000000000000000, -1.000000000000000000 ) ) ;
#39246=ORIENTED_EDGE ( 'NONE', *, *, #2860, .T. ) ;
#39249=DIRECTION ( 'NONE',  ( 1.000000000000000000, 0.000000000000000000, 8.718379230999707126E-17 ) ) ;
#39251=AXIS2_PLACEMENT_3D ( 'NONE', #17995, #22188, #32968 ) ;
#39256=ORIENTED_EDGE ( 'NONE', *, *, #2010, .F. ) ;
#39260=DIRECTION ( 'NONE',  ( -1.000000000000000000, 0.000000000000000000, 0.000000000000000000 ) ) ;
#39269=VECTOR ( 'NONE', #42818, 1000.000000000000000 ) ;
#39273=DIRECTION ( 'NONE',  ( 1.000000000000000000, 0.000000000000000000, 0.000000000000000000 ) ) ;
#39276=FACE_OUTER_BOUND ( 'NONE', #47982, .T. ) ;
#39277=LINE ( 'NONE', #26923, #9198 ) ;
#39278=ORIENTED_EDGE ( 'NONE', *, *, #20184, .F. ) ;
#39280=ADVANCED_FACE ( 'NONE', ( #40262 ), #4278, .F. ) ;
#39295=ORIENTED_EDGE ( 'NONE', *, *, #11621, .F. ) ;
#39299=VERTEX_POINT ( 'NONE', #24502 ) ;
#39304=FACE_OUTER_BOUND ( 'NONE', #31921, .T. ) ;
#39308=DIRECTION ( 'NONE',  ( -1.000000000000000000, -0.000000000000000000, 0.000000000000000000 ) ) ;
#39317=EDGE_CURVE ( 'NONE', #6162, #16187, #15832, .T. ) ;
#39321=EDGE_CURVE ( 'NONE', #16323, #15864, #11652, .T. ) ;
#39322=CARTESIAN_POINT ( 'NONE',  ( -339.1964088526558498, -84.08827740916129301, -45.24064679492073537 ) ) ;
#39327=VERTEX_POINT ( 'NONE', #29741 ) ;
#39330=CIRCLE ( 'NONE', #16700, 60.00000000000000000 ) ;
#39331=ORIENTED_EDGE ( 'NONE', *, *, #29013, .T. ) ;
#39334=DIRECTION ( 'NONE',  ( 1.000000000000000000, 8.465038975556392596E-17, -2.086444717177575158E-17 ) ) ;
#39336=PLANE ( 'NONE',  #7410 ) ;
#39337=EDGE_LOOP ( 'NONE', ( #31578, #29181, #51436, #13644 ) ) ;
#39339=VERTEX_POINT ( 'NONE', #33941 ) ;
#39344=EDGE_CURVE ( 'NONE', #41229, #12335, #25546, .T. ) ;
#39347=ORIENTED_EDGE ( 'NONE', *, *, #34971, .F. ) ;
#39350=CARTESIAN_POINT ( 'NONE',  ( 0.000000000000000000, -71.25809448646026567, 27.41866715058169390 ) ) ;
#39354=AXIS2_PLACEMENT_3D ( 'NONE', #19657, #20178, #200 ) ;
#39365=CARTESIAN_POINT ( 'NONE',  ( -330.4913330509368166, -115.8919814278871598, -58.50955523165758621 ) ) ;
#39368=ORIENTED_EDGE ( 'NONE', *, *, #41365, .F. ) ;
#39372=CARTESIAN_POINT ( 'NONE',  ( -330.4913330509368166, -89.57268800991444380, 48.27201571435978877 ) ) ;
#39375=PLANE ( 'NONE',  #1495 ) ;
#39377=ORIENTED_EDGE ( 'NONE', *, *, #35617, .F. ) ;
#39383=ORIENTED_EDGE ( 'NONE', *, *, #12163, .F. ) ;
#39384=LINE ( 'NONE', #51492, #43510 ) ;
#39385=ORIENTED_EDGE ( 'NONE', *, *, #38702, .T. ) ;
#39387=LINE ( 'NONE', #27042, #20797 ) ;
#39388=ORIENTED_EDGE ( 'NONE', *, *, #45396, .T. ) ;
#39389=DIRECTION ( 'NONE',  ( 1.000000000000000000, -0.000000000000000000, -0.000000000000000000 ) ) ;
#39390=ORIENTED_EDGE ( 'NONE', *, *, #3447, .F. ) ;
#39393=PLANE ( 'NONE',  #7072 ) ;
#39396=DIRECTION ( 'NONE',  ( 0.000000000000000000, -0.1205366802553130001, 0.9927088740980551940 ) ) ;
#39402=PLANE ( 'NONE',  #14549 ) ;
#39404=EDGE_CURVE ( 'NONE', #41896, #4643, #33695, .T. ) ;
#39405=FACE_OUTER_BOUND ( 'NONE', #37578, .T. ) ;
#39406=ORIENTED_EDGE ( 'NONE', *, *, #31455, .T. ) ;
#39408=EDGE_CURVE ( 'NONE', #13737, #153, #5157, .T. ) ;
#39409=LINE ( 'NONE', #47321, #50454 ) ;
#39419=EDGE_CURVE ( 'NONE', #48198, #16597, #45022, .T. ) ;
#39425=EDGE_LOOP ( 'NONE', ( #44646, #2162, #37533, #38099 ) ) ;
#39432=ORIENTED_EDGE ( 'NONE', *, *, #16978, .F. ) ;
#39437=DIRECTION ( 'NONE',  ( -1.000000000000000000, -0.000000000000000000, 0.000000000000000000 ) ) ;
#39438=LINE ( 'NONE', #21297, #29174 ) ;
#39439=LINE ( 'NONE', #51291, #11530 ) ;
#39442=ORIENTED_EDGE ( 'NONE', *, *, #40046, .F. ) ;
#39443=LINE ( 'NONE', #16317, #41494 ) ;
#39445=CARTESIAN_POINT ( 'NONE',  ( -330.4913330509368166, -103.0458197858332312, -55.34326076196081345 ) ) ;
#39446=CARTESIAN_POINT ( 'NONE',  ( -336.3521761649653854, -82.50558083279611310, 43.81161486573607533 ) ) ;
#39450=EDGE_CURVE ( 'NONE', #33330, #24129, #18962, .T. ) ;
#39467=DIRECTION ( 'NONE',  ( 0.000000000000000000, 1.595945597898662527E-14, 1.000000000000000000 ) ) ;
#39470=EDGE_CURVE ( 'NONE', #20555, #3885, #6629, .T. ) ;
#39473=CARTESIAN_POINT ( 'NONE',  ( -339.1964088526558498, -157.4273119900853146, -48.27201571435997352 ) ) ;
#39477=ADVANCED_FACE ( 'NONE', ( #30269 ), #11313, .F. ) ;
#39486=ORIENTED_EDGE ( 'NONE', *, *, #3047, .F. ) ;
#39487=PLANE ( 'NONE',  #13191 ) ;
#39490=ORIENTED_EDGE ( 'NONE', *, *, #50713, .F. ) ;
#39492=AXIS2_PLACEMENT_3D ( 'NONE', #18261, #34281, #21933 ) ;
#39493=DIRECTION ( 'NONE',  ( -0.000000000000000000, -0.5680647467311485954, 0.8229838658936613482 ) ) ;
#39494=ORIENTED_EDGE ( 'NONE', *, *, #38328, .T. ) ;
#39496=LINE ( 'NONE', #19782, #31712 ) ;
#39498=CARTESIAN_POINT ( 'NONE',  ( -339.1964088526558498, -89.00580675195261904, 49.09328500076523483 ) ) ;
#39507=FACE_OUTER_BOUND ( 'NONE', #28585, .T. ) ;
#39514=EDGE_LOOP ( 'NONE', ( #17934, #39009, #49579, #21751 ) ) ;
#39518=VERTEX_POINT ( 'NONE', #34466 ) ;
#39522=LINE ( 'NONE', #46928, #5000 ) ;
#39525=CARTESIAN_POINT ( 'NONE',  ( -332.3517673607765914, -105.0395444947681369, -56.09938080879045685 ) ) ;
#39527=DIRECTION ( 'NONE',  ( -1.000000000000000000, -0.000000000000000000, -0.000000000000000000 ) ) ;
#39533=DIRECTION ( 'NONE',  ( -8.718379230999707126E-17, -0.9927088740980527515, 0.1205366802553337890 ) ) ;
#39535=LINE ( 'NONE', #3545, #43753 ) ;
#39540=CARTESIAN_POINT ( 'NONE',  ( -330.4913330509368166, -84.00150778970706256, 43.83057281297416097 ) ) ;
#39545=EDGE_CURVE ( 'NONE', #49872, #20460, #39562, .T. ) ;
#39546=AXIS2_PLACEMENT_3D ( 'NONE', #44600, #8589, #24619 ) ;
#39550=CARTESIAN_POINT ( 'NONE',  ( -330.4913330509368166, -175.9742670995611036, 26.97593913775620678 ) ) ;
#39551=ORIENTED_EDGE ( 'NONE', *, *, #4263, .T. ) ;
#39553=CARTESIAN_POINT ( 'NONE',  ( -365.0000000000001137, -168.5000000000000284, -5.000000000000001776 ) ) ;
#39556=ORIENTED_EDGE ( 'NONE', *, *, #2760, .F. ) ;
#39562=CIRCLE ( 'NONE', #32027, 60.00000000000000000 ) ;
#39568=VERTEX_POINT ( 'NONE', #7403 ) ;
#39576=EDGE_CURVE ( 'NONE', #34925, #32740, #24641, .T. ) ;
#39578=EDGE_LOOP ( 'NONE', ( #18501, #12284, #37942, #24040 ) ) ;
#39579=CARTESIAN_POINT ( 'NONE',  ( -339.1964088526558498, -175.5095439275177398, -27.86139516340860212 ) ) ;
#39580=AXIS2_PLACEMENT_3D ( 'NONE', #45122, #20665, #9112 ) ;
#39585=CARTESIAN_POINT ( 'NONE',  ( -339.1964088526558498, -123.5000000000000284, 0.000000000000000000 ) ) ;
#39586=DIRECTION ( 'NONE',  ( -1.000000000000000000, -0.000000000000000000, -0.000000000000000000 ) ) ;
#39592=FACE_OUTER_BOUND ( 'NONE', #15203, .T. ) ;
#39597=VECTOR ( 'NONE', #24001, 1000.000000000000000 ) ;
#39599=CARTESIAN_POINT ( 'NONE',  ( -339.1964088526558498, -79.00630452878414189, 38.74998146212082162 ) ) ;
#39606=CARTESIAN_POINT ( 'NONE',  ( -336.3521761649654422, -133.2247606357419443, -58.25253621232173629 ) ) ;
#39610=ORIENTED_EDGE ( 'NONE', *, *, #13065, .T. ) ;
#39613=CARTESIAN_POINT ( 'NONE',  ( -336.3521761649654422, -140.1754235130667610, -56.65561927338005432 ) ) ;
#39619=VECTOR ( 'NONE', #48980, 1000.000000000000000 ) ;
#39623=CARTESIAN_POINT ( 'NONE',  ( -336.3521761649654422, -64.50000000000000000, -2.632288850093980503 ) ) ;
#39627=ORIENTED_EDGE ( 'NONE', *, *, #31710, .F. ) ;
#39628=DIRECTION ( 'NONE',  ( -0.000000000000000000, 0.7485107481710934207, -0.6631226582408039638 ) ) ;
#39632=EDGE_CURVE ( 'NONE', #29000, #14596, #33315, .T. ) ;
#39633=CARTESIAN_POINT ( 'NONE',  ( -339.1964088526558498, -115.8919814278862503, 58.50955523165745831 ) ) ;
#39645=CARTESIAN_POINT ( 'NONE',  ( -330.4913330509368166, -151.8251501453686956, -52.89315522109000511 ) ) ;
#39647=VECTOR ( 'NONE', #29580, 1000.000000000000000 ) ;
#39650=CARTESIAN_POINT ( 'NONE',  ( -336.3521761649654422, -182.2665742509934148, -5.491276508484069119 ) ) ;
#39651=DIRECTION ( 'NONE',  ( 0.000000000000000000, 0.000000000000000000, -1.000000000000000000 ) ) ;
#39654=ORIENTED_EDGE ( 'NONE', *, *, #402, .T. ) ;
#39656=ADVANCED_FACE ( 'NONE', ( #17039 ), #20438, .F. ) ;
#39662=EDGE_LOOP ( 'NONE', ( #17145, #47481, #43763, #37234 ) ) ;
#39666=VECTOR ( 'NONE', #45368, 1000.000000000000000 ) ;
#39667=LINE ( 'NONE', #35739, #21143 ) ;
#39672=ORIENTED_EDGE ( 'NONE', *, *, #46870, .T. ) ;
#39674=VERTEX_POINT ( 'NONE', #8606 ) ;
#39676=CIRCLE ( 'NONE', #18742, 60.00000000000000000 ) ;
#39678=EDGE_CURVE ( 'NONE', #34018, #3155, #44618, .T. ) ;
#39680=VECTOR ( 'NONE', #22959, 1000.000000000000000 ) ;
#39681=CARTESIAN_POINT ( 'NONE',  ( -336.3521761649654422, -163.8460225846223466, -43.07972642080364523 ) ) ;
#39684=LINE ( 'NONE', #6637, #37543 ) ;
#39686=CARTESIAN_POINT ( 'NONE',  ( -330.4913330509368166, -157.4273119900852578, -48.27201571436002325 ) ) ;
#39688=FACE_OUTER_BOUND ( 'NONE', #21080, .T. ) ;
#39689=EDGE_LOOP ( 'NONE', ( #37841, #10516, #20216, #29706 ) ) ;
#39690=FACE_OUTER_BOUND ( 'NONE', #372, .T. ) ;
#39691=EDGE_CURVE ( 'NONE', #18519, #11626, #458, .T. ) ;
#39693=DIRECTION ( 'NONE',  ( -0.000000000000000000, 0.8229838658936634577, 0.5680647467311457088 ) ) ;
#39695=VECTOR ( 'NONE', #49466, 1000.000000000000000 ) ;
#39697=ADVANCED_FACE ( 'NONE', ( #31551 ), #47607, .F. ) ;
#39698=FACE_OUTER_BOUND ( 'NONE', #41346, .T. ) ;
#39704=DIRECTION ( 'NONE',  ( -1.000000000000000000, 0.000000000000000000, -0.000000000000000000 ) ) ;
#39707=ORIENTED_EDGE ( 'NONE', *, *, #34076, .F. ) ;
#39711=ORIENTED_EDGE ( 'NONE', *, *, #28073, .F. ) ;
#39712=DIRECTION ( 'NONE',  ( 0.000000000000000000, 0.000000000000000000, -1.000000000000000000 ) ) ;
#39713=EDGE_LOOP ( 'NONE', ( #32553, #28096, #10363, #29440 ) ) ;
#39715=CARTESIAN_POINT ( 'NONE',  ( -330.4913330509368166, -71.02573290043878274, -26.97593913775585150 ) ) ;
#39719=DIRECTION ( 'NONE',  ( -0.000000000000000000, -0.9709418174260502354, 0.2393156642875652051 ) ) ;
#39720=AXIS2_PLACEMENT_3D ( 'NONE', #45973, #25975, #22030 ) ;
#39725=EDGE_LOOP ( 'NONE', ( #1928, #36256, #30037, #919 ) ) ;
#39726=ORIENTED_EDGE ( 'NONE', *, *, #13522, .F. ) ;
#39729=EDGE_CURVE ( 'NONE', #5479, #42477, #17561, .T. ) ;
#39736=FACE_OUTER_BOUND ( 'NONE', #16699, .T. ) ;
#39737=EDGE_CURVE ( 'NONE', #2241, #33953, #49609, .T. ) ;
#39741=DIRECTION ( 'NONE',  ( -1.000000000000000000, 0.000000000000000000, 0.000000000000000000 ) ) ;
#39742=VERTEX_POINT ( 'NONE', #37767 ) ;
#39743=EDGE_LOOP ( 'NONE', ( #51533, #29256, #46803, #28329 ) ) ;
#39747=DIRECTION ( 'NONE',  ( -0.000000000000000000, 0.9350162426854158326, 0.3546048870425331789 ) ) ;
#39748=CARTESIAN_POINT ( 'NONE',  ( -336.3521761649654422, -123.5000000000000284, 0.000000000000000000 ) ) ;
#39749=EDGE_CURVE ( 'NONE', #11792, #6023, #47986, .T. ) ;
#39751=CARTESIAN_POINT ( 'NONE',  ( -330.4913330509368166, -75.22798428563987727, -33.92731199008506593 ) ) ;
#39752=CIRCLE ( 'NONE', #5357, 60.00000000000000000 ) ;
#39754=LINE ( 'NONE', #340, #2856 ) ;
#39755=EDGE_CURVE ( 'NONE', #15605, #24889, #26139, .T. ) ;
#39758=VECTOR ( 'NONE', #5435, 1000.000000000000000 ) ;
#39760=ORIENTED_EDGE ( 'NONE', *, *, #13800, .F. ) ;
#39762=ORIENTED_EDGE ( 'NONE', *, *, #42745, .T. ) ;
#39765=CARTESIAN_POINT ( 'NONE',  ( -339.1964088526558498, -66.33409060400673241, -14.60509510167901404 ) ) ;
#39767=CARTESIAN_POINT ( 'NONE',  ( -336.3521761649654422, -174.5186198893880771, 29.74944317415823392 ) ) ;
#39771=ORIENTED_EDGE ( 'NONE', *, *, #35249, .F. ) ;
#39772=PLANE ( 'NONE',  #45233 ) ;
#39773=AXIS2_PLACEMENT_3D ( 'NONE', #9402, #25429, #16785 ) ;
#39774=EDGE_CURVE ( 'NONE', #50591, #29857, #30145, .T. ) ;
#39785=EDGE_CURVE ( 'NONE', #15240, #50991, #41964, .T. ) ;
#39796=CARTESIAN_POINT ( 'NONE',  ( -336.3521761649654422, -106.8245764869328980, 56.65561927337994064 ) ) ;
#39798=CARTESIAN_POINT ( 'NONE',  ( -332.3517673607765914, -65.12692710742291524, -8.732051761643681687 ) ) ;
#39806=EDGE_CURVE ( 'NONE', #10115, #50532, #46189, .T. ) ;
#39812=EDGE_CURVE ( 'NONE', #42957, #13339, #14376, .T. ) ;
#39819=CARTESIAN_POINT ( 'NONE',  ( -332.3517673607765914, -77.52356969168074841, 38.55084767037245541 ) ) ;
#39821=CARTESIAN_POINT ( 'NONE',  ( -336.3521761649654422, -179.2447759217480154, -19.39547174791710660 ) ) ;
#39823=CARTESIAN_POINT ( 'NONE',  ( -336.3521761649654422, -83.15397741537739762, 43.07972642080338233 ) ) ;
#39824=EDGE_LOOP ( 'NONE', ( #51924, #9351, #14135, #44642 ) ) ;
#39829=PLANE ( 'NONE',  #12354 ) ;
#39834=VERTEX_POINT ( 'NONE', #26717 ) ;
#39839=EDGE_LOOP ( 'NONE', ( #36754, #46681, #14182, #17086 ) ) ;
#39841=COLOUR_RGB ( '', 0.31764706, 0.68627451, 0.89019608) ;
#39842=CARTESIAN_POINT ( 'NONE',  ( -339.1964088526558498, -131.1080185721124849, 58.50955523165764305 ) ) ;
#39843=CARTESIAN_POINT ( 'NONE',  ( -339.1964088526558498, -138.1050951016783301, 57.16590939599346655 ) ) ;
#39845=LINE ( 'NONE', #169, #45757 ) ;
#39847=DIRECTION ( 'NONE',  ( 0.000000000000000000, 0.000000000000000000, 1.000000000000000000 ) ) ;
#39849=AXIS2_PLACEMENT_3D ( 'NONE', #15879, #31112, #27940 ) ;
#39854=CARTESIAN_POINT ( 'NONE',  ( -332.3517673607765914, -160.6539403396202772, 45.90766452162722544 ) ) ;
#39863=EDGE_LOOP ( 'NONE', ( #44963, #28720, #24587, #16005 ) ) ;
#39866=EDGE_CURVE ( 'NONE', #14596, #15649, #39047, .T. ) ;
#39867=LINE ( 'NONE', #11763, #47882 ) ;
#39869=AXIS2_PLACEMENT_3D ( 'NONE', #13320, #21464, #35346 ) ;
#39875=AXIS2_PLACEMENT_3D ( 'NONE', #46496, #30705, #49921 ) ;
#39879=LINE ( 'NONE', #44100, #4937 ) ;
#39881=ORIENTED_EDGE ( 'NONE', *, *, #21697, .F. ) ;
#39884=ORIENTED_EDGE ( 'NONE', *, *, #25945, .T. ) ;
#39885=VERTEX_POINT ( 'NONE', #23550 ) ;
#39886=EDGE_CURVE ( 'NONE', #46591, #26732, #3844, .T. ) ;
#39891=DIRECTION ( 'NONE',  ( 0.000000000000000000, 0.000000000000000000, 1.000000000000000000 ) ) ;
#39903=CARTESIAN_POINT ( 'NONE',  ( -339.1964088526558498, -71.02573290043838483, 26.97593913775504504 ) ) ;
#39905=VECTOR ( 'NONE', #45043, 1000.000000000000000 ) ;
#39914=CARTESIAN_POINT ( 'NONE',  ( -336.3521761649654422, -181.1761995186066088, -12.53476669029101842 ) ) ;
#39916=CIRCLE ( 'NONE', #20654, 60.00000000000000000 ) ;
#39919=VERTEX_POINT ( 'NONE', #35899 ) ;
#39923=ADVANCED_FACE ( 'NONE', ( #51427 ), #51950, .T. ) ;
#39930=EDGE_CURVE ( 'NONE', #40473, #3020, #46700, .T. ) ;
#39932=ORIENTED_EDGE ( 'NONE', *, *, #49473, .F. ) ;
#39937=ORIENTED_EDGE ( 'NONE', *, *, #41098, .T. ) ;
#39943=LINE ( 'NONE', #7132, #43688 ) ;
#39944=LINE ( 'NONE', #16312, #40913 ) ;
#39945=DIRECTION ( 'NONE',  ( -0.000000000000000000, 0.1205366802553337752, 0.9927088740980526405 ) ) ;
#39946=VERTEX_POINT ( 'NONE', #39322 ) ;
#39950=CARTESIAN_POINT ( 'NONE',  ( -336.3521761649654422, -70.03480886230919111, 25.08789112700620194 ) ) ;
#39953=ORIENTED_EDGE ( 'NONE', *, *, #10944, .T. ) ;
#39957=VECTOR ( 'NONE', #18567, 1000.000000000000000 ) ;
#39958=CARTESIAN_POINT ( 'NONE',  ( -332.3517673607765914, -66.84438072661991725, -16.67542351306652648 ) ) ;
#39959=CARTESIAN_POINT ( 'NONE',  ( -305.0000000000000568, -109.6270296344161750, -58.37414404713471328 ) ) ;
#39961=VERTEX_POINT ( 'NONE', #27744 ) ;
#39970=LINE ( 'NONE', #20020, #10808 ) ;
#39971=PLANE ( 'NONE',  #20599 ) ;
#39972=ORIENTED_EDGE ( 'NONE', *, *, #15698, .T. ) ;
#39975=VECTOR ( 'NONE', #9222, 1000.000000000000000 ) ;
#39976=VECTOR ( 'NONE', #7932, 1000.000000000000000 ) ;
#39978=CARTESIAN_POINT ( 'NONE',  ( -330.4913330509368166, -123.5000000000000284, 0.000000000000000000 ) ) ;
#39982=CARTESIAN_POINT ( 'NONE',  ( -332.3517673607765914, -149.9277501395804677, 53.86626052140529453 ) ) ;
#39983=CARTESIAN_POINT ( 'NONE',  ( -339.1964088526558498, -178.8432607619609485, -20.45418021416653076 ) ) ;
#39987=VECTOR ( 'NONE', #45753, 1000.000000000000000 ) ;
#39990=DIRECTION ( 'NONE',  ( 0.000000000000000000, 0.9927088740980548609, 0.1205366802553164696 ) ) ;
#39991=EDGE_LOOP ( 'NONE', ( #10632, #15594, #46220, #15988 ) ) ;
#39992=VECTOR ( 'NONE', #28195, 999.9999999999998863 ) ;
#39996=ADVANCED_FACE ( 'NONE', ( #15682, #8041, #44036, #48774, #24328, #16455, #20121, #32731, #16975, #24580, #32474, #4355, #21165, #40867, #40334, #4110, #48250, #16192, #49027, #24082, #45102, #48526, #928, #12743, #28768, #4614, #36150, #41132, #44821, #36938, #28002, #40093, #44560, #36404, #9089, #147, #32208, #12500, #12230, #5150, #28267, #28515, #8547, #44316, #37188, #8306, #25121, #20379, #40597, #399, #11969, #36678 ), #20642, .T. ) ;
#39999=AXIS2_PLACEMENT_3D ( 'NONE', #12576, #7357, #3923 ) ;
#40000=CARTESIAN_POINT ( 'NONE',  ( -339.1964088526558498, -66.33409060400673241, -14.60509510167901404 ) ) ;
#40002=ORIENTED_EDGE ( 'NONE', *, *, #44320, .F. ) ;
#40004=VERTEX_POINT ( 'NONE', #29035 ) ;
#40005=DIRECTION ( 'NONE',  ( 0.000000000000000000, 0.9709418174260534551, 0.2393156642875516327 ) ) ;
#40006=LINE ( 'NONE', #35818, #48501 ) ;
#40011=ORIENTED_EDGE ( 'NONE', *, *, #5861, .T. ) ;
#40012=LINE ( 'NONE', #4038, #25796 ) ;
#40016=VECTOR ( 'NONE', #50749, 1000.000000000000000 ) ;
#40018=DIRECTION ( 'NONE',  ( -1.000000000000000000, 1.036104688092334944E-14, -1.258058860540643439E-15 ) ) ;
#40022=FACE_OUTER_BOUND ( 'NONE', #3581, .T. ) ;
#40023=DIRECTION ( 'NONE',  ( 0.000000000000000000, 0.000000000000000000, -1.000000000000000000 ) ) ;
#40025=ORIENTED_EDGE ( 'NONE', *, *, #11802, .T. ) ;
#40029=DIRECTION ( 'NONE',  ( 1.043714542225393697E-14, 0.8229838658936495799, -0.5680647467311656929 ) ) ;
#40032=CARTESIAN_POINT ( 'NONE',  ( -332.3517673607765914, -114.7679482383557144, 58.37307289257701370 ) ) ;
#40033=VECTOR ( 'NONE', #28650, 1000.000000000000114 ) ;
#40034=CARTESIAN_POINT ( 'NONE',  ( -332.3517673607765914, -125.1322888500942270, -59.00000000000002132 ) ) ;
#40035=DIRECTION ( 'NONE',  ( 1.000000000000000000, 0.000000000000000000, 0.000000000000000000 ) ) ;
#40037=LINE ( 'NONE', #48208, #35986 ) ;
#40038=AXIS2_PLACEMENT_3D ( 'NONE', #4543, #20565, #9272 ) ;
#40040=EDGE_LOOP ( 'NONE', ( #6257, #30211, #6359, #38624 ) ) ;
#40046=EDGE_CURVE ( 'NONE', #12833, #40482, #17753, .T. ) ;
#40055=DIRECTION ( 'NONE',  ( -1.000000000000000000, 0.000000000000000000, 0.000000000000000000 ) ) ;
#40060=AXIS2_PLACEMENT_3D ( 'NONE', #16016, #48327, #24663 ) ;
#40062=CARTESIAN_POINT ( 'NONE',  ( 0.000000000000000000, -79.33786585790510060, -39.12423683620700388 ) ) ;
#40074=EDGE_CURVE ( 'NONE', #35455, #18186, #33767, .T. ) ;
#40081=VECTOR ( 'NONE', #9610, 1000.000000000000000 ) ;
#40082=EDGE_CURVE ( 'NONE', #27333, #6252, #43812, .T. ) ;
#40084=FACE_OUTER_BOUND ( 'NONE', #51101, .T. ) ;
#40086=EDGE_LOOP ( 'NONE', ( #32044, #27671, #36027, #27277 ) ) ;
#40093=FACE_BOUND ( 'NONE', #14306, .T. ) ;
#40096=EDGE_CURVE ( 'NONE', #49147, #33399, #6908, .T. ) ;
#40110=DIRECTION ( 'NONE',  ( 0.000000000000000000, 0.000000000000000000, -1.000000000000000000 ) ) ;
#40111=ORIENTED_EDGE ( 'NONE', *, *, #4205, .F. ) ;
#40116=CARTESIAN_POINT ( 'NONE',  ( -339.1964088526558498, -130.1153096980153236, -58.63009191191284941 ) ) ;
#40118=EDGE_CURVE ( 'NONE', #38437, #2241, #41388, .T. ) ;
#40124=LINE ( 'NONE', #23578, #30506 ) ;
#40125=CARTESIAN_POINT ( 'NONE',  ( -339.1964088526558498, -178.4886558749180949, 21.38919645685277970 ) ) ;
#40133=DIRECTION ( 'NONE',  ( 0.000000000000000000, 0.9709418174260526779, 0.2393156642875547968 ) ) ;
#40134=EDGE_CURVE ( 'NONE', #33953, #42476, #3270, .T. ) ;
#40140=AXIS2_PLACEMENT_3D ( 'NONE', #36526, #47611, #11591 ) ;
#40142=CARTESIAN_POINT ( 'NONE',  ( -336.3521761649654422, -68.91285928486892942, -22.44790492310182017 ) ) ;
#40144=AXIS2_PLACEMENT_3D ( 'NONE', #7128, #15031, #42611 ) ;
#40146=DIRECTION ( 'NONE',  ( -8.718379230999705894E-17, 0.8229838658936536877, -0.5680647467311596976 ) ) ;
#40148=ADVANCED_FACE ( 'NONE', ( #19304 ), #18651, .T. ) ;
#40157=LINE ( 'NONE', #40400, #51094 ) ;
#40160=CARTESIAN_POINT ( 'NONE',  ( -332.3517673607765914, -177.3662605214052519, -26.42775013958060271 ) ) ;
#40161=DIRECTION ( 'NONE',  ( 1.000000000000000000, 0.000000000000000000, 0.000000000000000000 ) ) ;
#40164=LINE ( 'NONE', #214, #27332 ) ;
#40173=ORIENTED_EDGE ( 'NONE', *, *, #7847, .T. ) ;
#40178=CARTESIAN_POINT ( 'NONE',  ( -336.3521761649654422, -88.64083255475578937, 47.62880233550460218 ) ) ;
#40189=CARTESIAN_POINT ( 'NONE',  ( -330.4913330509368166, -131.1080185721132807, -58.50955523165751515 ) ) ;
#40194=DIRECTION ( 'NONE',  ( 0.000000000000000000, 0.4647231720437789981, 0.8854560256532044704 ) ) ;
#40196=EDGE_LOOP ( 'NONE', ( #4910, #42878, #16287, #8862 ) ) ;
#40201=ADVANCED_FACE ( 'NONE', ( #50582 ), #11660, .F. ) ;
#40208=VECTOR ( 'NONE', #46751, 1000.000000000000000 ) ;
#40209=ORIENTED_EDGE ( 'NONE', *, *, #43627, .T. ) ;
#40210=DIRECTION ( 'NONE',  ( -0.000000000000000000, 0.9709418174260519008, -0.2393156642875582940 ) ) ;
#40211=VECTOR ( 'NONE', #6506, 1000.000000000000000 ) ;
#40214=CARTESIAN_POINT ( 'NONE',  ( -332.3517673607765914, -173.5513585866778214, -31.34948880313881503 ) ) ;
#40215=DIRECTION ( 'NONE',  ( -1.000000000000000000, 1.258058860540389820E-15, -1.036104688092337784E-14 ) ) ;
#40216=CARTESIAN_POINT ( 'NONE',  ( -339.1964088526558498, -115.8919814278862503, 58.50955523165745831 ) ) ;
#40217=ORIENTED_EDGE ( 'NONE', *, *, #32585, .F. ) ;
#40220=DIRECTION ( 'NONE',  ( -0.000000000000000000, 0.3546048870425463906, 0.9350162426854107256 ) ) ;
#40225=LINE ( 'NONE', #544, #18112 ) ;
#40226=ORIENTED_EDGE ( 'NONE', *, *, #31761, .F. ) ;
#40228=DIRECTION ( 'NONE',  ( 0.000000000000000000, 0.8854560256532110207, 0.4647231720437664526 ) ) ;
#40229=CARTESIAN_POINT ( 'NONE',  ( -336.3521761649653854, -63.76276212672765809, 5.609136410542458151 ) ) ;
#40232=CARTESIAN_POINT ( 'NONE',  ( -339.1964088526558498, -123.5000000000000284, 0.000000000000000000 ) ) ;
#40233=DIRECTION ( 'NONE',  ( 0.000000000000000000, -0.7485107481711046340, -0.6631226582407911962 ) ) ;
#40241=VECTOR ( 'NONE', #11700, 1000.000000000000000 ) ;
#40250=DIRECTION ( 'NONE',  ( -0.000000000000000000, 0.6631226582408016323, 0.7485107481710953081 ) ) ;
#40254=DIRECTION ( 'NONE',  ( 0.000000000000000000, -0.3546048870425235200, 0.9350162426854194964 ) ) ;
#40257=DIRECTION ( 'NONE',  ( 0.000000000000000000, -1.503427012513232710E-14, 1.000000000000000000 ) ) ;
#40261=DIRECTION ( 'NONE',  ( 0.000000000000000000, 0.000000000000000000, 1.000000000000000000 ) ) ;
#40262=FACE_OUTER_BOUND ( 'NONE', #23882, .T. ) ;
#40263=DIRECTION ( 'NONE',  ( 1.000000000000000000, 0.000000000000000000, -0.000000000000000000 ) ) ;
#40265=VERTEX_POINT ( 'NONE', #42939 ) ;
#40266=EDGE_LOOP ( 'NONE', ( #14144, #2930, #39707, #15521 ) ) ;
#40271=AXIS2_PLACEMENT_3D ( 'NONE', #51529, #7124, #23159 ) ;
#40272=DIRECTION ( 'NONE',  ( 0.000000000000000000, 0.000000000000000000, 1.000000000000000000 ) ) ;
#40285=LINE ( 'NONE', #39765, #19967 ) ;
#40293=AXIS2_PLACEMENT_3D ( 'NONE', #21883, #6634, #22655 ) ;
#40294=VECTOR ( 'NONE', #20540, 1000.000000000000000 ) ;
#40298=DIRECTION ( 'NONE',  ( 0.000000000000000000, -9.714451465470119729E-15, -1.000000000000000000 ) ) ;
#40299=LINE ( 'NONE', #24806, #35162 ) ;
#40300=ADVANCED_FACE ( 'NONE', ( #8234 ), #27939, .F. ) ;
#40303=LINE ( 'NONE', #4320, #4720 ) ;
#40306=DIRECTION ( 'NONE',  ( 0.000000000000000000, -1.000000000000000000, 1.047444401652940007E-14 ) ) ;
#40307=EDGE_LOOP ( 'NONE', ( #12791, #7302, #11912, #1445 ) ) ;
#40310=ORIENTED_EDGE ( 'NONE', *, *, #49242, .F. ) ;
#40317=LINE ( 'NONE', #4336, #33550 ) ;
#40319=CARTESIAN_POINT ( 'NONE',  ( -330.4913330509368166, -178.8432607619606358, 20.45418021416736565 ) ) ;
#40320=FACE_OUTER_BOUND ( 'NONE', #29751, .T. ) ;
#40324=VECTOR ( 'NONE', #50548, 1000.000000000000000 ) ;
#40327=ORIENTED_EDGE ( 'NONE', *, *, #1395, .F. ) ;
#40333=DIRECTION ( 'NONE',  ( -0.000000000000000000, 0.3546048870425426158, 0.9350162426854120579 ) ) ;
#40334=FACE_BOUND ( 'NONE', #13999, .T. ) ;
#40335=CARTESIAN_POINT ( 'NONE',  ( -332.3517673607765914, -123.5000000000000284, 0.000000000000000000 ) ) ;
#40336=ORIENTED_EDGE ( 'NONE', *, *, #4236, .F. ) ;
#40341=ORIENTED_EDGE ( 'NONE', *, *, #42903, .F. ) ;
#40346=CARTESIAN_POINT ( 'NONE',  ( -336.3521761649653854, -182.8437365148560616, 8.849911663702917153 ) ) ;
#40347=CARTESIAN_POINT ( 'NONE',  ( -339.1964088526558498, -90.39567187580880159, -48.84008046109142498 ) ) ;
#40348=LINE ( 'NONE', #16204, #51973 ) ;
#40350=EDGE_CURVE ( 'NONE', #33085, #43701, #12679, .T. ) ;
#40356=ADVANCED_FACE ( 'NONE', ( #19795 ), #8741, .F. ) ;
#40359=CARTESIAN_POINT ( 'NONE',  ( -336.3521761649654422, -75.87119766449505676, -34.85916744524372746 ) ) ;
#40363=LINE ( 'NONE', #4381, #7762 ) ;
#40364=ORIENTED_EDGE ( 'NONE', *, *, #26296, .F. ) ;
#40365=CARTESIAN_POINT ( 'NONE',  ( -336.3521761649654422, -97.52665284734005979, -53.00046796564681983 ) ) ;
#40370=ORIENTED_EDGE ( 'NONE', *, *, #20809, .F. ) ;
#40371=VECTOR ( 'NONE', #41358, 1000.000000000000000 ) ;
#40372=CARTESIAN_POINT ( 'NONE',  ( -305.0000000000000568, -89.82879061784626629, 49.66134974749640207 ) ) ;
#40373=FACE_OUTER_BOUND ( 'NONE', #5765, .T. ) ;
#40377=EDGE_CURVE ( 'NONE', #51496, #26301, #13623, .T. ) ;
#40382=VERTEX_POINT ( 'NONE', #36086 ) ;
#40384=ORIENTED_EDGE ( 'NONE', *, *, #40082, .F. ) ;
#40385=ORIENTED_EDGE ( 'NONE', *, *, #11709, .T. ) ;
#40394=EDGE_CURVE ( 'NONE', #28183, #23609, #48186, .T. ) ;
#40396=EDGE_CURVE ( 'NONE', #48950, #48787, #34703, .T. ) ;
#40397=VECTOR ( 'NONE', #5172, 1000.000000000000000 ) ;
#40400=CARTESIAN_POINT ( 'NONE',  ( -336.3521761649654422, -141.9604555052315220, 56.09938080879057765 ) ) ;
#40401=CARTESIAN_POINT ( 'NONE',  ( -339.1964088526558498, -144.8891964568526305, -54.98865587491811624 ) ) ;
#40402=EDGE_LOOP ( 'NONE', ( #44053, #48627, #14519, #34533 ) ) ;
#40405=VERTEX_POINT ( 'NONE', #27336 ) ;
#40410=CARTESIAN_POINT ( 'NONE',  ( -339.1964088526558498, -137.3729703655831429, 58.37414404713489091 ) ) ;
#40412=CARTESIAN_POINT ( 'NONE',  ( -332.3517673607765914, -161.4024510877913485, 45.24454186338643780 ) ) ;
#40414=ORIENTED_EDGE ( 'NONE', *, *, #50243, .T. ) ;
#40422=LINE ( 'NONE', #20208, #24545 ) ;
#40426=CARTESIAN_POINT ( 'NONE',  ( -330.4913330509368166, -108.8949048983204904, 57.16590939599316812 ) ) ;
#40427=DIRECTION ( 'NONE',  ( 0.000000000000000000, 0.000000000000000000, 1.000000000000000000 ) ) ;
#40430=EDGE_CURVE ( 'NONE', #49256, #39057, #23411, .T. ) ;
#40431=ORIENTED_EDGE ( 'NONE', *, *, #13811, .F. ) ;
#40432=CARTESIAN_POINT ( 'NONE',  ( -339.1964088526558498, -145.2430625708876732, -55.92172413327814695 ) ) ;
#40433=DIRECTION ( 'NONE',  ( 0.000000000000000000, 0.9350162426854146114, -0.3546048870425363986 ) ) ;
#40439=VECTOR ( 'NONE', #47305, 1000.000000000000000 ) ;
#40441=DIRECTION ( 'NONE',  ( -8.718379230999705894E-17, -0.1205366802553303057, -0.9927088740980530845 ) ) ;
#40442=ORIENTED_EDGE ( 'NONE', *, *, #13435, .F. ) ;
#40445=EDGE_LOOP ( 'NONE', ( #30028, #13618, #8675, #34701 ) ) ;
#40446=EDGE_CURVE ( 'NONE', #27774, #6375, #15019, .T. ) ;
#40454=LINE ( 'NONE', #20490, #36704 ) ;
#40464=EDGE_CURVE ( 'NONE', #30731, #37301, #7763, .T. ) ;
#40472=DIRECTION ( 'NONE',  ( -0.000000000000000000, 0.3546048870425363986, 0.9350162426854146114 ) ) ;
#40473=VERTEX_POINT ( 'NONE', #3676 ) ;
#40476=FACE_OUTER_BOUND ( 'NONE', #21167, .T. ) ;
#40480=CARTESIAN_POINT ( 'NONE',  ( -330.4913330509368166, -182.5000000000000568, 0.4999999999999549249 ) ) ;
#40482=VERTEX_POINT ( 'NONE', #27846 ) ;
#40483=AXIS2_PLACEMENT_3D ( 'NONE', #48632, #21018, #17355 ) ;
#40489=DIRECTION ( 'NONE',  ( 0.000000000000000000, -0.6631226582407965253, -0.7485107481711000821 ) ) ;
#40495=AXIS2_PLACEMENT_3D ( 'NONE', #47695, #15371, #31379 ) ;
#40496=EDGE_CURVE ( 'NONE', #23459, #51539, #7878, .T. ) ;
#40503=DIRECTION ( 'NONE',  ( 1.000000000000000000, 0.000000000000000000, -0.000000000000000000 ) ) ;
#40504=CARTESIAN_POINT ( 'NONE',  ( -336.3521761649654422, -179.5993808087905279, -18.46045550523168899 ) ) ;
#40505=PLANE ( 'NONE',  #26419 ) ;
#40508=DIRECTION ( 'NONE',  ( -0.000000000000000000, -0.3546048870425396182, -0.9350162426854132791 ) ) ;
#40509=CARTESIAN_POINT ( 'NONE',  ( -339.1964088526558498, -162.9984922102927385, -43.83057281297435992 ) ) ;
#40518=ORIENTED_EDGE ( 'NONE', *, *, #31900, .T. ) ;
#40519=ORIENTED_EDGE ( 'NONE', *, *, #35981, .F. ) ;
#40522=PLANE ( 'NONE',  #26966 ) ;
#40523=DIRECTION ( 'NONE',  ( -1.000000000000000000, 0.000000000000000000, 0.000000000000000000 ) ) ;
#40524=AXIS2_PLACEMENT_3D ( 'NONE', #4456, #21007, #40967 ) ;
#40528=ORIENTED_EDGE ( 'NONE', *, *, #37465, .F. ) ;
#40531=DIRECTION ( 'NONE',  ( -0.000000000000000000, 1.047444401652940007E-14, 1.000000000000000000 ) ) ;
#40534=DIRECTION ( 'NONE',  ( 0.000000000000000000, 0.4647231720437631775, -0.8854560256532126861 ) ) ;
#40536=ORIENTED_EDGE ( 'NONE', *, *, #27247, .F. ) ;
#40543=VERTEX_POINT ( 'NONE', #25383 ) ;
#40547=EDGE_CURVE ( 'NONE', #39299, #3275, #9102, .T. ) ;
#40552=CARTESIAN_POINT ( 'NONE',  ( 0.000000000000000000, -144.4216883355091170, 55.16595831843969933 ) ) ;
#40553=CARTESIAN_POINT ( 'NONE',  ( -330.4913330509368166, -79.00630452878421295, 38.74998146212088557 ) ) ;
#40557=ORIENTED_EDGE ( 'NONE', *, *, #45451, .T. ) ;
#40560=VERTEX_POINT ( 'NONE', #21178 ) ;
#40564=EDGE_CURVE ( 'NONE', #41391, #11859, #32990, .T. ) ;
#40574=VERTEX_POINT ( 'NONE', #49040 ) ;
#40579=ORIENTED_EDGE ( 'NONE', *, *, #28380, .F. ) ;
#40581=ORIENTED_EDGE ( 'NONE', *, *, #6108, .F. ) ;
#40586=DIRECTION ( 'NONE',  ( -0.000000000000000000, -0.2393156642875482742, 0.9709418174260544543 ) ) ;
#40589=ORIENTED_EDGE ( 'NONE', *, *, #3341, .F. ) ;
#40590=ADVANCED_FACE ( 'NONE', ( #41875 ), #33205, .T. ) ;
#40592=ORIENTED_EDGE ( 'NONE', *, *, #11802, .F. ) ;
#40593=CARTESIAN_POINT ( 'NONE',  ( -332.3517673607765914, -110.9652333097088217, -57.67619951860654481 ) ) ;
#40597=FACE_BOUND ( 'NONE', #34636, .T. ) ;
#40598=DIRECTION ( 'NONE',  ( 0.000000000000000000, -0.5680647467311485954, 0.8229838658936613482 ) ) ;
#40599=ORIENTED_EDGE ( 'NONE', *, *, #22902, .F. ) ;
#40600=VECTOR ( 'NONE', #1767, 1000.000000000000000 ) ;
#40602=CARTESIAN_POINT ( 'NONE',  ( -339.1964088526558498, -167.9936954712156592, -38.74998146212110584 ) ) ;
#40606=EDGE_CURVE ( 'NONE', #15472, #43725, #44723, .T. ) ;
#40608=DIRECTION ( 'NONE',  ( 0.000000000000000000, 7.100801428331730794E-14, -1.000000000000000000 ) ) ;
#40611=CARTESIAN_POINT ( 'NONE',  ( -332.3517673607765914, -181.7525362123217292, 9.724760635742144999 ) ) ;
#40617=VECTOR ( 'NONE', #37384, 1000.000000000000000 ) ;
#40618=LINE ( 'NONE', #24606, #38195 ) ;
#40619=AXIS2_PLACEMENT_3D ( 'NONE', #37017, #24669, #13370 ) ;
#40621=CARTESIAN_POINT ( 'NONE',  ( -332.3517673607765914, -181.4155151828941825, -11.56382487286496463 ) ) ;
#40631=ORIENTED_EDGE ( 'NONE', *, *, #21636, .F. ) ;
#40636=DIRECTION ( 'NONE',  ( 0.000000000000000000, 0.000000000000000000, -1.000000000000000000 ) ) ;
#40641=DIRECTION ( 'NONE',  ( -1.000000000000000000, 0.000000000000000000, 0.000000000000000000 ) ) ;
#40642=VERTEX_POINT ( 'NONE', #29267 ) ;
#40643=EDGE_CURVE ( 'NONE', #51592, #28874, #5110, .T. ) ;
#40660=ORIENTED_EDGE ( 'NONE', *, *, #43785, .F. ) ;
#40661=DIRECTION ( 'NONE',  ( -1.000000000000000000, 0.000000000000000000, 0.000000000000000000 ) ) ;
#40662=PLANE ( 'NONE',  #25602 ) ;
#40664=ORIENTED_EDGE ( 'NONE', *, *, #2585, .F. ) ;
#40666=DIRECTION ( 'NONE',  ( 0.000000000000000000, -0.9350162426854169428, -0.3546048870425300148 ) ) ;
#40668=DIRECTION ( 'NONE',  ( -0.000000000000000000, 0.000000000000000000, 1.000000000000000000 ) ) ;
#40675=AXIS2_PLACEMENT_3D ( 'NONE', #1114, #863, #49502 ) ;
#40681=PLANE ( 'NONE',  #2333 ) ;
#40682=LINE ( 'NONE', #19957, #4796 ) ;
#40683=DIRECTION ( 'NONE',  ( -0.000000000000000000, -0.7485107481710953081, 0.6631226582408016323 ) ) ;
#40685=DIRECTION ( 'NONE',  ( 0.000000000000000000, 0.9350162426854194964, 0.3546048870425235200 ) ) ;
#40686=DIRECTION ( 'NONE',  ( -0.000000000000000000, 1.047444401652940007E-14, 1.000000000000000000 ) ) ;
#40692=PLANE ( 'NONE',  #45009 ) ;
#40696=ADVANCED_FACE ( 'NONE', ( #13762 ), #50813, .T. ) ;
#40697=CARTESIAN_POINT ( 'NONE',  ( -330.4913330509368166, -109.8658467157472813, -57.40522506028090532 ) ) ;
#40701=EDGE_CURVE ( 'NONE', #48252, #30276, #14555, .T. ) ;
#40702=ORIENTED_EDGE ( 'NONE', *, *, #50629, .F. ) ;
#40712=VERTEX_POINT ( 'NONE', #21918 ) ;
#40715=AXIS2_PLACEMENT_3D ( 'NONE', #24721, #44695, #8174 ) ;
#40717=ORIENTED_EDGE ( 'NONE', *, *, #22482, .T. ) ;
#40718=EDGE_CURVE ( 'NONE', #6765, #41945, #18748, .T. ) ;
#40722=ADVANCED_FACE ( 'NONE', ( #34258 ), #37941, .T. ) ;
#40724=CARTESIAN_POINT ( 'NONE',  ( -170.0000000000000284, -123.5000000000000284, 0.000000000000000000 ) ) ;
#40727=DIRECTION ( 'NONE',  ( -1.000000000000000000, -0.000000000000000000, -0.000000000000000000 ) ) ;
#40731=ORIENTED_EDGE ( 'NONE', *, *, #43785, .T. ) ;
#40732=AXIS2_PLACEMENT_3D ( 'NONE', #34493, #35016, #14541 ) ;
#40734=VECTOR ( 'NONE', #3219, 1000.000000000000000 ) ;
#40738=EDGE_LOOP ( 'NONE', ( #43771, #39256, #29919, #8893 ) ) ;
#40740=FACE_OUTER_BOUND ( 'NONE', #10493, .T. ) ;
#40747=DIRECTION ( 'NONE',  ( -0.000000000000000000, -0.9350162426854158326, -0.3546048870425331234 ) ) ;
#40750=DIRECTION ( 'NONE',  ( -0.000000000000000000, -0.2393156642875615969, -0.9709418174260511236 ) ) ;
#40753=EDGE_LOOP ( 'NONE', ( #49170, #14584, #27898, #13087 ) ) ;
#40756=VECTOR ( 'NONE', #41190, 1000.000000000000114 ) ;
#40757=EDGE_CURVE ( 'NONE', #26962, #36738, #22440, .T. ) ;
#40759=CARTESIAN_POINT ( 'NONE',  ( 0.000000000000000000, -172.0560480877254861, 33.51582005713859758 ) ) ;
#40761=DIRECTION ( 'NONE',  ( -1.000000000000000000, -0.000000000000000000, -0.000000000000000000 ) ) ;
#40766=CARTESIAN_POINT ( 'NONE',  ( -336.3521761649654422, -155.6724726690323450, 49.48329383994676078 ) ) ;
#40770=AXIS2_PLACEMENT_3D ( 'NONE', #26807, #18423, #42586 ) ;
#40774=AXIS2_PLACEMENT_3D ( 'NONE', #45750, #37333, #9745 ) ;
#40776=ORIENTED_EDGE ( 'NONE', *, *, #31033, .F. ) ;
#40778=DIRECTION ( 'NONE',  ( 1.000000000000000000, 0.000000000000000000, 0.000000000000000000 ) ) ;
#40779=EDGE_LOOP ( 'NONE', ( #39771, #12067 ) ) ;
#40780=ORIENTED_EDGE ( 'NONE', *, *, #1886, .T. ) ;
#40781=EDGE_CURVE ( 'NONE', #41973, #29433, #37688, .T. ) ;
#40785=AXIS2_PLACEMENT_3D ( 'NONE', #13251, #28735, #9313 ) ;
#40786=EDGE_CURVE ( 'NONE', #33439, #47197, #26104, .T. ) ;
#40792=ADVANCED_FACE ( 'NONE', ( #26875 ), #31594, .F. ) ;
#40796=ORIENTED_EDGE ( 'NONE', *, *, #916, .T. ) ;
#40801=ORIENTED_EDGE ( 'NONE', *, *, #43214, .T. ) ;
#40806=VECTOR ( 'NONE', #4646, 999.9999999999998863 ) ;
#40807=ORIENTED_EDGE ( 'NONE', *, *, #35189, .F. ) ;
#40809=VECTOR ( 'NONE', #28737, 1000.000000000000000 ) ;
#40810=DIRECTION ( 'NONE',  ( 0.000000000000000000, 0.7485107481710977506, -0.6631226582407989678 ) ) ;
#40813=AXIS2_PLACEMENT_3D ( 'NONE', #17653, #1075, #17127 ) ;
#40817=DIRECTION ( 'NONE',  ( 0.000000000000000000, 1.251313867337936767E-13, 1.000000000000000000 ) ) ;
#40818=ORIENTED_EDGE ( 'NONE', *, *, #41705, .T. ) ;
#40820=ORIENTED_EDGE ( 'NONE', *, *, #16642, .F. ) ;
#40824=CARTESIAN_POINT ( 'NONE',  ( -332.3517673607765914, -142.2945752170892035, 56.98038208374156000 ) ) ;
#40826=VECTOR ( 'NONE', #49901, 999.9999999999998863 ) ;
#40834=CARTESIAN_POINT ( 'NONE',  ( -336.3521761649654422, -121.8677111499054320, 59.00000000000001421 ) ) ;
#40839=EDGE_LOOP ( 'NONE', ( #42412, #10274, #24370, #42120 ) ) ;
#40843=ORIENTED_EDGE ( 'NONE', *, *, #43583, .F. ) ;
#40844=CARTESIAN_POINT ( 'NONE',  ( -339.1964088526558498, -84.00150778970699150, 43.83057281297409702 ) ) ;
#40845=PLANE ( 'NONE',  #795 ) ;
#40847=VECTOR ( 'NONE', #647, 999.9999999999998863 ) ;
#40848=ORIENTED_EDGE ( 'NONE', *, *, #13820, .T. ) ;
#40849=CARTESIAN_POINT ( 'NONE',  ( -336.3521761649654422, -176.9651911376907094, -25.08789112700655721 ) ) ;
#40851=ORIENTED_EDGE ( 'NONE', *, *, #38686, .F. ) ;
#40859=EDGE_CURVE ( 'NONE', #11734, #14384, #11991, .T. ) ;
#40861=DIRECTION ( 'NONE',  ( -0.000000000000000000, -0.8229838658936575735, -0.5680647467311540355 ) ) ;
#40863=AXIS2_PLACEMENT_3D ( 'NONE', #37440, #8804, #41129 ) ;
#40865=CARTESIAN_POINT ( 'NONE',  ( -490.0000000000001137, -78.50000000000002842, -14.36509618646847386 ) ) ;
#40867=FACE_BOUND ( 'NONE', #901, .T. ) ;
#40869=DIRECTION ( 'NONE',  ( 0.000000000000000000, 0.4647231720437755564, 0.8854560256532062468 ) ) ;
#40874=DIRECTION ( 'NONE',  ( -1.000000000000000000, 0.000000000000000000, 0.000000000000000000 ) ) ;
#40876=ORIENTED_EDGE ( 'NONE', *, *, #18836, .F. ) ;
#40879=CARTESIAN_POINT ( 'NONE',  ( -332.3517673607765914, -123.5000000000000284, 0.000000000000000000 ) ) ;
#40881=ORIENTED_EDGE ( 'NONE', *, *, #48094, .F. ) ;
#40885=EDGE_LOOP ( 'NONE', ( #5881, #35784, #37001, #50292 ) ) ;
#40895=EDGE_CURVE ( 'NONE', #38101, #22193, #43063, .T. ) ;
#40897=CARTESIAN_POINT ( 'NONE',  ( -336.3521761649654422, -123.5000000000000284, 0.000000000000000000 ) ) ;
#40902=AXIS2_PLACEMENT_3D ( 'NONE', #6942, #42423, #38487 ) ;
#40905=FACE_OUTER_BOUND ( 'NONE', #48384, .T. ) ;
#40907=CIRCLE ( 'NONE', #24984, 5.000000000000001776 ) ;
#40908=DIRECTION ( 'NONE',  ( 0.000000000000000000, 0.9927088740980534176, -0.1205366802553268502 ) ) ;
#40912=ORIENTED_EDGE ( 'NONE', *, *, #50440, .F. ) ;
#40913=VECTOR ( 'NONE', #32321, 1000.000000000000000 ) ;
#40916=CARTESIAN_POINT ( 'NONE',  ( -336.3521761649654422, -65.82380048139334860, 12.53476669029061519 ) ) ;
#40918=ADVANCED_FACE ( 'NONE', ( #19763 ), #16100, .F. ) ;
#40921=ORIENTED_EDGE ( 'NONE', *, *, #50072, .T. ) ;
#40922=ORIENTED_EDGE ( 'NONE', *, *, #42830, .T. ) ;
#40928=ORIENTED_EDGE ( 'NONE', *, *, #15580, .T. ) ;
#40934=DIRECTION ( 'NONE',  ( 0.000000000000000000, -0.9927088740980530845, 0.1205366802553303196 ) ) ;
#40939=VECTOR ( 'NONE', #30573, 999.9999999999998863 ) ;
#40940=ORIENTED_EDGE ( 'NONE', *, *, #15698, .F. ) ;
#40949=EDGE_LOOP ( 'NONE', ( #51458, #11525, #269, #33905 ) ) ;
#40953=VERTEX_POINT ( 'NONE', #11105 ) ;
#40954=CARTESIAN_POINT ( 'NONE',  ( -330.4913330509368166, -64.50000000000000000, 0.4999999999999551470 ) ) ;
#40955=PLANE ( 'NONE',  #5544 ) ;
#40957=PLANE ( 'NONE',  #33391 ) ;
#40962=EDGE_CURVE ( 'NONE', #21654, #48787, #27133, .T. ) ;
#40964=DIRECTION ( 'NONE',  ( -1.000000000000000000, 0.000000000000000000, 0.000000000000000000 ) ) ;
#40967=DIRECTION ( 'NONE',  ( 0.000000000000000000, 0.000000000000000000, 1.000000000000000000 ) ) ;
#40971=EDGE_CURVE ( 'NONE', #50838, #8505, #19276, .T. ) ;
#40972=FACE_OUTER_BOUND ( 'NONE', #29010, .T. ) ;
#40976=PLANE ( 'NONE',  #11790 ) ;
#40977=CARTESIAN_POINT ( 'NONE',  ( -330.4913330509368166, -175.9742670995615015, -26.97593913775547136 ) ) ;
#40984=DIRECTION ( 'NONE',  ( -8.718379230999707126E-17, 0.8854560256532110207, 0.4647231720437664526 ) ) ;
#40986=ORIENTED_EDGE ( 'NONE', *, *, #51794, .T. ) ;
#40987=DIRECTION ( 'NONE',  ( 0.000000000000000000, 0.000000000000000000, 1.000000000000000000 ) ) ;
#41000=ORIENTED_EDGE ( 'NONE', *, *, #10908, .F. ) ;
#41009=EDGE_CURVE ( 'NONE', #38856, #11608, #16355, .T. ) ;
#41011=LINE ( 'NONE', #17386, #19136 ) ;
#41014=ORIENTED_EDGE ( 'NONE', *, *, #11224, .F. ) ;
#41017=CARTESIAN_POINT ( 'NONE',  ( -305.0000000000000568, -63.52220716707010695, -1.632288850093980725 ) ) ;
#41018=CARTESIAN_POINT ( 'NONE',  ( -336.3521761649654422, -141.9604555052315220, 56.09938080879057765 ) ) ;
#41019=FACE_OUTER_BOUND ( 'NONE', #38140, .T. ) ;
#41025=ORIENTED_EDGE ( 'NONE', *, *, #24088, .F. ) ;
#41029=AXIS2_PLACEMENT_3D ( 'NONE', #942, #48541, #16987 ) ;
#41034=CARTESIAN_POINT ( 'NONE',  ( -339.1964088526558498, -123.5000000000000284, 0.000000000000000000 ) ) ;
#41035=EDGE_CURVE ( 'NONE', #34925, #49907, #37091, .T. ) ;
#41037=DIRECTION ( 'NONE',  ( 1.000000000000000000, -0.000000000000000000, 0.000000000000000000 ) ) ;
#41039=VECTOR ( 'NONE', #44933, 1000.000000000000000 ) ;
#41041=CARTESIAN_POINT ( 'NONE',  ( -339.1964088526558498, -180.6659093959932250, 14.60509510167942437 ) ) ;
#41043=ORIENTED_EDGE ( 'NONE', *, *, #20498, .T. ) ;
#41044=AXIS2_PLACEMENT_3D ( 'NONE', #5149, #37900, #32207 ) ;
#41045=EDGE_LOOP ( 'NONE', ( #1809, #1674, #16299, #35757 ) ) ;
#41049=ORIENTED_EDGE ( 'NONE', *, *, #45926, .T. ) ;
#41050=CIRCLE ( 'NONE', #19232, 60.00000000000000000 ) ;
#41051=EDGE_LOOP ( 'NONE', ( #11406, #49380, #16143, #38446 ) ) ;
#41057=ORIENTED_EDGE ( 'NONE', *, *, #4115, .F. ) ;
#41062=ORIENTED_EDGE ( 'NONE', *, *, #10116, .T. ) ;
#41065=CARTESIAN_POINT ( 'NONE',  ( -336.3521761649654422, -146.8829211657874794, -54.23253582808848705 ) ) ;
#41068=EDGE_CURVE ( 'NONE', #30276, #15240, #12655, .T. ) ;
#41082=EDGE_CURVE ( 'NONE', #1973, #50621, #25528, .T. ) ;
#41085=CARTESIAN_POINT ( 'NONE',  ( -339.1964088526558498, -123.5000000000000284, 0.000000000000000000 ) ) ;
#41090=ADVANCED_FACE ( 'NONE', ( #22113 ), #5846, .F. ) ;
#41092=FACE_OUTER_BOUND ( 'NONE', #51616, .T. ) ;
#41098=EDGE_CURVE ( 'NONE', #22244, #14314, #21861, .T. ) ;
#41101=DIRECTION ( 'NONE',  ( -1.000000000000000000, 0.000000000000000000, -0.000000000000000000 ) ) ;
#41105=ORIENTED_EDGE ( 'NONE', *, *, #39632, .T. ) ;
#41115=ADVANCED_FACE ( 'NONE', ( #17917 ), #29724, .F. ) ;
#41116=LINE ( 'NONE', #17211, #19565 ) ;
#41119=VECTOR ( 'NONE', #51036, 1000.000000000000000 ) ;
#41120=DIRECTION ( 'NONE',  ( 0.000000000000000000, 0.000000000000000000, -1.000000000000000000 ) ) ;
#41123=LINE ( 'NONE', #13785, #5734 ) ;
#41126=VERTEX_POINT ( 'NONE', #38125 ) ;
#41129=DIRECTION ( 'NONE',  ( 0.000000000000000000, -0.5680647467311656929, -0.8229838658936495799 ) ) ;
#41131=LINE ( 'NONE', #6118, #30134 ) ;
#41132=FACE_BOUND ( 'NONE', #23054, .T. ) ;
#41135=ADVANCED_FACE ( 'NONE', ( #42331 ), #6093, .F. ) ;
#41138=VECTOR ( 'NONE', #23210, 1000.000000000000227 ) ;
#41139=ORIENTED_EDGE ( 'NONE', *, *, #19388, .T. ) ;
#41145=CARTESIAN_POINT ( 'NONE',  ( -305.0000000000000568, -130.2355952558264107, 59.62073260661670560 ) ) ;
#41146=DIRECTION ( 'NONE',  ( 0.000000000000000000, 0.000000000000000000, 1.000000000000000000 ) ) ;
#41147=CARTESIAN_POINT ( 'NONE',  ( -330.4913330509368166, -123.5000000000000284, 0.000000000000000000 ) ) ;
#41155=CARTESIAN_POINT ( 'NONE',  ( -330.4913330509368166, -108.8949048983204904, 57.16590939599316812 ) ) ;
#41159=ORIENTED_EDGE ( 'NONE', *, *, #33469, .F. ) ;
#41167=EDGE_LOOP ( 'NONE', ( #49136, #38014, #20255, #25765 ) ) ;
#41168=DIRECTION ( 'NONE',  ( 1.000000000000000000, -0.000000000000000000, -0.000000000000000000 ) ) ;
#41171=AXIS2_PLACEMENT_3D ( 'NONE', #48115, #19468, #39190 ) ;
#41174=CARTESIAN_POINT ( 'NONE',  ( -339.1964088526558498, -143.9541802141663709, 55.34326076196097688 ) ) ;
#41175=DIRECTION ( 'NONE',  ( -1.000000000000000000, 0.000000000000000000, 0.000000000000000000 ) ) ;
#41177=CARTESIAN_POINT ( 'NONE',  ( -305.0000000000000568, -143.2422018649890276, 56.65902810251888155 ) ) ;
#41179=VERTEX_POINT ( 'NONE', #24930 ) ;
#41181=PLANE ( 'NONE',  #6635 ) ;
#41186=LINE ( 'NONE', #25940, #40600 ) ;
#41190=DIRECTION ( 'NONE',  ( -0.000000000000000000, -0.7485107481710953081, 0.6631226582408016323 ) ) ;
#41195=ORIENTED_EDGE ( 'NONE', *, *, #14446, .F. ) ;
#41196=FACE_OUTER_BOUND ( 'NONE', #21129, .T. ) ;
#41200=EDGE_LOOP ( 'NONE', ( #19331, #160, #26712, #38058 ) ) ;
#41205=ORIENTED_EDGE ( 'NONE', *, *, #42570, .F. ) ;
#41207=ORIENTED_EDGE ( 'NONE', *, *, #305, .T. ) ;
#41211=PLANE ( 'NONE',  #40619 ) ;
#41213=ORIENTED_EDGE ( 'NONE', *, *, #497, .T. ) ;
#41218=DIRECTION ( 'NONE',  ( -1.000000000000000000, 0.000000000000000000, 0.000000000000000000 ) ) ;
#41219=DIRECTION ( 'NONE',  ( -1.000000000000000000, 0.000000000000000000, 0.000000000000000000 ) ) ;
#41222=ORIENTED_EDGE ( 'NONE', *, *, #14961, .F. ) ;
#41224=DIRECTION ( 'NONE',  ( 1.000000000000000000, 0.000000000000000000, -0.000000000000000000 ) ) ;
#41225=DIRECTION ( 'NONE',  ( 0.000000000000000000, 0.7485107481710934207, -0.6631226582408039638 ) ) ;
#41226=VERTEX_POINT ( 'NONE', #40412 ) ;
#41227=DIRECTION ( 'NONE',  ( 0.000000000000000000, -0.9709418174260534551, -0.2393156642875516327 ) ) ;
#41229=VERTEX_POINT ( 'NONE', #49374 ) ;
#41236=ADVANCED_FACE ( 'NONE', ( #753 ), #32548, .F. ) ;
#41238=AXIS2_PLACEMENT_3D ( 'NONE', #16476, #32496, #37210 ) ;
#41252=EDGE_LOOP ( 'NONE', ( #24599, #27356, #15747, #6212 ) ) ;
#41256=EDGE_CURVE ( 'NONE', #37730, #44450, #29117, .T. ) ;
#41258=CARTESIAN_POINT ( 'NONE',  ( -336.3521761649654422, -148.5878911270064009, 53.46519113769075204 ) ) ;
#41259=ORIENTED_EDGE ( 'NONE', *, *, #42728, .T. ) ;
#41265=CARTESIAN_POINT ( 'NONE',  ( -365.0000000000001137, -168.5000000000000284, 0.000000000000000000 ) ) ;
#41270=CARTESIAN_POINT ( 'NONE',  ( -332.3517673607765914, -105.0395444947681369, -56.09938080879045685 ) ) ;
#41273=DIRECTION ( 'NONE',  ( -1.000000000000000000, 0.000000000000000000, -0.000000000000000000 ) ) ;
#41279=VECTOR ( 'NONE', #12188, 1000.000000000000114 ) ;
#41282=AXIS2_PLACEMENT_3D ( 'NONE', #35285, #28425, #27911 ) ;
#41289=AXIS2_PLACEMENT_3D ( 'NONE', #18176, #49480, #34203 ) ;
#41291=AXIS2_PLACEMENT_3D ( 'NONE', #45445, #12844, #9436 ) ;
#41295=LINE ( 'NONE', #49980, #18643 ) ;
#41304=VERTEX_POINT ( 'NONE', #24402 ) ;
#41308=EDGE_CURVE ( 'NONE', #43501, #29348, #4435, .T. ) ;
#41310=CARTESIAN_POINT ( 'NONE',  ( -339.1964088526558498, -109.6270296344165160, -58.37414404713479854 ) ) ;
#41314=LINE ( 'NONE', #16654, #49562 ) ;
#41319=ORIENTED_EDGE ( 'NONE', *, *, #51631, .T. ) ;
#41321=EDGE_CURVE ( 'NONE', #1001, #15941, #18591, .T. ) ;
#41322=VERTEX_POINT ( 'NONE', #49880 ) ;
#41326=AXIS2_PLACEMENT_3D ( 'NONE', #10216, #17356, #9452 ) ;
#41339=AXIS2_PLACEMENT_3D ( 'NONE', #18376, #7565, #30690 ) ;
#41341=VERTEX_POINT ( 'NONE', #29633 ) ;
#41346=EDGE_LOOP ( 'NONE', ( #22446, #2154, #42274, #1510 ) ) ;
#41349=DIRECTION ( 'NONE',  ( -0.000000000000000000, -0.1205366802553130001, 0.9927088740980551940 ) ) ;
#41350=DIRECTION ( 'NONE',  ( 0.000000000000000000, 0.1205366802553337752, 0.9927088740980526405 ) ) ;
#41351=LINE ( 'NONE', #45328, #1396 ) ;
#41353=ORIENTED_EDGE ( 'NONE', *, *, #11455, .F. ) ;
#41354=LINE ( 'NONE', #549, #12721 ) ;
#41357=ORIENTED_EDGE ( 'NONE', *, *, #10218, .T. ) ;
#41358=DIRECTION ( 'NONE',  ( -1.000000000000000000, 0.000000000000000000, 0.000000000000000000 ) ) ;
#41364=DIRECTION ( 'NONE',  ( -0.000000000000000000, 0.1205366802553337752, 0.9927088740980526405 ) ) ;
#41365=EDGE_CURVE ( 'NONE', #41564, #19062, #9673, .T. ) ;
#41366=VECTOR ( 'NONE', #22626, 1000.000000000000000 ) ;
#41372=DIRECTION ( 'NONE',  ( 0.000000000000000000, -0.1205366802553199113, 0.9927088740980544168 ) ) ;
#41375=DIRECTION ( 'NONE',  ( 0.000000000000000000, 2.775557561562891351E-15, 1.000000000000000000 ) ) ;
#41376=DIRECTION ( 'NONE',  ( 1.000000000000000000, 0.000000000000000000, 0.000000000000000000 ) ) ;
#41377=VECTOR ( 'NONE', #27778, 1000.000000000000000 ) ;
#41380=CARTESIAN_POINT ( 'NONE',  ( -332.3517673607765914, -160.6539403396202772, 45.90766452162722544 ) ) ;
#41382=ORIENTED_EDGE ( 'NONE', *, *, #39729, .F. ) ;
#41383=EDGE_CURVE ( 'NONE', #7384, #1606, #45955, .T. ) ;
#41387=EDGE_CURVE ( 'NONE', #27746, #41391, #41981, .T. ) ;
#41388=LINE ( 'NONE', #49296, #50546 ) ;
#41391=VERTEX_POINT ( 'NONE', #17819 ) ;
#41392=EDGE_CURVE ( 'NONE', #23203, #25253, #5991, .T. ) ;
#41396=ORIENTED_EDGE ( 'NONE', *, *, #23448, .T. ) ;
#41401=DIRECTION ( 'NONE',  ( 0.000000000000000000, 0.000000000000000000, 1.000000000000000000 ) ) ;
#41408=ADVANCED_FACE ( 'NONE', ( #14149 ), #2813, .T. ) ;
#41417=CARTESIAN_POINT ( 'NONE',  ( -336.3521761649654422, -66.84438072661991725, -16.67542351306652648 ) ) ;
#41418=DIRECTION ( 'NONE',  ( 1.000000000000000000, -0.000000000000000000, -0.000000000000000000 ) ) ;
#41427=DIRECTION ( 'NONE',  ( 0.000000000000000000, -0.5680647467311457088, 0.8229838658936633466 ) ) ;
#41431=EDGE_CURVE ( 'NONE', #1552, #4433, #23325, .T. ) ;
#41437=VECTOR ( 'NONE', #11772, 1000.000000000000227 ) ;
#41438=ORIENTED_EDGE ( 'NONE', *, *, #43281, .F. ) ;
#41439=ORIENTED_EDGE ( 'NONE', *, *, #45564, .T. ) ;
#41440=ORIENTED_EDGE ( 'NONE', *, *, #5689, .T. ) ;
#41441=DIRECTION ( 'NONE',  ( 0.000000000000000000, 0.000000000000000000, -1.000000000000000000 ) ) ;
#41449=DIRECTION ( 'NONE',  ( -0.000000000000000000, 0.8854560256532093554, -0.4647231720437695057 ) ) ;
#41452=ORIENTED_EDGE ( 'NONE', *, *, #25963, .T. ) ;
#41461=LINE ( 'NONE', #25701, #51931 ) ;
#41462=ORIENTED_EDGE ( 'NONE', *, *, #6029, .F. ) ;
#41468=LINE ( 'NONE', #33072, #34074 ) ;
#41469=CARTESIAN_POINT ( 'NONE',  ( -330.4913330509368166, -64.86990808808705822, 6.615309698014281814 ) ) ;
#41478=AXIS2_PLACEMENT_3D ( 'NONE', #42694, #22477, #26132 ) ;
#41479=FACE_OUTER_BOUND ( 'NONE', #13732, .T. ) ;
#41485=EDGE_LOOP ( 'NONE', ( #12112, #44441, #8888, #6155 ) ) ;
#41492=LINE ( 'NONE', #8931, #48917 ) ;
#41493=LINE ( 'NONE', #29410, #27025 ) ;
#41494=VECTOR ( 'NONE', #40220, 1000.000000000000000 ) ;
#41497=FACE_OUTER_BOUND ( 'NONE', #38937, .T. ) ;
#41504=EDGE_CURVE ( 'NONE', #14763, #22171, #19881, .T. ) ;
#41505=CARTESIAN_POINT ( 'NONE',  ( -336.3521761649654422, -80.42027357919624819, -40.34602258462219027 ) ) ;
#41506=ORIENTED_EDGE ( 'NONE', *, *, #21099, .T. ) ;
#41510=CARTESIAN_POINT ( 'NONE',  ( -332.3517673607765914, -97.97423230103774472, -54.29949524055093946 ) ) ;
#41511=ORIENTED_EDGE ( 'NONE', *, *, #34958, .T. ) ;
#41512=CARTESIAN_POINT ( 'NONE',  ( -330.4913330509368166, -108.8949048983213004, -57.16590939599337418 ) ) ;
#41513=DIRECTION ( 'NONE',  ( 0.000000000000000000, 0.000000000000000000, 1.000000000000000000 ) ) ;
#41515=CARTESIAN_POINT ( 'NONE',  ( -330.4913330509368166, -167.3305728129748786, -39.49849221029221269 ) ) ;
#41525=CARTESIAN_POINT ( 'NONE',  ( -339.1964088526558498, -175.9742670995615015, -26.97593913775538965 ) ) ;
#41530=CARTESIAN_POINT ( 'NONE',  ( -339.1964088526558498, -123.9999999999993747, 59.00000000000002132 ) ) ;
#41539=EDGE_CURVE ( 'NONE', #8243, #29433, #2807, .T. ) ;
#41542=CARTESIAN_POINT ( 'NONE',  ( -336.3521761649653854, -114.6500883362968892, 59.34373651485599055 ) ) ;
#41543=LINE ( 'NONE', #22363, #16875 ) ;
#41545=VECTOR ( 'NONE', #37176, 999.9999999999998863 ) ;
#41552=EDGE_CURVE ( 'NONE', #24129, #48198, #43274, .T. ) ;
#41556=ORIENTED_EDGE ( 'NONE', *, *, #44039, .F. ) ;
#41558=CARTESIAN_POINT ( 'NONE',  ( -336.3521761649654422, -180.3949349376675855, 15.70448169564087770 ) ) ;
#41561=ORIENTED_EDGE ( 'NONE', *, *, #3184, .T. ) ;
#41564=VERTEX_POINT ( 'NONE', #17243 ) ;
#41565=EDGE_CURVE ( 'NONE', #43598, #20384, #35543, .T. ) ;
#41569=CARTESIAN_POINT ( 'NONE',  ( -330.4913330509368166, -180.6659093959932250, 14.60509510167933556 ) ) ;
#41572=VECTOR ( 'NONE', #12005, 1000.000000000000000 ) ;
#41583=AXIS2_PLACEMENT_3D ( 'NONE', #10124, #34540, #43204 ) ;
#41584=DIRECTION ( 'NONE',  ( -1.000000000000000000, -5.928974370888934796E-15, -8.589602288500814192E-15 ) ) ;
#41587=VERTEX_POINT ( 'NONE', #28780 ) ;
#41588=ORIENTED_EDGE ( 'NONE', *, *, #40971, .F. ) ;
#41590=DIRECTION ( 'NONE',  ( -0.000000000000000000, -0.4647231720437604574, 0.8854560256532141294 ) ) ;
#41592=CARTESIAN_POINT ( 'NONE',  ( -339.1964088526558498, -65.12585595286530804, -13.87297036558381080 ) ) ;
#41597=CARTESIAN_POINT ( 'NONE',  ( -336.3521761649654422, -179.5993808087905279, -18.46045550523168899 ) ) ;
#41599=DIRECTION ( 'NONE',  ( -0.000000000000000000, 0.5680647467311457088, -0.8229838658936633466 ) ) ;
#41603=DIRECTION ( 'NONE',  ( -0.000000000000000000, 0.1205366802553303196, 0.9927088740980530845 ) ) ;
#41608=CARTESIAN_POINT ( 'NONE',  ( -336.3521761649654422, -123.5000000000000284, 0.000000000000000000 ) ) ;
#41610=DIRECTION ( 'NONE',  ( 0.000000000000000000, 0.9350162426854132791, -0.3546048870425396182 ) ) ;
#41611=EDGE_CURVE ( 'NONE', #17341, #29772, #32183, .T. ) ;
#41613=ADVANCED_FACE ( 'NONE', ( #25385 ), #37200, .F. ) ;
#41614=VERTEX_POINT ( 'NONE', #24341 ) ;
#41617=ADVANCED_FACE ( 'NONE', ( #16741 ), #8559, .F. ) ;
#41619=DIRECTION ( 'NONE',  ( -1.000000000000000000, 0.000000000000000000, 0.000000000000000000 ) ) ;
#41620=DIRECTION ( 'NONE',  ( -0.000000000000000000, -0.4647231720437631775, 0.8854560256532126861 ) ) ;
#41627=DIRECTION ( 'NONE',  ( 0.000000000000000000, 0.000000000000000000, -1.000000000000000000 ) ) ;
#41635=ORIENTED_EDGE ( 'NONE', *, *, #44006, .F. ) ;
#41637=CARTESIAN_POINT ( 'NONE',  ( -332.3517673607765914, -123.5000000000000284, 0.000000000000000000 ) ) ;
#41640=AXIS2_PLACEMENT_3D ( 'NONE', #51450, #11483, #7552 ) ;
#41642=CARTESIAN_POINT ( 'NONE',  ( -336.3521761649654422, -160.6539403396202772, 45.90766452162722544 ) ) ;
#41645=AXIS2_PLACEMENT_3D ( 'NONE', #34596, #30396, #50391 ) ;
#41647=LINE ( 'NONE', #45362, #43310 ) ;
#41654=DIRECTION ( 'NONE',  ( 0.000000000000000000, 0.000000000000000000, -1.000000000000000000 ) ) ;
#41656=AXIS2_PLACEMENT_3D ( 'NONE', #4853, #28986, #48988 ) ;
#41660=EDGE_CURVE ( 'NONE', #40560, #34344, #5419, .T. ) ;
#41662=VERTEX_POINT ( 'NONE', #21434 ) ;
#41663=DIRECTION ( 'NONE',  ( 0.000000000000000000, 1.063963731932441632E-14, 1.000000000000000000 ) ) ;
#41671=VECTOR ( 'NONE', #33112, 1000.000000000000000 ) ;
#41679=CARTESIAN_POINT ( 'NONE',  ( 0.000000000000000000, -137.6196241929661710, -57.28556722813703317 ) ) ;
#41683=EDGE_CURVE ( 'NONE', #2972, #21974, #24594, .T. ) ;
#41684=VERTEX_POINT ( 'NONE', #20655 ) ;
#41685=VECTOR ( 'NONE', #43745, 1000.000000000000000 ) ;
#41696=VECTOR ( 'NONE', #40861, 1000.000000000000000 ) ;
#41701=VECTOR ( 'NONE', #46848, 1000.000000000000114 ) ;
#41703=VECTOR ( 'NONE', #38721, 1000.000000000000114 ) ;
#41705=EDGE_CURVE ( 'NONE', #22275, #11192, #14081, .T. ) ;
#41706=VERTEX_POINT ( 'NONE', #30097 ) ;
#41707=ORIENTED_EDGE ( 'NONE', *, *, #6342, .T. ) ;
#41708=ORIENTED_EDGE ( 'NONE', *, *, #14572, .T. ) ;
#41709=AXIS2_PLACEMENT_3D ( 'NONE', #12629, #23941, #20516 ) ;
#41717=ADVANCED_FACE ( 'NONE', ( #37976 ), #50341, .F. ) ;
#41719=EDGE_LOOP ( 'NONE', ( #23141, #37347, #8757, #24851 ) ) ;
#41723=EDGE_LOOP ( 'NONE', ( #41319, #28373, #29597, #21134 ) ) ;
#41726=FACE_OUTER_BOUND ( 'NONE', #13278, .T. ) ;
#41731=DIRECTION ( 'NONE',  ( -0.000000000000000000, 0.5680647467311540355, -0.8229838658936575735 ) ) ;
#41732=EDGE_CURVE ( 'NONE', #21321, #46459, #48894, .T. ) ;
#41736=CARTESIAN_POINT ( 'NONE',  ( -330.4913330509368166, -75.22798428563942252, 33.92731199008440512 ) ) ;
#41737=ORIENTED_EDGE ( 'NONE', *, *, #19255, .F. ) ;
#41738=ADVANCED_FACE ( 'NONE', ( #17763 ), #26143, .F. ) ;
#41739=ORIENTED_EDGE ( 'NONE', *, *, #33427, .T. ) ;
#41744=EDGE_CURVE ( 'NONE', #26309, #44752, #46398, .T. ) ;
#41745=CARTESIAN_POINT ( 'NONE',  ( -332.3517673607765914, -176.5004679656469477, -25.97334715265976612 ) ) ;
#41747=ORIENTED_EDGE ( 'NONE', *, *, #46257, .F. ) ;
#41752=PLANE ( 'NONE',  #27033 ) ;
#41756=DIRECTION ( 'NONE',  ( -0.000000000000000000, -0.5680647467311596976, -0.8229838658936536877 ) ) ;
#41763=CARTESIAN_POINT ( 'NONE',  ( -305.0000000000000568, -123.5000000000000284, -60.00000000000000000 ) ) ;
#41768=ORIENTED_EDGE ( 'NONE', *, *, #24000, .T. ) ;
#41770=AXIS2_PLACEMENT_3D ( 'NONE', #50019, #17453, #28977 ) ;
#41773=LINE ( 'NONE', #45715, #29541 ) ;
#41774=LINE ( 'NONE', #29155, #3553 ) ;
#41775=CIRCLE ( 'NONE', #14059, 60.00000000000000000 ) ;
#41776=CARTESIAN_POINT ( 'NONE',  ( -336.3521761649653854, -117.8908635894569272, -59.73723787327232060 ) ) ;
#41790=CARTESIAN_POINT ( 'NONE',  ( -339.1964088526558498, -79.66942718702553350, -39.49849221029258928 ) ) ;
#41791=VERTEX_POINT ( 'NONE', #18284 ) ;
#41802=CARTESIAN_POINT ( 'NONE',  ( -339.1964088526558498, -71.49045607248255862, -27.86139516340906397 ) ) ;
#41806=VECTOR ( 'NONE', #25318, 1000.000000000000000 ) ;
#41808=AXIS2_PLACEMENT_3D ( 'NONE', #13881, #18351, #1535 ) ;
#41816=ORIENTED_EDGE ( 'NONE', *, *, #27237, .T. ) ;
#41820=ORIENTED_EDGE ( 'NONE', *, *, #3739, .F. ) ;
#41826=LINE ( 'NONE', #1871, #29989 ) ;
#41827=ADVANCED_FACE ( 'NONE', ( #17519 ), #38505, .F. ) ;
#41828=DIRECTION ( 'NONE',  ( -8.718379230999705894E-17, 0.7485107481710977506, -0.6631226582407989678 ) ) ;
#41831=FACE_OUTER_BOUND ( 'NONE', #24308, .T. ) ;
#41834=ORIENTED_EDGE ( 'NONE', *, *, #4013, .F. ) ;
#41835=CARTESIAN_POINT ( 'NONE',  ( -305.0000000000000568, -70.14212160686594189, 27.43969411971487560 ) ) ;
#41837=CARTESIAN_POINT ( 'NONE',  ( -339.1964088526558498, -138.1050951016792681, -57.16590939599323917 ) ) ;
#41838=ORIENTED_EDGE ( 'NONE', *, *, #23168, .F. ) ;
#41845=AXIS2_PLACEMENT_3D ( 'NONE', #20500, #521, #36021 ) ;
#41851=DIRECTION ( 'NONE',  ( -0.000000000000000000, 0.000000000000000000, -1.000000000000000000 ) ) ;
#41854=ORIENTED_EDGE ( 'NONE', *, *, #30859, .F. ) ;
#41868=ADVANCED_FACE ( 'NONE', ( #22990 ), #7735, .F. ) ;
#41869=ORIENTED_EDGE ( 'NONE', *, *, #50762, .F. ) ;
#41871=PLANE ( 'NONE',  #18057 ) ;
#41872=EDGE_LOOP ( 'NONE', ( #25668, #3421, #44784, #46750 ) ) ;
#41873=CARTESIAN_POINT ( 'NONE',  ( -330.4913330509368166, -74.65991953890832633, 33.10432812419081472 ) ) ;
#41875=FACE_OUTER_BOUND ( 'NONE', #22424, .T. ) ;
#41877=CARTESIAN_POINT ( 'NONE',  ( -339.1964088526558498, -96.52406086224443982, -52.47426709956138069 ) ) ;
#41878=DIRECTION ( 'NONE',  ( -0.000000000000000000, 0.7485107481711089639, 0.6631226582407863113 ) ) ;
#41879=EDGE_CURVE ( 'NONE', #46318, #34791, #11676, .T. ) ;
#41880=VERTEX_POINT ( 'NONE', #11404 ) ;
#41881=AXIS2_PLACEMENT_3D ( 'NONE', #22838, #38857, #17868 ) ;
#41883=CARTESIAN_POINT ( 'NONE',  ( -330.4913330509368166, -130.1153096980145563, 58.63009191191294178 ) ) ;
#41884=CARTESIAN_POINT ( 'NONE',  ( -336.3521761649654422, -133.2247606357419443, -58.25253621232173629 ) ) ;
#41885=CARTESIAN_POINT ( 'NONE',  ( -336.3521761649654422, -123.5000000000000284, 0.000000000000000000 ) ) ;
#41887=DIRECTION ( 'NONE',  ( 0.000000000000000000, -0.2393156642875615969, -0.9709418174260511236 ) ) ;
#41889=CIRCLE ( 'NONE', #48620, 60.00000000000000000 ) ;
#41894=AXIS2_PLACEMENT_3D ( 'NONE', #35578, #15631, #31645 ) ;
#41896=VERTEX_POINT ( 'NONE', #3283 ) ;
#41900=DIRECTION ( 'NONE',  ( 1.000000000000000000, 0.000000000000000000, -0.000000000000000000 ) ) ;
#41901=ADVANCED_FACE ( 'NONE', ( #23763 ), #35327, .F. ) ;
#41904=ORIENTED_EDGE ( 'NONE', *, *, #1886, .F. ) ;
#41913=ORIENTED_EDGE ( 'NONE', *, *, #33062, .F. ) ;
#41915=ADVANCED_FACE ( 'NONE', ( #15628 ), #31902, .F. ) ;
#41919=ORIENTED_EDGE ( 'NONE', *, *, #42936, .T. ) ;
#41924=DIRECTION ( 'NONE',  ( -1.000000000000000000, -0.000000000000000000, -0.000000000000000000 ) ) ;
#41932=CARTESIAN_POINT ( 'NONE',  ( -339.1964088526558498, -71.49045607248213230, 27.86139516340826106 ) ) ;
#41934=VERTEX_POINT ( 'NONE', #23262 ) ;
#41945=VERTEX_POINT ( 'NONE', #31644 ) ;
#41948=PRODUCT ( 'Center Pivot Base Stud', 'Center Pivot Base Stud', '', ( #17333 ) ) ;
#41949=DIRECTION ( 'NONE',  ( 0.000000000000000000, -6.036837696399288689E-14, 1.000000000000000000 ) ) ;
#41952=EDGE_LOOP ( 'NONE', ( #47983, #22667, #28845, #25777 ) ) ;
#41954=EDGE_CURVE ( 'NONE', #41304, #29838, #31128, .T. ) ;
#41960=ORIENTED_EDGE ( 'NONE', *, *, #49052, .F. ) ;
#41963=CARTESIAN_POINT ( 'NONE',  ( 0.000000000000000000, -172.0560480877259408, -33.51582005713793677 ) ) ;
#41964=LINE ( 'NONE', #5979, #15273 ) ;
#41972=EDGE_LOOP ( 'NONE', ( #855, #38784, #24114, #21024 ) ) ;
#41973=VERTEX_POINT ( 'NONE', #43485 ) ;
#41974=ADVANCED_FACE ( 'NONE', ( #39276 ), #7489, .F. ) ;
#41976=ORIENTED_EDGE ( 'NONE', *, *, #29495, .F. ) ;
#41979=ORIENTED_EDGE ( 'NONE', *, *, #38805, .T. ) ;
#41980=EDGE_CURVE ( 'NONE', #30123, #49231, #20868, .T. ) ;
#41981=LINE ( 'NONE', #9940, #18758 ) ;
#41989=LINE ( 'NONE', #9953, #24474 ) ;
#41994=DIRECTION ( 'NONE',  ( -1.000000000000000000, 0.000000000000000000, 0.000000000000000000 ) ) ;
#41995=DIRECTION ( 'NONE',  ( -0.000000000000000000, -0.9709418174260534551, -0.2393156642875516327 ) ) ;
#41998=DIRECTION ( 'NONE',  ( 1.000000000000000000, 0.000000000000000000, 0.000000000000000000 ) ) ;
#42001=CARTESIAN_POINT ( 'NONE',  ( -305.0000000000000568, -83.33976666098978114, 44.57752413667957825 ) ) ;
#42005=LINE ( 'NONE', #41763, #24410 ) ;
#42007=VERTEX_POINT ( 'NONE', #353 ) ;
#42011=DIRECTION ( 'NONE',  ( 1.000000000000000000, -0.000000000000000000, -0.000000000000000000 ) ) ;
#42013=LINE ( 'NONE', #6027, #37948 ) ;
#42016=EDGE_CURVE ( 'NONE', #2925, #37502, #32159, .T. ) ;
#42018=DIRECTION ( 'NONE',  ( -0.000000000000000000, 0.000000000000000000, 1.000000000000000000 ) ) ;
#42025=CARTESIAN_POINT ( 'NONE',  ( -305.0000000000000568, -115.7716958700749643, 59.50019592636132160 ) ) ;
#42027=EDGE_CURVE ( 'NONE', #41587, #12564, #2730, .T. ) ;
#42029=VECTOR ( 'NONE', #50491, 1000.000000000000114 ) ;
#42034=CARTESIAN_POINT ( 'NONE',  ( -332.3517673607765914, -174.5186198893880771, 29.74944317415823392 ) ) ;
#42035=VERTEX_POINT ( 'NONE', #36625 ) ;
#42037=DIRECTION ( 'NONE',  ( -8.718379230999707126E-17, 0.5680647467311510379, -0.8229838658936596829 ) ) ;
#42042=PLANE ( 'NONE',  #11289 ) ;
#42046=LINE ( 'NONE', #33125, #38368 ) ;
#42049=EDGE_LOOP ( 'NONE', ( #26182, #6932, #46524, #9338 ) ) ;
#42055=CIRCLE ( 'NONE', #8469, 60.00000000000000000 ) ;
#42058=DIRECTION ( 'NONE',  ( 0.000000000000000000, 0.000000000000000000, 1.000000000000000000 ) ) ;
#42059=CARTESIAN_POINT ( 'NONE',  ( -330.4913330509368166, -123.5000000000000284, 0.000000000000000000 ) ) ;
#42060=CARTESIAN_POINT ( 'NONE',  ( -330.4913330509368166, -182.1300919119128423, 6.615309698015510165 ) ) ;
#42061=DIRECTION ( 'NONE',  ( 0.000000000000000000, -0.8229838658936556861, 0.5680647467311569221 ) ) ;
#42062=ORIENTED_EDGE ( 'NONE', *, *, #3115, .T. ) ;
#42073=DIRECTION ( 'NONE',  ( 1.000000000000000000, -0.000000000000000000, 0.000000000000000000 ) ) ;
#42079=VERTEX_POINT ( 'NONE', #8760 ) ;
#42087=FACE_OUTER_BOUND ( 'NONE', #17360, .T. ) ;
#42088=ORIENTED_EDGE ( 'NONE', *, *, #16677, .T. ) ;
#42090=CIRCLE ( 'NONE', #13546, 60.00000000000000000 ) ;
#42092=LINE ( 'NONE', #51042, #10785 ) ;
#42093=DIRECTION ( 'NONE',  ( -0.000000000000000000, -0.9709418174260502354, 0.2393156642875652051 ) ) ;
#42096=CARTESIAN_POINT ( 'NONE',  ( -305.0000000000000568, -172.5932850007656043, 34.49419324804693332 ) ) ;
#42098=LINE ( 'NONE', #18200, #5679 ) ;
#42104=ORIENTED_EDGE ( 'NONE', *, *, #33748, .F. ) ;
#42108=CARTESIAN_POINT ( 'NONE',  ( -336.3521761649654422, -64.50000000000000000, -1.632288850093980725 ) ) ;
#42114=ORIENTED_EDGE ( 'NONE', *, *, #21504, .F. ) ;
#42116=VERTEX_POINT ( 'NONE', #10019 ) ;
#42117=FACE_BOUND ( 'NONE', #28743, .T. ) ;
#42119=CARTESIAN_POINT ( 'NONE',  ( -336.3521761649654422, -153.2494431741581025, -51.01861988938816950 ) ) ;
#42120=ORIENTED_EDGE ( 'NONE', *, *, #36557, .F. ) ;
#42122=ORIENTED_EDGE ( 'NONE', *, *, #8262, .T. ) ;
#42124=VECTOR ( 'NONE', #35234, 1000.000000000000000 ) ;
#42127=ORIENTED_EDGE ( 'NONE', *, *, #21305, .F. ) ;
#42131=ORIENTED_EDGE ( 'NONE', *, *, #9575, .T. ) ;
#42132=CARTESIAN_POINT ( 'NONE',  ( -330.4913330509368166, -180.9052250602809693, -13.63415328425256945 ) ) ;
#42134=DIRECTION ( 'NONE',  ( -0.000000000000000000, 0.000000000000000000, 1.000000000000000000 ) ) ;
#42140=EDGE_CURVE ( 'NONE', #34344, #12665, #30238, .T. ) ;
#42144=ORIENTED_EDGE ( 'NONE', *, *, #10318, .T. ) ;
#42145=CARTESIAN_POINT ( 'NONE',  ( 0.000000000000000000, -167.6621341420946578, 39.12423683620730230 ) ) ;
#42148=CARTESIAN_POINT ( 'NONE',  ( -332.3517673607765914, -72.01665693856799066, -28.86398714850468039 ) ) ;
#42150=LINE ( 'NONE', #18765, #10651 ) ;
#42151=ORIENTED_EDGE ( 'NONE', *, *, #31598, .T. ) ;
#42154=AXIS2_PLACEMENT_3D ( 'NONE', #22209, #14333, #34544 ) ;
#42157=LINE ( 'NONE', #10627, #2543 ) ;
#42159=AXIS2_PLACEMENT_3D ( 'NONE', #24268, #20310, #15878 ) ;
#42160=EDGE_CURVE ( 'NONE', #38437, #12857, #14474, .T. ) ;
#42166=CARTESIAN_POINT ( 'NONE',  ( -332.3517673607765914, -123.5000000000000284, 0.000000000000000000 ) ) ;
#42170=VECTOR ( 'NONE', #3655, 1000.000000000000000 ) ;
#42172=CARTESIAN_POINT ( 'NONE',  ( -330.4913330509368166, -123.5000000000000284, 0.000000000000000000 ) ) ;
#42173=VERTEX_POINT ( 'NONE', #2386 ) ;
#42175=EDGE_CURVE ( 'NONE', #32017, #32388, #10507, .T. ) ;
#42180=ADVANCED_FACE ( 'NONE', ( #38628 ), #27049, .F. ) ;
#42189=CARTESIAN_POINT ( 'NONE',  ( -339.1964088526558498, -175.5095439275173135, 27.86139516340941213 ) ) ;
#42190=ORIENTED_EDGE ( 'NONE', *, *, #4709, .F. ) ;
#42191=AXIS2_PLACEMENT_3D ( 'NONE', #27465, #35347, #43232 ) ;
#42194=EDGE_LOOP ( 'NONE', ( #38109, #35204, #30833, #50148 ) ) ;
#42203=CARTESIAN_POINT ( 'NONE',  ( -336.3521761649654422, -119.0014323656137947, -58.88711093124865670 ) ) ;
#42206=LINE ( 'NONE', #46178, #31676 ) ;
#42210=EDGE_LOOP ( 'NONE', ( #28723, #15911, #34307, #35354 ) ) ;
#42214=DIRECTION ( 'NONE',  ( -0.000000000000000000, 0.1205366802553199113, -0.9927088740980544168 ) ) ;
#42217=LINE ( 'NONE', #35898, #43564 ) ;
#42219=CARTESIAN_POINT ( 'NONE',  ( -339.1964088526558498, -131.1080185721133660, -58.50955523165751515 ) ) ;
#42222=VECTOR ( 'NONE', #3043, 1000.000000000000000 ) ;
#42232=EDGE_LOOP ( 'NONE', ( #37137, #26147, #17100, #30794 ) ) ;
#42237=ORIENTED_EDGE ( 'NONE', *, *, #35945, .F. ) ;
#42240=LINE ( 'NONE', #22280, #49081 ) ;
#42252=ORIENTED_EDGE ( 'NONE', *, *, #31391, .T. ) ;
#42256=CARTESIAN_POINT ( 'NONE',  ( -332.3517673607765914, -163.8460225846223466, -43.07972642080364523 ) ) ;
#42259=CARTESIAN_POINT ( 'NONE',  ( -180.0000000000000568, -123.5000000000000284, 0.000000000000000000 ) ) ;
#42265=ADVANCED_FACE ( 'NONE', ( #28348 ), #39393, .F. ) ;
#42266=DIRECTION ( 'NONE',  ( 0.000000000000000000, 0.7485107481711000821, -0.6631226582407965253 ) ) ;
#42270=LINE ( 'NONE', #22304, #22920 ) ;
#42273=DIRECTION ( 'NONE',  ( -1.000000000000000000, 0.000000000000000000, 0.000000000000000000 ) ) ;
#42274=ORIENTED_EDGE ( 'NONE', *, *, #10464, .F. ) ;
#42275=FACE_OUTER_BOUND ( 'NONE', #1332, .T. ) ;
#42288=DIRECTION ( 'NONE',  ( -0.000000000000000000, -0.5680647467311510379, 0.8229838658936596829 ) ) ;
#42296=VECTOR ( 'NONE', #49359, 999.9999999999998863 ) ;
#42300=CARTESIAN_POINT ( 'NONE',  ( -305.0000000000000568, -173.1613497474965300, 33.67120938215357739 ) ) ;
#42301=DIRECTION ( 'NONE',  ( -8.718379230999707126E-17, -1.000000000000000000, 1.047444401652940007E-14 ) ) ;
#42303=EDGE_CURVE ( 'NONE', #51141, #11736, #23388, .T. ) ;
#42305=FACE_OUTER_BOUND ( 'NONE', #23429, .T. ) ;
#42318=VERTEX_POINT ( 'NONE', #40426 ) ;
#42320=ADVANCED_FACE ( 'NONE', ( #31254 ), #12048, .F. ) ;
#42326=CARTESIAN_POINT ( 'NONE',  ( -332.3517673607765914, -183.4777928329299357, 1.632288850093980725 ) ) ;
#42330=EDGE_CURVE ( 'NONE', #42476, #47980, #16023, .T. ) ;
#42331=FACE_OUTER_BOUND ( 'NONE', #39514, .T. ) ;
#42332=EDGE_CURVE ( 'NONE', #24982, #23338, #24169, .T. ) ;
#42333=CARTESIAN_POINT ( 'NONE',  ( -336.3521761649654422, -183.4422309845877805, 2.632288850093980503 ) ) ;
#42335=CARTESIAN_POINT ( 'NONE',  ( -305.0000000000000568, -64.66963335249506883, 11.78931550685348206 ) ) ;
#42337=ORIENTED_EDGE ( 'NONE', *, *, #39008, .T. ) ;
#42349=VERTEX_POINT ( 'NONE', #43358 ) ;
#42350=EDGE_CURVE ( 'NONE', #12857, #4717, #27579, .T. ) ;
#42354=CARTESIAN_POINT ( 'NONE',  ( -336.3521761649654422, -153.2494431741581025, -51.01861988938816950 ) ) ;
#42356=DIRECTION ( 'NONE',  ( -1.000000000000000000, -1.043714542225393381E-14, 3.644109847259164491E-29 ) ) ;
#42358=EDGE_LOOP ( 'NONE', ( #18766, #36134, #39406, #25782 ) ) ;
#42366=EDGE_CURVE ( 'NONE', #44602, #50728, #20997, .T. ) ;
#42367=VERTEX_POINT ( 'NONE', #45694 ) ;
#42372=DIRECTION ( 'NONE',  ( -0.000000000000000000, 0.9709418174260553425, 0.2393156642875449158 ) ) ;
#42375=ADVANCED_FACE ( 'NONE', ( #9176 ), #41211, .F. ) ;
#42377=VERTEX_POINT ( 'NONE', #21256 ) ;
#42378=EDGE_CURVE ( 'NONE', #36303, #49241, #37789, .T. ) ;
#42379=FACE_BOUND ( 'NONE', #30629, .T. ) ;
#42381=DIRECTION ( 'NONE',  ( -8.718379230999708359E-17, -0.4647231720437573488, 0.8854560256532157947 ) ) ;
#42384=CARTESIAN_POINT ( 'NONE',  ( -330.4913330509368166, -156.6043281241909995, 48.84008046109159551 ) ) ;
#42385=EDGE_LOOP ( 'NONE', ( #24290, #48964, #16745, #21258 ) ) ;
#42392=ORIENTED_EDGE ( 'NONE', *, *, #42813, .T. ) ;
#42393=DIRECTION ( 'NONE',  ( -0.000000000000000000, 0.3546048870425331789, -0.9350162426854158326 ) ) ;
#42394=ORIENTED_EDGE ( 'NONE', *, *, #45012, .T. ) ;
#42398=CARTESIAN_POINT ( 'NONE',  ( -332.3517673607765914, -123.5000000000000284, 0.000000000000000000 ) ) ;
#42403=EDGE_CURVE ( 'NONE', #20203, #10838, #17584, .T. ) ;
#42408=FACE_OUTER_BOUND ( 'NONE', #38861, .T. ) ;
#42411=AXIS2_PLACEMENT_3D ( 'NONE', #29567, #13013, #13543 ) ;
#42412=ORIENTED_EDGE ( 'NONE', *, *, #29821, .T. ) ;
#42414=LINE ( 'NONE', #46372, #26688 ) ;
#42415=CIRCLE ( 'NONE', #50833, 60.00000000000000000 ) ;
#42418=LINE ( 'NONE', #2484, #36644 ) ;
#42423=DIRECTION ( 'NONE',  ( 1.000000000000000000, -0.000000000000000000, -0.000000000000000000 ) ) ;
#42429=ORIENTED_EDGE ( 'NONE', *, *, #26005, .T. ) ;
#42439=EDGE_CURVE ( 'NONE', #40265, #47080, #12838, .T. ) ;
#42442=ORIENTED_EDGE ( 'NONE', *, *, #13814, .F. ) ;
#42444=AXIS2_PLACEMENT_3D ( 'NONE', #41265, #13170, #29187 ) ;
#42450=DIRECTION ( 'NONE',  ( 0.000000000000000000, 0.000000000000000000, 1.000000000000000000 ) ) ;
#42452=CARTESIAN_POINT ( 'NONE',  ( -336.3521761649654422, -66.60506506233235768, -15.70448169564047092 ) ) ;
#42454=AXIS2_PLACEMENT_3D ( 'NONE', #3294, #39533, #30610 ) ;
#42455=VERTEX_POINT ( 'NONE', #36768 ) ;
#42456=EDGE_CURVE ( 'NONE', #18178, #20840, #13787, .T. ) ;
#42460=CARTESIAN_POINT ( 'NONE',  ( -339.1964088526558498, -180.6659093959934523, -14.60509510167853264 ) ) ;
#42461=VERTEX_POINT ( 'NONE', #37277 ) ;
#42463=PLANE ( 'NONE',  #36052 ) ;
#42468=LINE ( 'NONE', #11184, #44751 ) ;
#42469=EDGE_LOOP ( 'NONE', ( #26979, #51114, #25887, #45155 ) ) ;
#42474=CARTESIAN_POINT ( 'NONE',  ( -336.3521761649654422, -75.87119766449505676, -34.85916744524372746 ) ) ;
#42476=VERTEX_POINT ( 'NONE', #25710 ) ;
#42477=VERTEX_POINT ( 'NONE', #41745 ) ;
#42478=CARTESIAN_POINT ( 'NONE',  ( -330.4913330509368166, -144.8891964568517778, 54.98865587491845730 ) ) ;
#42480=VECTOR ( 'NONE', #41364, 1000.000000000000114 ) ;
#42481=LINE ( 'NONE', #26187, #38539 ) ;
#42483=DIRECTION ( 'NONE',  ( 1.000000000000000000, -0.000000000000000000, -0.000000000000000000 ) ) ;
#42487=VECTOR ( 'NONE', #21313, 1000.000000000000000 ) ;
#42491=ORIENTED_EDGE ( 'NONE', *, *, #3175, .T. ) ;
#42493=ORIENTED_EDGE ( 'NONE', *, *, #14961, .T. ) ;
#42494=ORIENTED_EDGE ( 'NONE', *, *, #42027, .F. ) ;
#42505=DIRECTION ( 'NONE',  ( -0.000000000000000000, 0.5680647467311569221, 0.8229838658936556861 ) ) ;
#42506=ADVANCED_FACE ( 'NONE', ( #1541 ), #44911, .T. ) ;
#42514=VECTOR ( 'NONE', #6511, 1000.000000000000000 ) ;
#42517=VERTEX_POINT ( 'NONE', #4979 ) ;
#42520=DIRECTION ( 'NONE',  ( 1.000000000000000000, 0.000000000000000000, -0.000000000000000000 ) ) ;
#42523=VECTOR ( 'NONE', #39260, 1000.000000000000000 ) ;
#42530=CIRCLE ( 'NONE', #27402, 60.00000000000000000 ) ;
#42531=ORIENTED_EDGE ( 'NONE', *, *, #6062, .F. ) ;
#42532=VECTOR ( 'NONE', #21639, 1000.000000000000227 ) ;
#42534=CARTESIAN_POINT ( 'NONE',  ( -336.3521761649654422, -76.43926241122620979, -35.68215131113738181 ) ) ;
#42536=DIRECTION ( 'NONE',  ( 0.000000000000000000, -1.000000000000000000, 3.491481338843133355E-15 ) ) ;
#42538=ORIENTED_EDGE ( 'NONE', *, *, #50762, .T. ) ;
#42539=CARTESIAN_POINT ( 'NONE',  ( -332.3517673607765914, -123.5000000000000284, 0.000000000000000000 ) ) ;
#42563=CONICAL_SURFACE ( 'NONE', #35031, 20.00000000000000355, 0.4363323129985833826 ) ;
#42564=CARTESIAN_POINT ( 'NONE',  ( -339.1964088526558498, -175.9742670995610752, 26.97593913775620678 ) ) ;
#42568=VERTEX_POINT ( 'NONE', #43028 ) ;
#42570=EDGE_CURVE ( 'NONE', #13751, #3383, #1789, .T. ) ;
#42573=ORIENTED_EDGE ( 'NONE', *, *, #14812, .F. ) ;
#42574=DIRECTION ( 'NONE',  ( -1.000000000000000000, 0.000000000000000000, 0.000000000000000000 ) ) ;
#42577=EDGE_CURVE ( 'NONE', #37376, #19422, #41989, .T. ) ;
#42579=DIRECTION ( 'NONE',  ( 0.000000000000000000, -0.6631226582407863113, 0.7485107481711089639 ) ) ;
#42585=DIRECTION ( 'NONE',  ( -1.000000000000000000, 0.000000000000000000, 0.000000000000000000 ) ) ;
#42586=DIRECTION ( 'NONE',  ( 0.000000000000000000, 0.000000000000000000, 1.000000000000000000 ) ) ;
#42587=CARTESIAN_POINT ( 'NONE',  ( -339.1964088526558498, -84.00150778970699150, 43.83057281297409702 ) ) ;
#42588=VERTEX_POINT ( 'NONE', #14158 ) ;
#42590=VECTOR ( 'NONE', #14987, 1000.000000000000000 ) ;
#42591=DIRECTION ( 'NONE',  ( -0.000000000000000000, -0.1205366802553130001, 0.9927088740980551940 ) ) ;
#42592=FACE_OUTER_BOUND ( 'NONE', #37662, .T. ) ;
#42596=ORIENTED_EDGE ( 'NONE', *, *, #1912, .T. ) ;
#42602=AXIS2_PLACEMENT_3D ( 'NONE', #13874, #49875, #5988 ) ;
#42604=AXIS2_PLACEMENT_3D ( 'NONE', #21588, #26801, #14998 ) ;
#42610=ORIENTED_EDGE ( 'NONE', *, *, #14125, .F. ) ;
#42611=DIRECTION ( 'NONE',  ( 0.000000000000000000, 0.1205366802553233113, 0.9927088740980538617 ) ) ;
#42619=PLANE ( 'NONE',  #40293 ) ;
#42624=CIRCLE ( 'NONE', #19968, 60.00000000000000000 ) ;
#42625=EDGE_CURVE ( 'NONE', #4472, #37318, #48272, .T. ) ;
#42627=ORIENTED_EDGE ( 'NONE', *, *, #40096, .F. ) ;
#42632=EDGE_CURVE ( 'NONE', #30980, #7704, #51198, .T. ) ;
#42643=CARTESIAN_POINT ( 'NONE',  ( -330.4913330509368166, -143.9541802141664562, 55.34326076196094135 ) ) ;
#42646=FACE_BOUND ( 'NONE', #3740, .T. ) ;
#42647=CARTESIAN_POINT ( 'NONE',  ( -305.0000000000000568, -70.14212160686619768, -27.43969411971536942 ) ) ;
#42648=VECTOR ( 'NONE', #7838, 1000.000000000000000 ) ;
#42653=LINE ( 'NONE', #9558, #40324 ) ;
#42654=VERTEX_POINT ( 'NONE', #3084 ) ;
#42663=AXIS2_PLACEMENT_3D ( 'NONE', #45731, #40727, #13151 ) ;
#42667=ORIENTED_EDGE ( 'NONE', *, *, #38702, .F. ) ;
#42669=VERTEX_POINT ( 'NONE', #28536 ) ;
#42671=EDGE_CURVE ( 'NONE', #4717, #42476, #10222, .T. ) ;
#42672=DIRECTION ( 'NONE',  ( -8.718379230999705894E-17, -0.7485107481711069655, -0.6631226582407885317 ) ) ;
#42674=ORIENTED_EDGE ( 'NONE', *, *, #5373, .F. ) ;
#42677=CARTESIAN_POINT ( 'NONE',  ( -305.0000000000000568, -183.4422309845877805, 2.632288850093980503 ) ) ;
#42678=DIRECTION ( 'NONE',  ( -0.000000000000000000, -0.9350162426854169428, -0.3546048870425300148 ) ) ;
#42682=EDGE_CURVE ( 'NONE', #42318, #46650, #8571, .T. ) ;
#42683=DIRECTION ( 'NONE',  ( -0.000000000000000000, 0.2393156642875547968, -0.9709418174260527890 ) ) ;
#42688=ORIENTED_EDGE ( 'NONE', *, *, #49078, .F. ) ;
#42692=EDGE_CURVE ( 'NONE', #7764, #23663, #24604, .T. ) ;
#42694=CARTESIAN_POINT ( 'NONE',  ( -336.3521761649654422, -123.5000000000000284, 0.000000000000000000 ) ) ;
#42697=EDGE_CURVE ( 'NONE', #21438, #34375, #4377, .T. ) ;
#42700=ADVANCED_FACE ( 'NONE', ( #4636 ), #13033, .F. ) ;
#42701=ORIENTED_EDGE ( 'NONE', *, *, #4078, .T. ) ;
#42705=DIRECTION ( 'NONE',  ( 0.000000000000000000, 0.9927088740980534176, -0.1205366802553268502 ) ) ;
#42710=VECTOR ( 'NONE', #11252, 1000.000000000000114 ) ;
#42712=CARTESIAN_POINT ( 'NONE',  ( -336.3521761649654422, -168.7445418633863596, -37.90245108779149064 ) ) ;
#42715=DIRECTION ( 'NONE',  ( -0.000000000000000000, -0.3546048870425267951, 0.9350162426854181641 ) ) ;
#42717=ORIENTED_EDGE ( 'NONE', *, *, #18153, .F. ) ;
#42718=CARTESIAN_POINT ( 'NONE',  ( -332.3517673607765914, -181.8730728925770563, 8.732051761644092025 ) ) ;
#42725=PLANE ( 'NONE',  #45864 ) ;
#42728=EDGE_CURVE ( 'NONE', #49241, #27624, #44842, .T. ) ;
#42729=DIRECTION ( 'NONE',  ( 0.000000000000000000, 0.2393156642875685636, 0.9709418174260492362 ) ) ;
#42731=PLANE ( 'NONE',  #17752 ) ;
#42735=ORIENTED_EDGE ( 'NONE', *, *, #2145, .T. ) ;
#42736=CARTESIAN_POINT ( 'NONE',  ( -339.1964088526558498, -71.02573290043838483, 26.97593913775504504 ) ) ;
#42745=EDGE_CURVE ( 'NONE', #40405, #13290, #20940, .T. ) ;
#42752=CARTESIAN_POINT ( 'NONE',  ( -339.1964088526558498, -123.5000000000000284, 0.000000000000000000 ) ) ;
#42754=DIRECTION ( 'NONE',  ( 0.000000000000000000, -0.8854560256532141294, -0.4647231720437604574 ) ) ;
#42755=DIRECTION ( 'NONE',  ( -0.000000000000000000, 0.9927088740980556381, 0.1205366802553095307 ) ) ;
#42770=DIRECTION ( 'NONE',  ( 0.000000000000000000, 0.8854560256532126861, 0.4647231720437631775 ) ) ;
#42771=EDGE_LOOP ( 'NONE', ( #37439, #46421, #31398, #21895 ) ) ;
#42773=ORIENTED_EDGE ( 'NONE', *, *, #36602, .T. ) ;
#42777=PLANE ( 'NONE',  #19013 ) ;
#42781=DIRECTION ( 'NONE',  ( -1.000000000000000000, 0.000000000000000000, 0.000000000000000000 ) ) ;
#42782=DIRECTION ( 'NONE',  ( 0.000000000000000000, 0.3546048870425463906, 0.9350162426854107256 ) ) ;
#42783=ORIENTED_EDGE ( 'NONE', *, *, #51349, .F. ) ;
#42785=CARTESIAN_POINT ( 'NONE',  ( -330.4913330509368166, -79.00630452878421295, 38.74998146212088557 ) ) ;
#42786=LINE ( 'NONE', #34880, #23220 ) ;
#42791=VERTEX_POINT ( 'NONE', #22740 ) ;
#42793=VECTOR ( 'NONE', #36652, 1000.000000000000000 ) ;
#42796=CARTESIAN_POINT ( 'NONE',  ( -336.3521761649654422, -164.5945333327934463, -42.41660376256285048 ) ) ;
#42805=ORIENTED_EDGE ( 'NONE', *, *, #4115, .T. ) ;
#42813=EDGE_CURVE ( 'NONE', #33858, #17577, #25908, .T. ) ;
#42815=ORIENTED_EDGE ( 'NONE', *, *, #9475, .F. ) ;
#42817=ORIENTED_EDGE ( 'NONE', *, *, #38818, .F. ) ;
#42818=DIRECTION ( 'NONE',  ( -0.000000000000000000, 0.6631226582408039638, 0.7485107481710934207 ) ) ;
#42819=EDGE_LOOP ( 'NONE', ( #42088, #48267, #36014, #51035 ) ) ;
#42824=VECTOR ( 'NONE', #28961, 1000.000000000000000 ) ;
#42827=CARTESIAN_POINT ( 'NONE',  ( -336.3521761649654422, -86.34605966037949543, -45.90766452162698386 ) ) ;
#42830=EDGE_CURVE ( 'NONE', #50621, #34413, #47149, .T. ) ;
#42831=CARTESIAN_POINT ( 'NONE',  ( -336.3521761649654422, -158.3591674452439122, -47.62880233550485087 ) ) ;
#42833=CARTESIAN_POINT ( 'NONE',  ( -339.1964088526558498, -144.8891964568526305, -54.98865587491811624 ) ) ;
#42835=ORIENTED_EDGE ( 'NONE', *, *, #4942, .T. ) ;
#42836=EDGE_CURVE ( 'NONE', #50802, #16302, #46662, .T. ) ;
#42838=CARTESIAN_POINT ( 'NONE',  ( -339.1964088526558498, -71.02573290043838483, 26.97593913775504504 ) ) ;
#42844=CARTESIAN_POINT ( 'NONE',  ( -330.4913330509368166, -123.5000000000000284, 0.000000000000000000 ) ) ;
#42845=DIRECTION ( 'NONE',  ( 0.000000000000000000, 0.9350162426854158326, 0.3546048870425331234 ) ) ;
#42850=CARTESIAN_POINT ( 'NONE',  ( -336.3521761649653854, -88.08538291676191534, 48.43351006119235080 ) ) ;
#42851=LINE ( 'NONE', #22115, #2682 ) ;
#42863=ORIENTED_EDGE ( 'NONE', *, *, #35668, .T. ) ;
#42865=EDGE_LOOP ( 'NONE', ( #29278, #22768, #7695, #35230 ) ) ;
#42866=DIRECTION ( 'NONE',  ( -1.000000000000000000, 0.000000000000000000, 0.000000000000000000 ) ) ;
#42868=DIRECTION ( 'NONE',  ( -0.000000000000000000, 0.9350162426854146114, -0.3546048870425363986 ) ) ;
#42870=CARTESIAN_POINT ( 'NONE',  ( -332.3517673607765914, -177.7325358280884586, 23.38292116578760726 ) ) ;
#42873=PLANE ( 'NONE',  #12351 ) ;
#42876=ADVANCED_FACE ( 'NONE', ( #50604 ), #14601, .T. ) ;
#42878=ORIENTED_EDGE ( 'NONE', *, *, #12627, .F. ) ;
#42880=EDGE_LOOP ( 'NONE', ( #27932, #47551, #36406, #39937 ) ) ;
#42882=CARTESIAN_POINT ( 'NONE',  ( -330.4913330509368166, -175.5095439275177398, -27.86139516340860212 ) ) ;
#42883=DIRECTION ( 'NONE',  ( 0.000000000000000000, -0.1205366802553268363, -0.9927088740980534176 ) ) ;
#42885=ORIENTED_EDGE ( 'NONE', *, *, #26943, .T. ) ;
#42887=DIRECTION ( 'NONE',  ( -0.000000000000000000, -0.9350162426854169428, -0.3546048870425300148 ) ) ;
#42893=FACE_BOUND ( 'NONE', #149, .T. ) ;
#42898=VERTEX_POINT ( 'NONE', #46405 ) ;
#42903=EDGE_CURVE ( 'NONE', #32843, #47910, #34805, .T. ) ;
#42905=CARTESIAN_POINT ( 'NONE',  ( -339.1964088526558498, -75.22798428563991990, -33.92731199008514409 ) ) ;
#42907=ORIENTED_EDGE ( 'NONE', *, *, #30759, .T. ) ;
#42911=DIRECTION ( 'NONE',  ( 0.000000000000000000, 1.003826651431912330E-13, -1.000000000000000000 ) ) ;
#42913=ORIENTED_EDGE ( 'NONE', *, *, #15129, .F. ) ;
#42915=DIRECTION ( 'NONE',  ( 1.000000000000000000, 0.000000000000000000, 0.000000000000000000 ) ) ;
#42916=EDGE_CURVE ( 'NONE', #44016, #27425, #50098, .T. ) ;
#42921=EDGE_CURVE ( 'NONE', #12660, #2495, #25638, .T. ) ;
#42929=LINE ( 'NONE', #3757, #24128 ) ;
#42931=ORIENTED_EDGE ( 'NONE', *, *, #2216, .T. ) ;
#42936=EDGE_CURVE ( 'NONE', #25203, #42991, #10388, .T. ) ;
#42939=CARTESIAN_POINT ( 'NONE',  ( -336.3521761649654422, -70.03480886230919111, 25.08789112700620194 ) ) ;
#42940=DIRECTION ( 'NONE',  ( -0.000000000000000000, 0.1205366802553337752, 0.9927088740980526405 ) ) ;
#42941=ORIENTED_EDGE ( 'NONE', *, *, #41009, .T. ) ;
#42942=DIRECTION ( 'NONE',  ( 1.000000000000000000, -0.000000000000000000, -0.000000000000000000 ) ) ;
#42943=DIRECTION ( 'NONE',  ( 0.000000000000000000, 0.7485107481711069655, 0.6631226582407885317 ) ) ;
#42944=VECTOR ( 'NONE', #13199, 1000.000000000000000 ) ;
#42949=LINE ( 'NONE', #6710, #38194 ) ;
#42955=LINE ( 'NONE', #6965, #2416 ) ;
#42957=VERTEX_POINT ( 'NONE', #23000 ) ;
#42961=VECTOR ( 'NONE', #36647, 1000.000000000000000 ) ;
#42964=EDGE_CURVE ( 'NONE', #40712, #47727, #51144, .T. ) ;
#42968=VECTOR ( 'NONE', #9310, 1000.000000000000000 ) ;
#42969=CARTESIAN_POINT ( 'NONE',  ( -339.1964088526558498, -63.99980407363855761, 7.728304129923844634 ) ) ;
#42976=FACE_OUTER_BOUND ( 'NONE', #5059, .T. ) ;
#42981=ORIENTED_EDGE ( 'NONE', *, *, #32111, .T. ) ;
#42986=AXIS2_PLACEMENT_3D ( 'NONE', #36608, #24514, #40272 ) ;
#42987=ORIENTED_EDGE ( 'NONE', *, *, #29214, .T. ) ;
#42988=EDGE_CURVE ( 'NONE', #15810, #12661, #6888, .T. ) ;
#42991=VERTEX_POINT ( 'NONE', #3795 ) ;
#42992=DIRECTION ( 'NONE',  ( 1.000000000000000000, -0.000000000000000000, -0.000000000000000000 ) ) ;
#42999=EDGE_LOOP ( 'NONE', ( #33092, #49832, #23228, #39672 ) ) ;
#43003=DIRECTION ( 'NONE',  ( 0.000000000000000000, -0.7485107481710934207, 0.6631226582408039638 ) ) ;
#43008=AXIS2_PLACEMENT_3D ( 'NONE', #4733, #13131, #20761 ) ;
#43009=LINE ( 'NONE', #23038, #42514 ) ;
#43020=ORIENTED_EDGE ( 'NONE', *, *, #30379, .F. ) ;
#43022=VECTOR ( 'NONE', #10128, 1000.000000000000000 ) ;
#43027=VECTOR ( 'NONE', #33265, 1000.000000000000000 ) ;
#43028=CARTESIAN_POINT ( 'NONE',  ( -339.1964088526558498, -122.9999999999993605, 59.99791663049642665 ) ) ;
#43030=EDGE_LOOP ( 'NONE', ( #41739, #26632, #27445, #45886 ) ) ;
#43037=AXIS2_PLACEMENT_3D ( 'NONE', #31213, #3362, #31468 ) ;
#43048=ORIENTED_EDGE ( 'NONE', *, *, #1081, .F. ) ;
#43052=LINE ( 'NONE', #7060, #2453 ) ;
#43063=CIRCLE ( 'NONE', #4468, 60.00000000000000000 ) ;
#43065=DIRECTION ( 'NONE',  ( 0.000000000000000000, 0.000000000000000000, -1.000000000000000000 ) ) ;
#43066=VECTOR ( 'NONE', #40133, 1000.000000000000114 ) ;
#43067=PLANE ( 'NONE',  #44363 ) ;
#43071=LINE ( 'NONE', #19666, #1252 ) ;
#43076=VECTOR ( 'NONE', #33663, 1000.000000000000000 ) ;
#43078=PLANE ( 'NONE',  #9948 ) ;
#43079=ORIENTED_EDGE ( 'NONE', *, *, #35188, .F. ) ;
#43086=CARTESIAN_POINT ( 'NONE',  ( -305.0000000000000568, -174.3267994849386184, -31.88473700876087591 ) ) ;
#43087=FACE_OUTER_BOUND ( 'NONE', #21948, .T. ) ;
#43090=DIRECTION ( 'NONE',  ( -1.000000000000000000, 0.000000000000000000, -0.000000000000000000 ) ) ;
#43091=PLANE ( 'NONE',  #47567 ) ;
#43092=DIRECTION ( 'NONE',  ( -1.000000000000000000, -0.000000000000000000, 0.000000000000000000 ) ) ;
#43094=EDGE_CURVE ( 'NONE', #19724, #13250, #24542, .T. ) ;
#43095=ADVANCED_FACE ( 'NONE', ( #36369 ), #12705, .F. ) ;
#43096=AXIS2_PLACEMENT_3D ( 'NONE', #22406, #45807, #38676 ) ;
#43097=DIRECTION ( 'NONE',  ( -0.000000000000000000, 0.9709418174260553425, 0.2393156642875449158 ) ) ;
#43101=VECTOR ( 'NONE', #44331, 1000.000000000000000 ) ;
#43105=DIRECTION ( 'NONE',  ( 1.000000000000000000, -0.000000000000000000, -0.000000000000000000 ) ) ;
#43117=AXIS2_PLACEMENT_3D ( 'NONE', #25143, #49838, #1483 ) ;
#43120=VERTEX_POINT ( 'NONE', #32691 ) ;
#43126=ORIENTED_EDGE ( 'NONE', *, *, #35796, .F. ) ;
#43127=DIRECTION ( 'NONE',  ( 0.000000000000000000, 0.000000000000000000, 1.000000000000000000 ) ) ;
#43128=DIRECTION ( 'NONE',  ( 0.000000000000000000, 0.000000000000000000, 1.000000000000000000 ) ) ;
#43134=CARTESIAN_POINT ( 'NONE',  ( -339.1964088526558498, -162.2499814621209850, 44.49369547121574442 ) ) ;
#43135=VERTEX_POINT ( 'NONE', #40824 ) ;
#43136=CARTESIAN_POINT ( 'NONE',  ( -332.3517673607765914, -178.0871407151310279, 22.44790492310219676 ) ) ;
#43137=CARTESIAN_POINT ( 'NONE',  ( -332.3517673607765914, -106.8245764869328980, 56.65561927337994064 ) ) ;
#43140=ORIENTED_EDGE ( 'NONE', *, *, #21738, .F. ) ;
#43144=DIRECTION ( 'NONE',  ( 0.000000000000000000, -0.9927088740980526405, 0.1205366802553337890 ) ) ;
#43148=AXIS2_PLACEMENT_3D ( 'NONE', #16662, #19798, #8745 ) ;
#43153=FACE_BOUND ( 'NONE', #32796, .T. ) ;
#43155=AXIS2_PLACEMENT_3D ( 'NONE', #37683, #25333, #32942 ) ;
#43157=PLANE ( 'NONE',  #51808 ) ;
#43161=CARTESIAN_POINT ( 'NONE',  ( -336.3521761649654422, -73.44864141332200802, 31.34948880313848107 ) ) ;
#43162=VERTEX_POINT ( 'NONE', #32431 ) ;
#43166=AXIS2_PLACEMENT_3D ( 'NONE', #34588, #30646, #18061 ) ;
#43168=CARTESIAN_POINT ( 'NONE',  ( -305.0000000000000568, -150.9396941197150852, 53.35787839313398706 ) ) ;
#43171=DIRECTION ( 'NONE',  ( 1.043714542225393223E-14, 0.6631226582407863113, -0.7485107481711089639 ) ) ;
#43186=FACE_OUTER_BOUND ( 'NONE', #21881, .T. ) ;
#43193=CARTESIAN_POINT ( 'NONE',  ( -332.3517673607765914, -76.88706545914891421, 37.77875505479673279 ) ) ;
#43196=PLANE ( 'NONE',  #35661 ) ;
#43198=EDGE_CURVE ( 'NONE', #37735, #20132, #8510, .T. ) ;
#43204=DIRECTION ( 'NONE',  ( 0.000000000000000000, -2.914335439641035919E-13, -1.000000000000000000 ) ) ;
#43205=DIRECTION ( 'NONE',  ( 0.000000000000000000, 0.000000000000000000, 1.000000000000000000 ) ) ;
#43206=CARTESIAN_POINT ( 'NONE',  ( -339.1964088526558498, -156.6043281241909426, 48.84008046109164525 ) ) ;
#43209=DIRECTION ( 'NONE',  ( -1.000000000000000000, 8.589602288500749505E-15, -5.928974370889027093E-15 ) ) ;
#43213=CARTESIAN_POINT ( 'NONE',  ( -332.3517673607765914, -87.28260048324004572, 47.83617848703421771 ) ) ;
#43214=EDGE_CURVE ( 'NONE', #50151, #9197, #29269, .T. ) ;
#43218=VECTOR ( 'NONE', #49888, 1000.000000000000000 ) ;
#43231=DIRECTION ( 'NONE',  ( 1.000000000000000000, 0.000000000000000000, 0.000000000000000000 ) ) ;
#43232=DIRECTION ( 'NONE',  ( -0.000000000000000000, 0.000000000000000000, -1.000000000000000000 ) ) ;
#43235=EDGE_LOOP ( 'NONE', ( #10401, #44090, #21572, #34366 ) ) ;
#43238=ORIENTED_EDGE ( 'NONE', *, *, #11476, .T. ) ;
#43248=ORIENTED_EDGE ( 'NONE', *, *, #12627, .T. ) ;
#43250=ORIENTED_EDGE ( 'NONE', *, *, #50348, .T. ) ;
#43251=DIRECTION ( 'NONE',  ( 1.000000000000000000, -0.000000000000000000, -0.000000000000000000 ) ) ;
#43253=AXIS2_PLACEMENT_3D ( 'NONE', #3226, #51317, #35782 ) ;
#43255=CARTESIAN_POINT ( 'NONE',  ( -332.3517673607765914, -97.52665284734005979, -53.00046796564681983 ) ) ;
#43257=ORIENTED_EDGE ( 'NONE', *, *, #1563, .F. ) ;
#43258=CIRCLE ( 'NONE', #44127, 60.00000000000000000 ) ;
#43259=EDGE_CURVE ( 'NONE', #15531, #30167, #24504, .T. ) ;
#43260=EDGE_CURVE ( 'NONE', #41322, #27872, #37679, .T. ) ;
#43261=EDGE_CURVE ( 'NONE', #32390, #37883, #25851, .T. ) ;
#43264=VERTEX_POINT ( 'NONE', #22430 ) ;
#43267=EDGE_LOOP ( 'NONE', ( #42122, #7733, #7218, #8158 ) ) ;
#43271=EDGE_CURVE ( 'NONE', #34582, #4879, #42653, .T. ) ;
#43272=LINE ( 'NONE', #39061, #1453 ) ;
#43274=LINE ( 'NONE', #7286, #47319 ) ;
#43281=EDGE_CURVE ( 'NONE', #5750, #14193, #10334, .T. ) ;
#43284=EDGE_LOOP ( 'NONE', ( #1056, #45394, #20052, #11208 ) ) ;
#43286=CARTESIAN_POINT ( 'NONE',  ( -340.0000000000000568, -123.5000000000000142, 60.00000000000000000 ) ) ;
#43288=CARTESIAN_POINT ( 'NONE',  ( -336.3521761649654422, -78.25545813661345562, 37.90245108779119931 ) ) ;
#43289=DIRECTION ( 'NONE',  ( -0.000000000000000000, 0.000000000000000000, -1.000000000000000000 ) ) ;
#43300=CARTESIAN_POINT ( 'NONE',  ( -336.3521761649654422, -133.2247606357419443, -58.25253621232173629 ) ) ;
#43305=DIRECTION ( 'NONE',  ( -0.000000000000000000, 0.2393156642875448881, -0.9709418174260553425 ) ) ;
#43307=ADVANCED_FACE ( 'NONE', ( #1679 ), #18482, .T. ) ;
#43310=VECTOR ( 'NONE', #20925, 1000.000000000000000 ) ;
#43311=LINE ( 'NONE', #39365, #27068 ) ;
#43313=VECTOR ( 'NONE', #6410, 1000.000000000000114 ) ;
#43315=DIRECTION ( 'NONE',  ( 1.000000000000000000, -4.051632851310597467E-17, 7.719741424018539620E-17 ) ) ;
#43323=EDGE_CURVE ( 'NONE', #4472, #26301, #22165, .T. ) ;
#43328=LINE ( 'NONE', #43833, #4108 ) ;
#43330=EDGE_LOOP ( 'NONE', ( #36934, #26084, #11715, #17540 ) ) ;
#43331=CARTESIAN_POINT ( 'NONE',  ( -305.0000000000000568, -175.8491356171901145, 29.31839013542587935 ) ) ;
#43333=VERTEX_POINT ( 'NONE', #14808 ) ;
#43339=EDGE_LOOP ( 'NONE', ( #16006, #11249, #9459, #1676 ) ) ;
#43348=EDGE_LOOP ( 'NONE', ( #5884, #32668, #38129, #16242 ) ) ;
#43352=DIRECTION ( 'NONE',  ( -0.000000000000000000, 0.8229838658936613482, 0.5680647467311485954 ) ) ;
#43354=DIRECTION ( 'NONE',  ( 0.000000000000000000, -0.9350162426854121689, 0.3546048870425426713 ) ) ;
#43358=CARTESIAN_POINT ( 'NONE',  ( -332.3517673607765914, -135.0638248728647852, 57.91551518289418254 ) ) ;
#43359=DIRECTION ( 'NONE',  ( 1.000000000000000000, 0.000000000000000000, -0.000000000000000000 ) ) ;
#43361=VECTOR ( 'NONE', #8506, 1000.000000000000114 ) ;
#43363=ADVANCED_FACE ( 'NONE', ( #7166 ), #3729, .F. ) ;
#43366=VECTOR ( 'NONE', #6692, 1000.000000000000000 ) ;
#43368=DIRECTION ( 'NONE',  ( -0.000000000000000000, 0.000000000000000000, 1.000000000000000000 ) ) ;
#43374=DIRECTION ( 'NONE',  ( 0.000000000000000000, 0.000000000000000000, -1.000000000000000000 ) ) ;
#43375=CARTESIAN_POINT ( 'NONE',  ( -305.0000000000000568, -63.99980407363861445, -7.728304129924412180 ) ) ;
#43377=VERTEX_POINT ( 'NONE', #39715 ) ;
#43378=ORIENTED_EDGE ( 'NONE', *, *, #19525, .T. ) ;
#43384=CARTESIAN_POINT ( 'NONE',  ( -332.3517673607765914, -123.5000000000000284, 0.000000000000000000 ) ) ;
#43387=VERTEX_POINT ( 'NONE', #15845 ) ;
#43399=CARTESIAN_POINT ( 'NONE',  ( -339.1964088526558498, -138.1050951016792681, -57.16590939599323917 ) ) ;
#43400=VECTOR ( 'NONE', #27678, 1000.000000000000000 ) ;
#43402=VECTOR ( 'NONE', #26790, 1000.000000000000000 ) ;
#43404=DIRECTION ( 'NONE',  ( 1.043714542225393381E-14, -0.2393156642875582940, -0.9709418174260519008 ) ) ;
#43406=DIRECTION ( 'NONE',  ( 1.000000000000000000, -0.000000000000000000, 0.000000000000000000 ) ) ;
#43415=LINE ( 'NONE', #51553, #45838 ) ;
#43417=CARTESIAN_POINT ( 'NONE',  ( -339.1964088526558498, -96.52406086224361559, 52.47426709956096147 ) ) ;
#43418=AXIS2_PLACEMENT_3D ( 'NONE', #17114, #33120, #36537 ) ;
#43419=ORIENTED_EDGE ( 'NONE', *, *, #48573, .T. ) ;
#43425=VECTOR ( 'NONE', #18115, 999.9999999999998863 ) ;
#43429=CARTESIAN_POINT ( 'NONE',  ( -336.3521761649654422, -139.2044816956407089, -56.89493493766761389 ) ) ;
#43431=ORIENTED_EDGE ( 'NONE', *, *, #3608, .T. ) ;
#43437=CARTESIAN_POINT ( 'NONE',  ( -339.1964088526558498, -83.33976666099020747, -44.57752413667995484 ) ) ;
#43438=VECTOR ( 'NONE', #24593, 1000.000000000000000 ) ;
#43443=DIRECTION ( 'NONE',  ( 0.000000000000000000, 0.000000000000000000, 1.000000000000000000 ) ) ;
#43444=VECTOR ( 'NONE', #32276, 1000.000000000000000 ) ;
#43446=LINE ( 'NONE', #11880, #46583 ) ;
#43448=VERTEX_POINT ( 'NONE', #43161 ) ;
#43449=ORIENTED_EDGE ( 'NONE', *, *, #51654, .T. ) ;
#43455=ORIENTED_EDGE ( 'NONE', *, *, #32558, .F. ) ;
#43460=AXIS2_PLACEMENT_3D ( 'NONE', #48698, #15867, #32130 ) ;
#43463=CARTESIAN_POINT ( 'NONE',  ( -336.3521761649654422, -67.75522407825191351, 19.39547174791671935 ) ) ;
#43464=ORIENTED_EDGE ( 'NONE', *, *, #7411, .F. ) ;
#43466=VERTEX_POINT ( 'NONE', #43437 ) ;
#43468=CARTESIAN_POINT ( 'NONE',  ( -332.3517673607765914, -156.2279223070262049, 50.28800156563452362 ) ) ;
#43471=DIRECTION ( 'NONE',  ( 1.000000000000000000, -0.000000000000000000, 0.000000000000000000 ) ) ;
#43474=CARTESIAN_POINT ( 'NONE',  ( -330.4913330509368166, -123.5000000000000284, 0.000000000000000000 ) ) ;
#43475=FACE_OUTER_BOUND ( 'NONE', #43030, .T. ) ;
#43481=DIRECTION ( 'NONE',  ( 0.000000000000000000, -0.9350162426854158326, -0.3546048870425331789 ) ) ;
#43483=EDGE_CURVE ( 'NONE', #33612, #15472, #7682, .T. ) ;
#43484=DIRECTION ( 'NONE',  ( 0.000000000000000000, 0.000000000000000000, -1.000000000000000000 ) ) ;
#43485=CARTESIAN_POINT ( 'NONE',  ( -330.4913330509368166, -103.0458197858332312, -55.34326076196081345 ) ) ;
#43492=VECTOR ( 'NONE', #6876, 1000.000000000000000 ) ;
#43495=VECTOR ( 'NONE', #6626, 1000.000000000000000 ) ;
#43500=FACE_OUTER_BOUND ( 'NONE', #45634, .T. ) ;
#43501=VERTEX_POINT ( 'NONE', #36569 ) ;
#43504=CARTESIAN_POINT ( 'NONE',  ( -336.3521761649654422, -80.42027357919624819, -40.34602258462219027 ) ) ;
#43508=ORIENTED_EDGE ( 'NONE', *, *, #20495, .F. ) ;
#43510=VECTOR ( 'NONE', #43849, 1000.000000000000114 ) ;
#43512=DIRECTION ( 'NONE',  ( 0.000000000000000000, 0.000000000000000000, 1.000000000000000000 ) ) ;
#43517=CARTESIAN_POINT ( 'NONE',  ( -339.1964088526558498, -171.7720157143604069, -33.92731199008472487 ) ) ;
#43521=ORIENTED_EDGE ( 'NONE', *, *, #39806, .T. ) ;
#43542=DIRECTION ( 'NONE',  ( 0.000000000000000000, 0.9350162426854132791, -0.3546048870425396182 ) ) ;
#43544=FACE_OUTER_BOUND ( 'NONE', #30342, .T. ) ;
#43547=VERTEX_POINT ( 'NONE', #36309 ) ;
#43548=VECTOR ( 'NONE', #29050, 1000.000000000000114 ) ;
#43559=CARTESIAN_POINT ( 'NONE',  ( -332.3517673607765914, -69.26746417191145611, -23.38292116578723068 ) ) ;
#43563=LINE ( 'NONE', #27262, #25596 ) ;
#43564=VECTOR ( 'NONE', #16191, 1000.000000000000000 ) ;
#43568=EDGE_CURVE ( 'NONE', #31066, #34017, #33671, .T. ) ;
#43572=DIRECTION ( 'NONE',  ( -1.000000000000000000, -0.000000000000000000, -0.000000000000000000 ) ) ;
#43574=FACE_OUTER_BOUND ( 'NONE', #35831, .T. ) ;
#43578=ORIENTED_EDGE ( 'NONE', *, *, #12757, .T. ) ;
#43581=ORIENTED_EDGE ( 'NONE', *, *, #27607, .T. ) ;
#43582=CARTESIAN_POINT ( 'NONE',  ( -339.1964088526558498, -162.2499814621209850, 44.49369547121574442 ) ) ;
#43583=EDGE_CURVE ( 'NONE', #34438, #48449, #23573, .T. ) ;
#43587=DIRECTION ( 'NONE',  ( -0.000000000000000000, 0.8854560256532093554, -0.4647231720437695057 ) ) ;
#43590=CARTESIAN_POINT ( 'NONE',  ( -332.3517673607765914, -168.7445418633863596, -37.90245108779149064 ) ) ;
#43593=AXIS2_PLACEMENT_3D ( 'NONE', #29345, #38259, #41949 ) ;
#43598=VERTEX_POINT ( 'NONE', #5051 ) ;
#43601=FACE_OUTER_BOUND ( 'NONE', #18415, .T. ) ;
#43605=ORIENTED_EDGE ( 'NONE', *, *, #45769, .T. ) ;
#43608=CARTESIAN_POINT ( 'NONE',  ( -305.0000000000000568, -181.0704707379907745, 16.90091414705587525 ) ) ;
#43609=DIRECTION ( 'NONE',  ( -0.000000000000000000, -0.5680647467311485954, 0.8229838658936613482 ) ) ;
#43611=DIRECTION ( 'NONE',  ( 0.000000000000000000, 0.9927088740980551940, 0.1205366802553130001 ) ) ;
#43614=LINE ( 'NONE', #12326, #44810 ) ;
#43615=PLANE ( 'NONE',  #29031 ) ;
#43620=CARTESIAN_POINT ( 'NONE',  ( -339.1964088526558498, -182.0095552316575152, 7.608018572113563138 ) ) ;
#43621=DIRECTION ( 'NONE',  ( 0.000000000000000000, 0.000000000000000000, -1.000000000000000000 ) ) ;
#43625=ORIENTED_EDGE ( 'NONE', *, *, #14285, .F. ) ;
#43626=ADVANCED_FACE ( 'NONE', ( #10031 ), #49469, .F. ) ;
#43627=EDGE_CURVE ( 'NONE', #6745, #19363, #6339, .T. ) ;
#43632=EDGE_CURVE ( 'NONE', #4146, #5935, #30250, .T. ) ;
#43635=CARTESIAN_POINT ( 'NONE',  ( -330.4913330509368166, -162.9117225908391333, -45.24064679492040142 ) ) ;
#43636=EDGE_LOOP ( 'NONE', ( #1253, #9340, #14467, #42237 ) ) ;
#43645=EDGE_CURVE ( 'NONE', #18653, #46318, #41543, .T. ) ;
#43650=AXIS2_PLACEMENT_3D ( 'NONE', #8276, #36125, #44011 ) ;
#43652=DIRECTION ( 'NONE',  ( -0.000000000000000000, 0.9927088740980538617, -0.1205366802553232974 ) ) ;
#43658=CARTESIAN_POINT ( 'NONE',  ( -339.1964088526558498, -79.00630452878414189, 38.74998146212082162 ) ) ;
#43664=ADVANCED_FACE ( 'NONE', ( #49969 ), #38389, .F. ) ;
#43665=ORIENTED_EDGE ( 'NONE', *, *, #27844, .T. ) ;
#43666=DIRECTION ( 'NONE',  ( 0.000000000000000000, 0.000000000000000000, -1.000000000000000000 ) ) ;
#43688=VECTOR ( 'NONE', #2927, 1000.000000000000114 ) ;
#43689=ADVANCED_FACE ( 'NONE', ( #6084 ), #46044, .F. ) ;
#43698=FACE_OUTER_BOUND ( 'NONE', #20578, .T. ) ;
#43701=VERTEX_POINT ( 'NONE', #9763 ) ;
#43705=ORIENTED_EDGE ( 'NONE', *, *, #41321, .T. ) ;
#43707=CARTESIAN_POINT ( 'NONE',  ( -339.1964088526558498, -143.9541802141672235, -55.34326076196065003 ) ) ;
#43711=EDGE_LOOP ( 'NONE', ( #5167, #7458, #45989, #2447 ) ) ;
#43716=CARTESIAN_POINT ( 'NONE',  ( -305.0000000000000568, -80.37812621821328207, -41.71934804796994456 ) ) ;
#43725=VERTEX_POINT ( 'NONE', #3165 ) ;
#43729=LINE ( 'NONE', #15624, #37567 ) ;
#43731=LINE ( 'NONE', #15369, #14820 ) ;
#43732=CARTESIAN_POINT ( 'NONE',  ( -336.3521761649654422, -100.1170788342122080, 54.23253582808833073 ) ) ;
#43733=CARTESIAN_POINT ( 'NONE',  ( -330.4913330509368166, -66.09477493971917283, -13.63415328425296202 ) ) ;
#43734=ORIENTED_EDGE ( 'NONE', *, *, #13065, .F. ) ;
#43745=DIRECTION ( 'NONE',  ( 1.000000000000000000, -0.000000000000000000, -0.000000000000000000 ) ) ;
#43748=VERTEX_POINT ( 'NONE', #4387 ) ;
#43753=VECTOR ( 'NONE', #19577, 1000.000000000000000 ) ;
#43755=LINE ( 'NONE', #7757, #30501 ) ;
#43756=VECTOR ( 'NONE', #18027, 1000.000000000000000 ) ;
#43757=VECTOR ( 'NONE', #10602, 1000.000000000000114 ) ;
#43758=DIRECTION ( 'NONE',  ( -0.000000000000000000, -0.6631226582407989678, -0.7485107481710977506 ) ) ;
#43759=EDGE_LOOP ( 'NONE', ( #16512, #34581, #18695, #45841 ) ) ;
#43763=ORIENTED_EDGE ( 'NONE', *, *, #49547, .F. ) ;
#43769=AXIS2_PLACEMENT_3D ( 'NONE', #19076, #31402, #31670 ) ;
#43771=ORIENTED_EDGE ( 'NONE', *, *, #23469, .T. ) ;
#43777=LINE ( 'NONE', #15940, #30589 ) ;
#43780=CARTESIAN_POINT ( 'NONE',  ( -330.4913330509368166, -182.0095552316575152, 7.608018572113473432 ) ) ;
#43783=ORIENTED_EDGE ( 'NONE', *, *, #42936, .F. ) ;
#43785=EDGE_CURVE ( 'NONE', #11713, #49096, #7108, .T. ) ;
#43786=LINE ( 'NONE', #154, #49316 ) ;
#43787=CARTESIAN_POINT ( 'NONE',  ( -332.3517673607765914, -180.3949349376675855, 15.70448169564087770 ) ) ;
#43798=LINE ( 'NONE', #7799, #20381 ) ;
#43799=DIRECTION ( 'NONE',  ( 1.000000000000000000, -8.465038975556420946E-17, -2.086444717177458678E-17 ) ) ;
#43804=EDGE_LOOP ( 'NONE', ( #1760, #20134, #50765, #11442 ) ) ;
#43805=CARTESIAN_POINT ( 'NONE',  ( -332.3517673607765914, -85.72124494520284088, -46.61293454085073051 ) ) ;
#43810=AXIS2_PLACEMENT_3D ( 'NONE', #14245, #9777, #22376 ) ;
#43812=CIRCLE ( 'NONE', #1878, 60.00000000000000000 ) ;
#43824=CARTESIAN_POINT ( 'NONE',  ( -305.0000000000000568, -63.50208336950359467, 0.4999999999999573119 ) ) ;
#43826=EDGE_LOOP ( 'NONE', ( #35804, #32631, #15224, #37970 ) ) ;
#43833=CARTESIAN_POINT ( 'NONE',  ( -336.3521761649654422, -88.64083255475578937, 47.62880233550460218 ) ) ;
#43835=ORIENTED_EDGE ( 'NONE', *, *, #37705, .T. ) ;
#43836=LINE ( 'NONE', #27291, #9908 ) ;
#43838=ORIENTED_EDGE ( 'NONE', *, *, #20080, .T. ) ;
#43840=VECTOR ( 'NONE', #50752, 1000.000000000000000 ) ;
#43841=EDGE_LOOP ( 'NONE', ( #44716, #18223, #19556, #34242 ) ) ;
#43843=ORIENTED_EDGE ( 'NONE', *, *, #10879, .T. ) ;
#43844=CARTESIAN_POINT ( 'NONE',  ( -336.3521761649654422, -170.5607375887735770, 35.68215131113770155 ) ) ;
#43845=VERTEX_POINT ( 'NONE', #51515 ) ;
#43846=EDGE_CURVE ( 'NONE', #34815, #31384, #39409, .T. ) ;
#43848=CLOSED_SHELL ( 'NONE', ( #14761, #40148, #4407, #3264, #18551, #4535, #43307, #17841, #5383, #46806, #26903, #6095, #23828, #39996, #36059, #5738, #34898, #907, #1709, #10231, #16047, #3773, #29156, #33314, #10919, #33123, #18435, #9635, #40590, #16668, #740, #4807, #23347, #19197, #40918, #38982, #20063, #18163, #34953, #20885, #38120, #21868, #38033, #13969, #33674, #49422, #25642, #11997, #30904, #29884, #29215, #3000, #17071, #40722, #49748, #30695, #21152, #16707, #37805, #9009, #27306, #39697, #20902, #8508, #41613, #49405, #18928, #21806, #33840, #16437, #5736, #49450, #49156, #34029, #18882, #3120, #43939, #49262, #20377, #33405, #29565, #46970, #41115, #44965, #29753, #12544, #34973, #7425, #539, #11361, #47730, #28731, #18948, #28744, #42320, #31132, #50077, #34077, #28199, #8269, #6150, #34024, #2823, #42506, #41827, #18265, #9812, #13113, #39923, #41974, #51369, #27542, #39051, #36737, #23683, #47906, #48370, #22385, #8608, #20151, #9652, #26825, #19317, #6089, #11159, #51018, #17190, #10292, #7991, #35117, #8592, #42265, #6747, #48438, #4416, #34343, #22134, #36193, #46394, #13662, #39280, #2406, #43909, #47645, #27258, #44060, #27713, #36191, #39194, #49746, #2537, #43868, #25485, #10814, #6915, #5461, #14036, #9192, #2004, #18890, #20671, #29748, #50758, #48925, #28432, #3416, #46610, #48514, #15035, #51969, #31448, #12452, #10920, #26360, #49841, #43363, #30812, #49409, #23930, #44314, #13072, #9290, #20181, #25538, #48736, #41236, #8338, #7034, #22699, #12792, #31410, #49408, #46314, #4344, #26844, #2473, #32875, #10233, #19081, #38902, #16646, #931, #35650, #36632, #34099, #47085, #23061, #44279, #144, #40792, #4404, #19602, #8966, #15765, #1979, #13157, #19442, #44290, #24052, #7834, #9466, #31127, #184, #15010, #14033, #22386, #2413, #28540, #49089, #14049, #33623, #36323, #21798, #24696, #41901, #26607, #27637, #36573, #30747, #47560, #2164, #13779, #37406, #19762, #32176, #41617, #45677, #43626, #36601, #21575, #15860, #35975, #9286, #24713, #33807, #46891, #3311, #31800, #2811, #44527, #25072, #36081, #43931, #27546, #36221, #50303, #8134, #15799, #48636, #29999, #6898, #47022, #5762, #24373, #41738, #3007, #9703, #2885, #32162, #37724, #11466, #4029, #21682, #14339, #18816, #21748, #1607, #6097, #6576, #3465, #1283, #1859, #28343, #45919, #38116, #18615, #9947, #50467, #15443, #23037, #12357, #47704, #6903, #44703, #34693, #29473, #11301, #36873, #18892, #14137, #135, #37584, #24711, #34620, #46551, #2518, #5918, #23258, #50343, #6380, #3474, #45370, #41915, #27026, #3964, #16999, #29676, #2286, #32793, #7941, #10309, #29668, #40356, #538, #50047, #2859, #20532, #3826, #18829, #18622, #42375, #51423, #40300, #13754, #16029, #1868, #27886, #2168, #35733, #27887, #28492, #39656, #25073, #11522, #38743, #49346, #13398, #1750, #33029, #41868, #12061, #21446, #24946, #51800, #41717, #14381, #49416, #41090, #1948, #33063, #24535, #38479, #42180, #28480, #38646, #30990, #46704, #38423, #7909, #49123, #15014, #14819, #16539, #12890, #47146, #38850, #37342, #34482, #52028, #17947, #198, #22736, #5390, #21226, #11869, #13805, #50182, #31763, #21458, #23633, #15534, #19849, #35477, #50585, #47265, #46195, #13796, #13493, #40696, #5457, #9783, #26041, #50498, #26824, #15326, #30456, #40201, #47488, #17043, #38509, #34215, #36824, #43689, #42876, #35537, #21206, #37101, #29949, #49306, #24297, #41135, #23035, #51705, #46217, #46737, #3662, #982, #24640, #32670, #48798, #34625, #51062, #1327, #32734, #24131, #44581, #26379, #45554, #46255, #18336, #51686, #12292, #13345, #3865, #39477, #48075, #20854, #9602, #32407, #47382, #15714, #8222, #46151, #17250, #37587, #33896, #17597, #28196, #25716, #19526, #5071, #43095, #25233, #16174, #17142, #16511, #34465, #23422, #26772, #44764, #50787, #21542, #13749, #33989, #20607, #25300, #48734, #5222, #41408, #24369, #1091, #8365, #12504, #36947, #30224, #16007, #6391, #51736, #30818, #29004, #27784, #34206, #45079, #38842, #45772, #7229, #4993, #33086, #33718, #50003, #20247, #44645, #45402, #35848, #47745, #3388, #20440, #42700, #27862, #44288, #47133, #1856, #16604, #1259, #36555, #51308, #14592, #21142, #46187, #43664, #50416, #37873, #1531, #38221, #1202, #13744, #51964, #21272, #36444, #31852, #18776, #17019, #12477, #28419 ) ) ;
#43849=DIRECTION ( 'NONE',  ( -0.000000000000000000, 0.7485107481710999711, -0.6631226582407964143 ) ) ;
#43859=PLANE ( 'NONE',  #36723 ) ;
#43868=ADVANCED_FACE ( 'NONE', ( #42592 ), #38641, .F. ) ;
#43870=CARTESIAN_POINT ( 'NONE',  ( -339.1964088526558498, -90.39567187580801999, 48.84008046109089918 ) ) ;
#43873=CARTESIAN_POINT ( 'NONE',  ( -336.3521761649654422, -181.7525362123217292, 9.724760635742144999 ) ) ;
#43875=LINE ( 'NONE', #45206, #50455 ) ;
#43876=DIRECTION ( 'NONE',  ( 1.000000000000000000, -0.000000000000000000, 0.000000000000000000 ) ) ;
#43877=ORIENTED_EDGE ( 'NONE', *, *, #45845, .F. ) ;
#43886=LINE ( 'NONE', #3955, #2757 ) ;
#43899=CARTESIAN_POINT ( 'NONE',  ( -339.1964088526558498, -123.5000000000000284, 0.000000000000000000 ) ) ;
#43901=DIRECTION ( 'NONE',  ( -0.000000000000000000, -0.000000000000000000, -1.000000000000000000 ) ) ;
#43903=DIRECTION ( 'NONE',  ( 1.000000000000000000, -0.000000000000000000, -0.000000000000000000 ) ) ;
#43905=CARTESIAN_POINT ( 'NONE',  ( -339.1964088526558498, -79.66942718702553350, -39.49849221029258928 ) ) ;
#43909=ADVANCED_FACE ( 'NONE', ( #49326 ), #25403, .F. ) ;
#43911=DIRECTION ( 'NONE',  ( 0.000000000000000000, -0.8854560256532079121, 0.4647231720437725033 ) ) ;
#43914=VECTOR ( 'NONE', #23184, 999.9999999999998863 ) ;
#43926=ORIENTED_EDGE ( 'NONE', *, *, #33069, .F. ) ;
#43931=ADVANCED_FACE ( 'NONE', ( #45385 ), #29066, .F. ) ;
#43934=ORIENTED_EDGE ( 'NONE', *, *, #46194, .F. ) ;
#43938=VECTOR ( 'NONE', #32503, 1000.000000000000114 ) ;
#43939=ADVANCED_FACE ( 'NONE', ( #44593 ), #45644, .F. ) ;
#43940=DIRECTION ( 'NONE',  ( -1.000000000000000000, 0.000000000000000000, 0.000000000000000000 ) ) ;
#43942=CARTESIAN_POINT ( 'NONE',  ( -336.3521761649654422, -106.8245764869328980, 56.65561927337994064 ) ) ;
#43945=FACE_OUTER_BOUND ( 'NONE', #49618, .T. ) ;
#43948=ORIENTED_EDGE ( 'NONE', *, *, #12163, .T. ) ;
#43950=PLANE ( 'NONE',  #29116 ) ;
#43951=AXIS2_PLACEMENT_3D ( 'NONE', #46830, #36203, #44375 ) ;
#43952=EDGE_CURVE ( 'NONE', #809, #23381, #5174, .T. ) ;
#43955=EDGE_LOOP ( 'NONE', ( #26575, #28696, #4835, #2703 ) ) ;
#43957=DIRECTION ( 'NONE',  ( -8.718379230999707126E-17, 0.2393156642875516604, -0.9709418174260535661 ) ) ;
#43959=CARTESIAN_POINT ( 'NONE',  ( 0.000000000000000000, -109.3803758070334737, 57.28556722813694080 ) ) ;
#43963=ORIENTED_EDGE ( 'NONE', *, *, #46090, .F. ) ;
#43965=CARTESIAN_POINT ( 'NONE',  ( -336.3521761649654422, -65.58448481710581746, 11.56382487286456140 ) ) ;
#43966=CARTESIAN_POINT ( 'NONE',  ( -332.3517673607765914, -182.2665742509934148, -5.491276508484069119 ) ) ;
#43967=CARTESIAN_POINT ( 'NONE',  ( -330.4913330509368166, -178.8432607619609200, -20.45418021416661247 ) ) ;
#43969=CARTESIAN_POINT ( 'NONE',  ( -339.1964088526558498, -172.3400804610915600, -33.10432812419107051 ) ) ;
#43974=EDGE_CURVE ( 'NONE', #49096, #36522, #45132, .T. ) ;
#43976=EDGE_CURVE ( 'NONE', #20460, #21321, #17265, .T. ) ;
#43979=CARTESIAN_POINT ( 'NONE',  ( -336.3521761649654422, -176.9651911376907094, -25.08789112700655721 ) ) ;
#43981=EDGE_CURVE ( 'NONE', #27241, #49313, #5441, .T. ) ;
#43985=CARTESIAN_POINT ( 'NONE',  ( -339.1964088526558498, -151.3613951634092700, -52.00954392751739164 ) ) ;
#43988=DIRECTION ( 'NONE',  ( -1.000000000000000000, -0.000000000000000000, 0.000000000000000000 ) ) ;
#43989=DIRECTION ( 'NONE',  ( -1.000000000000000000, 0.000000000000000000, -0.000000000000000000 ) ) ;
#43990=PLANE ( 'NONE',  #23447 ) ;
#43992=FACE_OUTER_BOUND ( 'NONE', #11603, .T. ) ;
#43994=ORIENTED_EDGE ( 'NONE', *, *, #28772, .F. ) ;
#43997=DIRECTION ( 'NONE',  ( 0.000000000000000000, 0.000000000000000000, 1.000000000000000000 ) ) ;
#44001=EDGE_CURVE ( 'NONE', #39339, #38101, #33795, .T. ) ;
#44004=CARTESIAN_POINT ( 'NONE',  ( -339.1964088526558498, -162.9117225908391333, -45.24064679492040142 ) ) ;
#44006=EDGE_CURVE ( 'NONE', #2225, #48882, #3027, .T. ) ;
#44008=CARTESIAN_POINT ( 'NONE',  ( -336.3521761649654422, -69.26746417191145611, -23.38292116578723068 ) ) ;
#44010=ORIENTED_EDGE ( 'NONE', *, *, #26326, .F. ) ;
#44011=DIRECTION ( 'NONE',  ( 0.000000000000000000, -0.1205366802553095168, 0.9927088740980556381 ) ) ;
#44013=ORIENTED_EDGE ( 'NONE', *, *, #13788, .T. ) ;
#44016=VERTEX_POINT ( 'NONE', #10921 ) ;
#44017=LINE ( 'NONE', #36656, #38275 ) ;
#44018=AXIS2_PLACEMENT_3D ( 'NONE', #50608, #10658, #26690 ) ;
#44020=CARTESIAN_POINT ( 'NONE',  ( -336.3521761649654422, -81.08339623743702873, -41.09453333279329712 ) ) ;
#44021=ORIENTED_EDGE ( 'NONE', *, *, #7857, .F. ) ;
#44022=CARTESIAN_POINT ( 'NONE',  ( -336.3521761649654422, -159.1821513111375452, -47.06073758877369073 ) ) ;
#44023=DIRECTION ( 'NONE',  ( 0.000000000000000000, 0.000000000000000000, 1.000000000000000000 ) ) ;
#44025=DIRECTION ( 'NONE',  ( 0.000000000000000000, 0.000000000000000000, 1.000000000000000000 ) ) ;
#44026=CARTESIAN_POINT ( 'NONE',  ( -332.3517673607765914, -153.2494431741581025, -51.01861988938816950 ) ) ;
#44027=DIRECTION ( 'NONE',  ( 1.000000000000000000, -0.000000000000000000, 0.000000000000000000 ) ) ;
#44031=ORIENTED_EDGE ( 'NONE', *, *, #44885, .F. ) ;
#44036=FACE_BOUND ( 'NONE', #49121, .T. ) ;
#44037=DIRECTION ( 'NONE',  ( 0.000000000000000000, -0.3546048870425426158, -0.9350162426854120579 ) ) ;
#44039=EDGE_CURVE ( 'NONE', #32740, #34582, #6980, .T. ) ;
#44050=AXIS2_PLACEMENT_3D ( 'NONE', #10721, #38823, #29910 ) ;
#44051=CARTESIAN_POINT ( 'NONE',  ( -339.1964088526558498, -151.3613951634084742, 52.00954392751779665 ) ) ;
#44052=LINE ( 'NONE', #5164, #43548 ) ;
#44053=ORIENTED_EDGE ( 'NONE', *, *, #36918, .T. ) ;
#44055=ORIENTED_EDGE ( 'NONE', *, *, #47731, .T. ) ;
#44060=ADVANCED_FACE ( 'NONE', ( #18037 ), #13834, .F. ) ;
#44071=EDGE_CURVE ( 'NONE', #19790, #18653, #30894, .T. ) ;
#44075=DIRECTION ( 'NONE',  ( -0.000000000000000000, 0.2393156642875448881, -0.9709418174260553425 ) ) ;
#44079=ORIENTED_EDGE ( 'NONE', *, *, #20009, .F. ) ;
#44085=AXIS2_PLACEMENT_3D ( 'NONE', #8451, #40761, #20814 ) ;
#44088=CIRCLE ( 'NONE', #13029, 60.00000000000000000 ) ;
#44090=ORIENTED_EDGE ( 'NONE', *, *, #27479, .T. ) ;
#44091=FACE_OUTER_BOUND ( 'NONE', #29611, .T. ) ;
#44093=AXIS2_PLACEMENT_3D ( 'NONE', #39823, #47994, #16732 ) ;
#44096=CARTESIAN_POINT ( 'NONE',  ( -330.4913330509368166, -115.8919814278863356, 58.50955523165747252 ) ) ;
#44100=CARTESIAN_POINT ( 'NONE',  ( -339.1964088526558498, -95.63860483659122735, -52.00954392751761191 ) ) ;
#44114=CARTESIAN_POINT ( 'NONE',  ( -330.4913330509368166, -178.8432607619609200, -20.45418021416661247 ) ) ;
#44115=CARTESIAN_POINT ( 'NONE',  ( -336.3521761649654422, -70.03480886230919111, 25.08789112700620194 ) ) ;
#44119=VECTOR ( 'NONE', #41219, 1000.000000000000000 ) ;
#44122=DIRECTION ( 'NONE',  ( -1.000000000000000000, 0.000000000000000000, 0.000000000000000000 ) ) ;
#44127=AXIS2_PLACEMENT_3D ( 'NONE', #4004, #8713, #52 ) ;
#44131=CARTESIAN_POINT ( 'NONE',  ( -339.1964088526558498, -95.63860483659122735, -52.00954392751761191 ) ) ;
#44134=ORIENTED_EDGE ( 'NONE', *, *, #4403, .F. ) ;
#44137=VECTOR ( 'NONE', #110, 1000.000000000000000 ) ;
#44138=DIRECTION ( 'NONE',  ( -1.000000000000000000, 0.000000000000000000, -0.000000000000000000 ) ) ;
#44139=FACE_OUTER_BOUND ( 'NONE', #43348, .T. ) ;
#44143=ORIENTED_EDGE ( 'NONE', *, *, #3739, .T. ) ;
#44146=CARTESIAN_POINT ( 'NONE',  ( -336.3521761649654422, -65.12692710742291524, -8.732051761643681687 ) ) ;
#44150=DIRECTION ( 'NONE',  ( -0.000000000000000000, 0.8854560256532093554, -0.4647231720437695057 ) ) ;
#44151=ORIENTED_EDGE ( 'NONE', *, *, #35318, .T. ) ;
#44155=CIRCLE ( 'NONE', #30717, 60.00000000000000000 ) ;
#44157=VERTEX_POINT ( 'NONE', #22227 ) ;
#44160=VECTOR ( 'NONE', #39214, 1000.000000000000000 ) ;
#44166=PLANE ( 'NONE',  #34458 ) ;
#44168=FACE_OUTER_BOUND ( 'NONE', #40307, .T. ) ;
#44171=EDGE_CURVE ( 'NONE', #50347, #51592, #35592, .T. ) ;
#44174=PLANE ( 'NONE',  #2953 ) ;
#44175=AXIS2_PLACEMENT_3D ( 'NONE', #21118, #359, #5363 ) ;
#44177=DIRECTION ( 'NONE',  ( 0.000000000000000000, 0.9350162426854146114, -0.3546048870425363986 ) ) ;
#44181=PLANE ( 'NONE',  #6198 ) ;
#44182=DIRECTION ( 'NONE',  ( -1.000000000000000000, 2.497772389992620524E-15, 1.013386094502321458E-14 ) ) ;
#44184=ORIENTED_EDGE ( 'NONE', *, *, #44006, .T. ) ;
#44189=VECTOR ( 'NONE', #35695, 999.9999999999998863 ) ;
#44195=LINE ( 'NONE', #3998, #47468 ) ;
#44197=CARTESIAN_POINT ( 'NONE',  ( -336.3521761649653854, -139.4384828369889249, -57.84431488793872944 ) ) ;
#44201=LINE ( 'NONE', #36053, #21432 ) ;
#44204=DIRECTION ( 'NONE',  ( -1.000000000000000000, -0.000000000000000000, 0.000000000000000000 ) ) ;
#44206=DIRECTION ( 'NONE',  ( 0.000000000000000000, 0.9709418174260502354, -0.2393156642875652051 ) ) ;
#44207=CARTESIAN_POINT ( 'NONE',  ( -336.3521761649654422, -181.4155151828941825, -11.56382487286496463 ) ) ;
#44211=CARTESIAN_POINT ( 'NONE',  ( -339.1964088526558498, -74.65991953890826949, 33.10432812419072945 ) ) ;
#44212=CARTESIAN_POINT ( 'NONE',  ( -336.3521761649654422, -161.4024510877913485, 45.24454186338643780 ) ) ;
#44218=EDGE_CURVE ( 'NONE', #11822, #28559, #23276, .T. ) ;
#44219=DIRECTION ( 'NONE',  ( -0.000000000000000000, 0.000000000000000000, 1.000000000000000000 ) ) ;
#44220=CIRCLE ( 'NONE', #34135, 60.00000000000000000 ) ;
#44221=VECTOR ( 'NONE', #21834, 1000.000000000000000 ) ;
#44226=DIRECTION ( 'NONE',  ( -0.000000000000000000, -0.4647231720437604574, 0.8854560256532141294 ) ) ;
#44234=ORIENTED_EDGE ( 'NONE', *, *, #9964, .F. ) ;
#44241=DIRECTION ( 'NONE',  ( 1.000000000000000000, -0.000000000000000000, -0.000000000000000000 ) ) ;
#44247=CARTESIAN_POINT ( 'NONE',  ( -339.1964088526558498, -84.75001853787875916, -44.49369547121548862 ) ) ;
#44248=DIRECTION ( 'NONE',  ( -0.000000000000000000, -1.000000000000000000, 3.491481338843133355E-15 ) ) ;
#44255=LINE ( 'NONE', #36357, #32527 ) ;
#44256=VECTOR ( 'NONE', #7963, 1000.000000000000000 ) ;
#44258=DIRECTION ( 'NONE',  ( 0.000000000000000000, 0.7485107481710953081, -0.6631226582408016323 ) ) ;
#44259=VECTOR ( 'NONE', #46979, 1000.000000000000114 ) ;
#44262=FACE_OUTER_BOUND ( 'NONE', #33299, .T. ) ;
#44271=ORIENTED_EDGE ( 'NONE', *, *, #40446, .T. ) ;
#44272=FACE_OUTER_BOUND ( 'NONE', #17318, .T. ) ;
#44276=ORIENTED_EDGE ( 'NONE', *, *, #19334, .F. ) ;
#44279=ADVANCED_FACE ( 'NONE', ( #15387 ), #24041, .F. ) ;
#44286=AXIS2_PLACEMENT_3D ( 'NONE', #17741, #34008, #45088 ) ;
#44288=ADVANCED_FACE ( 'NONE', ( #11939 ), #47441, .F. ) ;
#44290=ADVANCED_FACE ( 'NONE', ( #43500 ), #31144, .F. ) ;
#44292=EDGE_CURVE ( 'NONE', #29433, #18178, #39535, .T. ) ;
#44295=CIRCLE ( 'NONE', #27515, 60.00000000000000000 ) ;
#44297=DIRECTION ( 'NONE',  ( -1.000000000000000000, 0.000000000000000000, 0.000000000000000000 ) ) ;
#44301=DIRECTION ( 'NONE',  ( -1.000000000000000000, 0.000000000000000000, 0.000000000000000000 ) ) ;
#44305=DIRECTION ( 'NONE',  ( 1.000000000000000000, 0.000000000000000000, 0.000000000000000000 ) ) ;
#44313=CARTESIAN_POINT ( 'NONE',  ( -332.3517673607765914, -181.0704707379907745, 16.90091414705587525 ) ) ;
#44314=ADVANCED_FACE ( 'NONE', ( #48493 ), #8777, .F. ) ;
#44316=FACE_BOUND ( 'NONE', #26865, .T. ) ;
#44317=CARTESIAN_POINT ( 'NONE',  ( -305.0000000000000568, -126.1322888500942554, -59.94223098458773080 ) ) ;
#44320=EDGE_CURVE ( 'NONE', #41179, #16323, #49000, .T. ) ;
#44322=LINE ( 'NONE', #40602, #44935 ) ;
#44323=ORIENTED_EDGE ( 'NONE', *, *, #38489, .T. ) ;
#44324=LINE ( 'NONE', #31181, #37204 ) ;
#44326=EDGE_LOOP ( 'NONE', ( #39972, #12490, #49540, #35270 ) ) ;
#44331=DIRECTION ( 'NONE',  ( -1.000000000000000000, -8.589602288500833124E-15, -5.928974370888904820E-15 ) ) ;
#44334=CARTESIAN_POINT ( 'NONE',  ( -336.3521761649654422, -128.9912765084839066, 58.76657425099337928 ) ) ;
#44347=DIRECTION ( 'NONE',  ( 0.000000000000000000, 0.000000000000000000, -1.000000000000000000 ) ) ;
#44351=DIRECTION ( 'NONE',  ( -0.000000000000000000, -0.6631226582407885317, 0.7485107481711069655 ) ) ;
#44354=VERTEX_POINT ( 'NONE', #36377 ) ;
#44357=ORIENTED_EDGE ( 'NONE', *, *, #11877, .F. ) ;
#44359=EDGE_CURVE ( 'NONE', #48723, #7602, #20892, .T. ) ;
#44363=AXIS2_PLACEMENT_3D ( 'NONE', #19162, #50456, #30213 ) ;
#44366=ORIENTED_EDGE ( 'NONE', *, *, #47034, .T. ) ;
#44368=EDGE_LOOP ( 'NONE', ( #5857, #41025, #18106, #43838 ) ) ;
#44371=AXIS2_PLACEMENT_3D ( 'NONE', #18823, #6504, #46439 ) ;
#44375=DIRECTION ( 'NONE',  ( 0.000000000000000000, 0.000000000000000000, 1.000000000000000000 ) ) ;
#44380=ORIENTED_EDGE ( 'NONE', *, *, #46865, .F. ) ;
#44382=PLANE ( 'NONE',  #18887 ) ;
#44386=EDGE_LOOP ( 'NONE', ( #20833, #748, #10295, #47946 ) ) ;
#44388=VERTEX_POINT ( 'NONE', #21128 ) ;
#44391=ORIENTED_EDGE ( 'NONE', *, *, #5627, .F. ) ;
#44392=CARTESIAN_POINT ( 'NONE',  ( -339.1964088526558498, -157.9941932480463436, 49.09328500076600221 ) ) ;
#44395=ORIENTED_EDGE ( 'NONE', *, *, #6717, .F. ) ;
#44401=FACE_OUTER_BOUND ( 'NONE', #30221, .T. ) ;
#44408=CARTESIAN_POINT ( 'NONE',  ( -336.3521761649654422, -70.49953203435293858, 25.97334715265942151 ) ) ;
#44413=CARTESIAN_POINT ( 'NONE',  ( -332.3517673607765914, -181.7525362123217292, 9.724760635742144999 ) ) ;
#44414=DIRECTION ( 'NONE',  ( 0.000000000000000000, 0.000000000000000000, 1.000000000000000000 ) ) ;
#44417=VERTEX_POINT ( 'NONE', #33216 ) ;
#44418=ORIENTED_EDGE ( 'NONE', *, *, #30302, .T. ) ;
#44422=DIRECTION ( 'NONE',  ( 0.000000000000000000, -1.420160285666346159E-13, -1.000000000000000000 ) ) ;
#44426=DIRECTION ( 'NONE',  ( 0.000000000000000000, 0.5680647467311569221, 0.8229838658936556861 ) ) ;
#44430=ORIENTED_EDGE ( 'NONE', *, *, #25647, .T. ) ;
#44438=EDGE_LOOP ( 'NONE', ( #20115, #31133, #37772, #35904, #26103, #32373, #24822, #4692, #22127, #47007, #38957, #35621 ) ) ;
#44439=EDGE_CURVE ( 'NONE', #37940, #30972, #41354, .T. ) ;
#44441=ORIENTED_EDGE ( 'NONE', *, *, #43981, .T. ) ;
#44449=DIRECTION ( 'NONE',  ( 0.000000000000000000, 0.000000000000000000, -1.000000000000000000 ) ) ;
#44450=VERTEX_POINT ( 'NONE', #11611 ) ;
#44451=VECTOR ( 'NONE', #6072, 1000.000000000000114 ) ;
#44457=LINE ( 'NONE', #16332, #47552 ) ;
#44460=DIRECTION ( 'NONE',  ( 1.000000000000000000, -0.000000000000000000, 0.000000000000000000 ) ) ;
#44465=AXIS2_PLACEMENT_3D ( 'NONE', #5717, #1752, #21470 ) ;
#44467=DIRECTION ( 'NONE',  ( -1.000000000000000000, -0.000000000000000000, 0.000000000000000000 ) ) ;
#44470=LINE ( 'NONE', #8717, #33328 ) ;
#44478=ORIENTED_EDGE ( 'NONE', *, *, #11042, .T. ) ;
#44483=ORIENTED_EDGE ( 'NONE', *, *, #17395, .F. ) ;
#44488=CARTESIAN_POINT ( 'NONE',  ( -336.3521761649654422, -106.8245764869328980, 56.65561927337994064 ) ) ;
#44492=ORIENTED_EDGE ( 'NONE', *, *, #17072, .T. ) ;
#44493=DIRECTION ( 'NONE',  ( -1.000000000000000000, -0.000000000000000000, -0.000000000000000000 ) ) ;
#44499=PLANE ( 'NONE',  #40675 ) ;
#44502=LINE ( 'NONE', #8487, #12321 ) ;
#44504=DIRECTION ( 'NONE',  ( 1.000000000000000000, -0.000000000000000000, 0.000000000000000000 ) ) ;
#44505=ORIENTED_EDGE ( 'NONE', *, *, #45194, .F. ) ;
#44519=ORIENTED_EDGE ( 'NONE', *, *, #9588, .F. ) ;
#44522=DIRECTION ( 'NONE',  ( -0.000000000000000000, 0.000000000000000000, -1.000000000000000000 ) ) ;
#44526=LINE ( 'NONE', #36118, #9807 ) ;
#44527=ADVANCED_FACE ( 'NONE', ( #7911 ), #23946, .F. ) ;
#44528=DIRECTION ( 'NONE',  ( -1.000000000000000000, -0.000000000000000000, 0.000000000000000000 ) ) ;
#44530=ORIENTED_EDGE ( 'NONE', *, *, #24585, .F. ) ;
#44538=ORIENTED_EDGE ( 'NONE', *, *, #6777, .T. ) ;
#44543=EDGE_CURVE ( 'NONE', #15537, #1436, #8186, .T. ) ;
#44551=PLANE ( 'NONE',  #48746 ) ;
#44555=AXIS2_PLACEMENT_3D ( 'NONE', #42259, #37806, #34391 ) ;
#44556=ORIENTED_EDGE ( 'NONE', *, *, #2023, .F. ) ;
#44559=CARTESIAN_POINT ( 'NONE',  ( -336.3521761649654422, -106.5990858529439578, 57.57047073799066794 ) ) ;
#44560=FACE_BOUND ( 'NONE', #28643, .T. ) ;
#44562=VERTEX_POINT ( 'NONE', #40229 ) ;
#44564=DIRECTION ( 'NONE',  ( 0.000000000000000000, -0.8854560256532126861, -0.4647231720437631775 ) ) ;
#44565=ORIENTED_EDGE ( 'NONE', *, *, #7064, .T. ) ;
#44567=VECTOR ( 'NONE', #34834, 1000.000000000000000 ) ;
#44570=EDGE_CURVE ( 'NONE', #38201, #49836, #290, .T. ) ;
#44577=ORIENTED_EDGE ( 'NONE', *, *, #28252, .F. ) ;
#44581=ADVANCED_FACE ( 'NONE', ( #33652 ), #29974, .F. ) ;
#44593=FACE_OUTER_BOUND ( 'NONE', #14092, .T. ) ;
#44600=CARTESIAN_POINT ( 'NONE',  ( -339.1964088526558498, -143.9541802141663709, 55.34326076196097688 ) ) ;
#44602=VERTEX_POINT ( 'NONE', #1068 ) ;
#44607=VECTOR ( 'NONE', #33170, 1000.000000000000000 ) ;
#44610=ORIENTED_EDGE ( 'NONE', *, *, #37849, .F. ) ;
#44613=ORIENTED_EDGE ( 'NONE', *, *, #36803, .F. ) ;
#44618=LINE ( 'NONE', #25175, #44650 ) ;
#44622=VECTOR ( 'NONE', #36847, 1000.000000000000114 ) ;
#44625=DIRECTION ( 'NONE',  ( -0.000000000000000000, -0.7485107481711024136, -0.6631226582407937498 ) ) ;
#44640=CARTESIAN_POINT ( 'NONE',  ( -330.4913330509368166, -151.8251501453679850, 52.89315522109040302 ) ) ;
#44642=ORIENTED_EDGE ( 'NONE', *, *, #6449, .F. ) ;
#44643=VECTOR ( 'NONE', #18499, 1000.000000000000000 ) ;
#44645=ADVANCED_FACE ( 'NONE', ( #13948 ), #30732, .F. ) ;
#44646=ORIENTED_EDGE ( 'NONE', *, *, #44359, .T. ) ;
#44649=DIRECTION ( 'NONE',  ( -0.000000000000000000, 1.047444401652940007E-14, 1.000000000000000000 ) ) ;
#44650=VECTOR ( 'NONE', #32791, 1000.000000000000000 ) ;
#44652=FACE_OUTER_BOUND ( 'NONE', #45788, .T. ) ;
#44653=LINE ( 'NONE', #36484, #8955 ) ;
#44654=CARTESIAN_POINT ( 'NONE',  ( -332.3517673607765914, -164.5945333327934463, -42.41660376256285048 ) ) ;
#44662=FACE_OUTER_BOUND ( 'NONE', #17279, .T. ) ;
#44664=AXIS2_PLACEMENT_3D ( 'NONE', #1334, #44980, #49950 ) ;
#44668=EDGE_LOOP ( 'NONE', ( #32134, #37985, #45321, #392 ) ) ;
#44669=VERTEX_POINT ( 'NONE', #10259 ) ;
#44672=EDGE_CURVE ( 'NONE', #11150, #38873, #6835, .T. ) ;
#44682=VERTEX_POINT ( 'NONE', #3148 ) ;
#44686=CIRCLE ( 'NONE', #33798, 60.00000000000000000 ) ;
#44691=CARTESIAN_POINT ( 'NONE',  ( -339.1964088526558498, -144.8891964568526305, -54.98865587491811624 ) ) ;
#44692=DIRECTION ( 'NONE',  ( -0.000000000000000000, -0.6631226582407989678, -0.7485107481710977506 ) ) ;
#44695=DIRECTION ( 'NONE',  ( 1.043714542225393381E-14, -0.8229838658936575735, -0.5680647467311540355 ) ) ;
#44696=ORIENTED_EDGE ( 'NONE', *, *, #12004, .T. ) ;
#44700=ORIENTED_EDGE ( 'NONE', *, *, #37238, .F. ) ;
#44702=LINE ( 'NONE', #49619, #11497 ) ;
#44703=ADVANCED_FACE ( 'NONE', ( #2382 ), #18915, .T. ) ;
#44705=DIRECTION ( 'NONE',  ( -1.000000000000000000, 0.000000000000000000, 0.000000000000000000 ) ) ;
#44708=VECTOR ( 'NONE', #35226, 1000.000000000000000 ) ;
#44713=CARTESIAN_POINT ( 'NONE',  ( -305.0000000000000568, -123.5000000000000284, 0.000000000000000000 ) ) ;
#44714=PLANE ( 'NONE',  #9781 ) ;
#44716=ORIENTED_EDGE ( 'NONE', *, *, #32453, .T. ) ;
#44723=CIRCLE ( 'NONE', #31277, 60.00000000000000000 ) ;
#44729=DIRECTION ( 'NONE',  ( 0.000000000000000000, 0.000000000000000000, 1.000000000000000000 ) ) ;
#44731=EDGE_CURVE ( 'NONE', #30632, #40004, #11272, .T. ) ;
#44734=DIRECTION ( 'NONE',  ( 1.000000000000000000, -0.000000000000000000, 0.000000000000000000 ) ) ;
#44737=VECTOR ( 'NONE', #33786, 1000.000000000000114 ) ;
#44742=LINE ( 'NONE', #40000, #21266 ) ;
#44748=PLANE ( 'NONE',  #28307 ) ;
#44751=VECTOR ( 'NONE', #15149, 999.9999999999998863 ) ;
#44752=VERTEX_POINT ( 'NONE', #14216 ) ;
#44753=EDGE_CURVE ( 'NONE', #6309, #28688, #50475, .T. ) ;
#44757=ORIENTED_EDGE ( 'NONE', *, *, #23754, .T. ) ;
#44761=ORIENTED_EDGE ( 'NONE', *, *, #19564, .T. ) ;
#44762=FACE_OUTER_BOUND ( 'NONE', #31465, .T. ) ;
#44764=ADVANCED_FACE ( 'NONE', ( #38371 ), #26796, .F. ) ;
#44766=CARTESIAN_POINT ( 'NONE',  ( -330.4913330509368166, -175.9742670995615015, -26.97593913775547136 ) ) ;
#44779=ORIENTED_EDGE ( 'NONE', *, *, #44439, .F. ) ;
#44781=DIRECTION ( 'NONE',  ( 1.000000000000000000, -0.000000000000000000, -0.000000000000000000 ) ) ;
#44784=ORIENTED_EDGE ( 'NONE', *, *, #30759, .F. ) ;
#44787=ORIENTED_EDGE ( 'NONE', *, *, #3640, .T. ) ;
#44790=LINE ( 'NONE', #41883, #38980 ) ;
#44793=ORIENTED_EDGE ( 'NONE', *, *, #7905, .T. ) ;
#44797=VERTEX_POINT ( 'NONE', #19180 ) ;
#44798=VECTOR ( 'NONE', #30660, 1000.000000000000000 ) ;
#44799=CARTESIAN_POINT ( 'NONE',  ( -330.4913330509368166, -151.3613951634084742, 52.00954392751779665 ) ) ;
#44802=ORIENTED_EDGE ( 'NONE', *, *, #3513, .F. ) ;
#44804=CARTESIAN_POINT ( 'NONE',  ( -339.1964088526558498, -70.14212160686578557, 27.43969411971455585 ) ) ;
#44807=VERTEX_POINT ( 'NONE', #51764 ) ;
#44808=DIRECTION ( 'NONE',  ( 0.000000000000000000, 0.000000000000000000, -1.000000000000000000 ) ) ;
#44810=VECTOR ( 'NONE', #8394, 999.9999999999998863 ) ;
#44813=CARTESIAN_POINT ( 'NONE',  ( -365.0000000000001137, -168.5000000000000284, 0.000000000000000000 ) ) ;
#44814=ORIENTED_EDGE ( 'NONE', *, *, #10464, .T. ) ;
#44815=ORIENTED_EDGE ( 'NONE', *, *, #15225, .F. ) ;
#44821=FACE_BOUND ( 'NONE', #41045, .T. ) ;
#44822=FACE_OUTER_BOUND ( 'NONE', #32351, .T. ) ;
#44827=ORIENTED_EDGE ( 'NONE', *, *, #1573, .F. ) ;
#44828=DIRECTION ( 'NONE',  ( 0.000000000000000000, -0.5680647467311457088, 0.8229838658936633466 ) ) ;
#44829=VERTEX_POINT ( 'NONE', #15778 ) ;
#44830=EDGE_LOOP ( 'NONE', ( #25603, #14857, #31880, #1026 ) ) ;
#44836=DIRECTION ( 'NONE',  ( 1.000000000000000000, 0.000000000000000000, 8.718379230999705894E-17 ) ) ;
#44839=EDGE_LOOP ( 'NONE', ( #50007, #33992 ) ) ;
#44842=LINE ( 'NONE', #45378, #14400 ) ;
#44847=DIRECTION ( 'NONE',  ( -1.000000000000000000, -0.000000000000000000, -0.000000000000000000 ) ) ;
#44848=CARTESIAN_POINT ( 'NONE',  ( -330.4913330509368166, -172.3400804610910200, 33.10432812419180948 ) ) ;
#44851=PLANE ( 'NONE',  #5395 ) ;
#44854=CARTESIAN_POINT ( 'NONE',  ( -336.3521761649654422, -107.7955183043589500, 56.89493493766750731 ) ) ;
#44857=DIRECTION ( 'NONE',  ( 1.000000000000000000, -0.000000000000000000, -0.000000000000000000 ) ) ;
#44859=CARTESIAN_POINT ( 'NONE',  ( 0.000000000000000000, -130.6116641350643022, -58.56982357178517873 ) ) ;
#44860=ORIENTED_EDGE ( 'NONE', *, *, #32356, .F. ) ;
#44861=CARTESIAN_POINT ( 'NONE',  ( -332.3517673607765914, -149.4733471526596134, 53.00046796564699036 ) ) ;
#44866=CARTESIAN_POINT ( 'NONE',  ( -336.3521761649654422, -155.6724726690323450, 49.48329383994676078 ) ) ;
#44867=LINE ( 'NONE', #9643, #38849 ) ;
#44869=EDGE_CURVE ( 'NONE', #11668, #25203, #47823, .T. ) ;
#44872=CARTESIAN_POINT ( 'NONE',  ( -330.4913330509368166, -137.1341532842523918, 57.40522506028099770 ) ) ;
#44879=CARTESIAN_POINT ( 'NONE',  ( -305.0000000000000568, -96.06030588028460215, -53.35787839313380232 ) ) ;
#44883=LINE ( 'NONE', #13348, #45661 ) ;
#44885=EDGE_CURVE ( 'NONE', #44797, #27513, #3927, .T. ) ;
#44887=EDGE_CURVE ( 'NONE', #8253, #18899, #48605, .T. ) ;
#44890=EDGE_LOOP ( 'NONE', ( #25556, #49554, #10962, #37483 ) ) ;
#44895=EDGE_CURVE ( 'NONE', #42517, #6623, #35985, .T. ) ;
#44896=AXIS2_PLACEMENT_3D ( 'NONE', #23867, #48589, #12566 ) ;
#44898=ORIENTED_EDGE ( 'NONE', *, *, #3814, .T. ) ;
#44901=EDGE_CURVE ( 'NONE', #26369, #13489, #40422, .T. ) ;
#44904=ORIENTED_EDGE ( 'NONE', *, *, #32353, .T. ) ;
#44905=DIRECTION ( 'NONE',  ( 1.000000000000000000, -0.000000000000000000, -0.000000000000000000 ) ) ;
#44907=EDGE_LOOP ( 'NONE', ( #50337, #26624, #16070, #10609 ) ) ;
#44911=PLANE ( 'NONE',  #27198 ) ;
#44917=CARTESIAN_POINT ( 'NONE',  ( -330.4913330509368166, -151.3613951634091848, -52.00954392751743427 ) ) ;
#44920=PLANE ( 'NONE',  #35506 ) ;
#44921=ORIENTED_EDGE ( 'NONE', *, *, #51905, .F. ) ;
#44924=AXIS2_PLACEMENT_3D ( 'NONE', #34921, #11008, #27037 ) ;
#44928=ORIENTED_EDGE ( 'NONE', *, *, #48739, .F. ) ;
#44930=VERTEX_POINT ( 'NONE', #4443 ) ;
#44931=AXIS2_PLACEMENT_3D ( 'NONE', #19075, #22510, #38523 ) ;
#44933=DIRECTION ( 'NONE',  ( 0.000000000000000000, -0.8229838658936613482, -0.5680647467311485954 ) ) ;
#44935=VECTOR ( 'NONE', #4618, 1000.000000000000000 ) ;
#44936=CARTESIAN_POINT ( 'NONE',  ( -339.1964088526558498, -95.63860483659122735, -52.00954392751761191 ) ) ;
#44941=EDGE_CURVE ( 'NONE', #37560, #45837, #13100, .T. ) ;
#44942=EDGE_CURVE ( 'NONE', #48882, #30259, #33071, .T. ) ;
#44948=EDGE_CURVE ( 'NONE', #36522, #5943, #4700, .T. ) ;
#44949=CARTESIAN_POINT ( 'NONE',  ( -336.3521761649654422, -123.5000000000000284, 0.000000000000000000 ) ) ;
#44952=CARTESIAN_POINT ( 'NONE',  ( -336.3521761649654422, -86.34605966037949543, -45.90766452162698386 ) ) ;
#44953=ORIENTED_EDGE ( 'NONE', *, *, #18375, .F. ) ;
#44960=LINE ( 'NONE', #48648, #31943 ) ;
#44961=CARTESIAN_POINT ( 'NONE',  ( -330.4913330509368166, -75.22798428563942252, 33.92731199008440512 ) ) ;
#44962=LINE ( 'NONE', #32851, #19089 ) ;
#44963=ORIENTED_EDGE ( 'NONE', *, *, #23976, .F. ) ;
#44965=ADVANCED_FACE ( 'NONE', ( #21254 ), #17828, .T. ) ;
#44967=AXIS2_PLACEMENT_3D ( 'NONE', #16916, #40029, #4053 ) ;
#44971=EDGE_LOOP ( 'NONE', ( #44276, #24928, #14045, #22311 ) ) ;
#44975=LINE ( 'NONE', #5550, #19913 ) ;
#44978=EDGE_CURVE ( 'NONE', #34020, #5922, #17846, .T. ) ;
#44980=DIRECTION ( 'NONE',  ( 1.043714542225393539E-14, -0.9709418174260527890, -0.2393156642875547968 ) ) ;
#44983=VECTOR ( 'NONE', #40874, 1000.000000000000000 ) ;
#44985=CARTESIAN_POINT ( 'NONE',  ( -339.1964088526558498, -66.33409060400673241, -14.60509510167901404 ) ) ;
#44986=DIRECTION ( 'NONE',  ( -1.000000000000000000, 9.241633304753606050E-15, 4.850383327711861546E-15 ) ) ;
#44992=EDGE_CURVE ( 'NONE', #5970, #37898, #1009, .T. ) ;
#44993=VECTOR ( 'NONE', #45417, 1000.000000000000114 ) ;
#45001=CARTESIAN_POINT ( 'NONE',  ( -339.1964088526558498, -180.9052250602809977, -13.63415328425247885 ) ) ;
#45002=CIRCLE ( 'NONE', #11396, 60.00000000000000000 ) ;
#45003=CIRCLE ( 'NONE', #20680, 60.00000000000000000 ) ;
#45006=PLANE ( 'NONE',  #36227 ) ;
#45009=AXIS2_PLACEMENT_3D ( 'NONE', #28616, #16561, #8655 ) ;
#45010=ORIENTED_EDGE ( 'NONE', *, *, #25886, .F. ) ;
#45012=EDGE_CURVE ( 'NONE', #7333, #29626, #49117, .T. ) ;
#45014=FACE_OUTER_BOUND ( 'NONE', #11999, .T. ) ;
#45015=EDGE_LOOP ( 'NONE', ( #50264, #35153, #44031, #36218 ) ) ;
#45022=LINE ( 'NONE', #9013, #44607 ) ;
#45025=VERTEX_POINT ( 'NONE', #38042 ) ;
#45030=VERTEX_POINT ( 'NONE', #34110 ) ;
#45033=VERTEX_POINT ( 'NONE', #23059 ) ;
#45040=EDGE_LOOP ( 'NONE', ( #50916, #358, #44079, #26316 ) ) ;
#45043=DIRECTION ( 'NONE',  ( 1.000000000000000000, 0.000000000000000000, 0.000000000000000000 ) ) ;
#45045=CARTESIAN_POINT ( 'NONE',  ( 0.000000000000000000, -162.6242368362071602, -44.16213414209478572 ) ) ;
#45052=CARTESIAN_POINT ( 'NONE',  ( -305.0000000000000568, -123.0000000000002700, -59.99791663049643375 ) ) ;
#45054=DIRECTION ( 'NONE',  ( 0.000000000000000000, -0.4647231720437789981, -0.8854560256532044704 ) ) ;
#45058=DIRECTION ( 'NONE',  ( 0.000000000000000000, 1.000000000000000000, 0.000000000000000000 ) ) ;
#45062=VECTOR ( 'NONE', #21973, 1000.000000000000000 ) ;
#45064=FACE_OUTER_BOUND ( 'NONE', #48778, .T. ) ;
#45079=ADVANCED_FACE ( 'NONE', ( #50928 ), #35140, .F. ) ;
#45080=DIRECTION ( 'NONE',  ( 0.000000000000000000, 0.000000000000000000, 1.000000000000000000 ) ) ;
#45082=VECTOR ( 'NONE', #19574, 1000.000000000000000 ) ;
#45088=DIRECTION ( 'NONE',  ( 0.000000000000000000, 0.3546048870425463906, 0.9350162426854107256 ) ) ;
#45090=LINE ( 'NONE', #37181, #34474 ) ;
#45091=DIRECTION ( 'NONE',  ( 0.000000000000000000, 0.000000000000000000, -1.000000000000000000 ) ) ;
#45092=VERTEX_POINT ( 'NONE', #10444 ) ;
#45096=DIRECTION ( 'NONE',  ( 0.000000000000000000, -0.2393156642875482742, 0.9709418174260544543 ) ) ;
#45100=DIRECTION ( 'NONE',  ( -0.000000000000000000, -0.9927088740980548609, -0.1205366802553164696 ) ) ;
#45102=FACE_BOUND ( 'NONE', #7875, .T. ) ;
#45105=ORIENTED_EDGE ( 'NONE', *, *, #30815, .T. ) ;
#45106=ORIENTED_EDGE ( 'NONE', *, *, #41954, .T. ) ;
#45109=VERTEX_POINT ( 'NONE', #50413 ) ;
#45110=DIRECTION ( 'NONE',  ( -1.000000000000000000, 0.000000000000000000, 0.000000000000000000 ) ) ;
#45111=CARTESIAN_POINT ( 'NONE',  ( -336.3521761649654422, -136.0347666902908372, 57.67619951860663718 ) ) ;
#45113=CARTESIAN_POINT ( 'NONE',  ( -339.1964088526558498, -68.15673923803898049, 20.45418021416614351 ) ) ;
#45118=ORIENTED_EDGE ( 'NONE', *, *, #43094, .F. ) ;
#45119=CARTESIAN_POINT ( 'NONE',  ( -336.3521761649654422, -92.15051119686104641, -50.05135858667769355 ) ) ;
#45122=CARTESIAN_POINT ( 'NONE',  ( -339.1964088526558498, -71.02573290043878274, -26.97593913775585506 ) ) ;
#45123=AXIS2_PLACEMENT_3D ( 'NONE', #36136, #24065, #28505 ) ;
#45126=LINE ( 'NONE', #9371, #35569 ) ;
#45130=DIRECTION ( 'NONE',  ( 0.000000000000000000, -1.091719307548070640E-13, 1.000000000000000000 ) ) ;
#45131=EDGE_CURVE ( 'NONE', #5355, #20985, #22039, .T. ) ;
#45132=LINE ( 'NONE', #9121, #7666 ) ;
#45134=ORIENTED_EDGE ( 'NONE', *, *, #20858, .T. ) ;
#45136=AXIS2_PLACEMENT_3D ( 'NONE', #30218, #21565, #9728 ) ;
#45137=CARTESIAN_POINT ( 'NONE',  ( -336.3521761649654422, -93.31268025388605736, 51.85292399224829296 ) ) ;
#45138=ORIENTED_EDGE ( 'NONE', *, *, #30325, .F. ) ;
#45139=AXIS2_PLACEMENT_3D ( 'NONE', #25130, #33262, #41401 ) ;
#45155=ORIENTED_EDGE ( 'NONE', *, *, #44039, .T. ) ;
#45158=VECTOR ( 'NONE', #39273, 1000.000000000000000 ) ;
#45162=EDGE_CURVE ( 'NONE', #4141, #48781, #22021, .T. ) ;
#45168=PLANE ( 'NONE',  #1595 ) ;
#45169=CARTESIAN_POINT ( 'NONE',  ( 0.000000000000000000, -182.0698235717851787, 7.111664135064491354 ) ) ;
#45170=ORIENTED_EDGE ( 'NONE', *, *, #26937, .F. ) ;
#45174=VECTOR ( 'NONE', #50059, 1000.000000000000000 ) ;
#45187=CARTESIAN_POINT ( 'NONE',  ( -305.0000000000000568, -66.84097189748108292, 19.74220186498881091 ) ) ;
#45192=CARTESIAN_POINT ( 'NONE',  ( -339.1964088526558498, -123.5000000000000284, 0.000000000000000000 ) ) ;
#45194=EDGE_CURVE ( 'NONE', #7784, #5668, #26210, .T. ) ;
#45198=DIRECTION ( 'NONE',  ( 0.000000000000000000, 0.2393156642875548246, -0.9709418174260527890 ) ) ;
#45203=AXIS2_PLACEMENT_3D ( 'NONE', #40611, #24100, #40110 ) ;
#45206=CARTESIAN_POINT ( 'NONE',  ( -330.4913330509368166, -79.00630452878473875, -38.74998146212148953 ) ) ;
#45208=ORIENTED_EDGE ( 'NONE', *, *, #49129, .T. ) ;
#45209=LINE ( 'NONE', #37293, #36313 ) ;
#45220=DIRECTION ( 'NONE',  ( 0.000000000000000000, 1.794860556477336491E-13, -1.000000000000000000 ) ) ;
#45230=LINE ( 'NONE', #37319, #4049 ) ;
#45231=CARTESIAN_POINT ( 'NONE',  ( -330.4913330509368166, -175.5095439275173419, 27.86139516340933042 ) ) ;
#45233=AXIS2_PLACEMENT_3D ( 'NONE', #8250, #3788, #19814 ) ;
#45235=DIRECTION ( 'NONE',  ( 0.000000000000000000, -0.9350162426854146114, 0.3546048870425363986 ) ) ;
#45237=LINE ( 'NONE', #21830, #31440 ) ;
#45238=LINE ( 'NONE', #28911, #26644 ) ;
#45241=CARTESIAN_POINT ( 'NONE',  ( -330.4913330509368166, -84.75001853787871653, -44.49369547121542467 ) ) ;
#45242=CARTESIAN_POINT ( 'NONE',  ( -339.1964088526558498, -130.2355952558260412, 59.62073260661674823 ) ) ;
#45244=ORIENTED_EDGE ( 'NONE', *, *, #10672, .F. ) ;
#45254=DIRECTION ( 'NONE',  ( 0.000000000000000000, 0.000000000000000000, 1.000000000000000000 ) ) ;
#45259=CARTESIAN_POINT ( 'NONE',  ( -332.3517673607765914, -123.5000000000000284, 0.000000000000000000 ) ) ;
#45260=DIRECTION ( 'NONE',  ( 0.000000000000000000, -1.850371707708594366E-15, -1.000000000000000000 ) ) ;
#45261=EDGE_CURVE ( 'NONE', #33448, #7384, #19628, .T. ) ;
#45265=CARTESIAN_POINT ( 'NONE',  ( 0.000000000000000000, -102.5783116644905562, -55.16595831843955722 ) ) ;
#45274=LINE ( 'NONE', #48683, #34562 ) ;
#45276=CARTESIAN_POINT ( 'NONE',  ( -339.1964088526558498, -71.49045607248255862, -27.86139516340906397 ) ) ;
#45284=CARTESIAN_POINT ( 'NONE',  ( -336.3521761649654422, -82.40546666720629787, 42.41660376256258047 ) ) ;
#45285=ORIENTED_EDGE ( 'NONE', *, *, #13814, .T. ) ;
#45292=EDGE_CURVE ( 'NONE', #41684, #30672, #43798, .T. ) ;
#45294=DIRECTION ( 'NONE',  ( 0.000000000000000000, 1.191176786837407622E-13, 1.000000000000000000 ) ) ;
#45295=FACE_OUTER_BOUND ( 'NONE', #42210, .T. ) ;
#45298=ORIENTED_EDGE ( 'NONE', *, *, #28332, .T. ) ;
#45300=ORIENTED_EDGE ( 'NONE', *, *, #11281, .T. ) ;
#45301=FACE_OUTER_BOUND ( 'NONE', #22915, .T. ) ;
#45303=DIRECTION ( 'NONE',  ( -0.000000000000000000, 0.000000000000000000, 1.000000000000000000 ) ) ;
#45307=FACE_OUTER_BOUND ( 'NONE', #11919, .T. ) ;
#45314=EDGE_LOOP ( 'NONE', ( #32343, #7114, #18187, #50942 ) ) ;
#45321=ORIENTED_EDGE ( 'NONE', *, *, #286, .F. ) ;
#45322=DIRECTION ( 'NONE',  ( 1.000000000000000000, 1.050884489711603377E-17, -8.654812430365582767E-17 ) ) ;
#45325=DIRECTION ( 'NONE',  ( 1.000000000000000000, 0.000000000000000000, 0.000000000000000000 ) ) ;
#45328=CARTESIAN_POINT ( 'NONE',  ( -332.3517673607765914, -172.9832938399466684, -32.17247266903247294 ) ) ;
#45338=ORIENTED_EDGE ( 'NONE', *, *, #24055, .F. ) ;
#45339=DIRECTION ( 'NONE',  ( 1.000000000000000000, -0.000000000000000000, -0.000000000000000000 ) ) ;
#45341=DIRECTION ( 'NONE',  ( -1.000000000000000000, 0.000000000000000000, -0.000000000000000000 ) ) ;
#45346=DIRECTION ( 'NONE',  ( 1.000000000000000000, 0.000000000000000000, 0.000000000000000000 ) ) ;
#45348=FACE_OUTER_BOUND ( 'NONE', #14083, .T. ) ;
#45353=CARTESIAN_POINT ( 'NONE',  ( -330.4913330509368166, -90.39567187580871632, -48.84008046109136814 ) ) ;
#45361=ORIENTED_EDGE ( 'NONE', *, *, #5775, .F. ) ;
#45362=CARTESIAN_POINT ( 'NONE',  ( -336.3521761649654422, -66.84438072661991725, -16.67542351306652648 ) ) ;
#45363=VERTEX_POINT ( 'NONE', #13305 ) ;
#45368=DIRECTION ( 'NONE',  ( 1.000000000000000000, 0.000000000000000000, 0.000000000000000000 ) ) ;
#45370=ADVANCED_FACE ( 'NONE', ( #49048 ), #45376, .F. ) ;
#45372=ORIENTED_EDGE ( 'NONE', *, *, #42570, .T. ) ;
#45374=ORIENTED_EDGE ( 'NONE', *, *, #42439, .T. ) ;
#45375=ORIENTED_EDGE ( 'NONE', *, *, #42813, .F. ) ;
#45376=PLANE ( 'NONE',  #26226 ) ;
#45377=CIRCLE ( 'NONE', #15992, 60.00000000000000000 ) ;
#45378=CARTESIAN_POINT ( 'NONE',  ( -330.4913330509368166, -64.86990808808705822, 6.615309698014281814 ) ) ;
#45380=DIRECTION ( 'NONE',  ( -0.000000000000000000, 0.8229838658936575735, 0.5680647467311540355 ) ) ;
#45382=FACE_OUTER_BOUND ( 'NONE', #23529, .T. ) ;
#45384=PLANE ( 'NONE',  #23204 ) ;
#45385=FACE_OUTER_BOUND ( 'NONE', #26518, .T. ) ;
#45390=EDGE_LOOP ( 'NONE', ( #3614, #45946, #28458, #18308 ) ) ;
#45394=ORIENTED_EDGE ( 'NONE', *, *, #42456, .T. ) ;
#45396=EDGE_CURVE ( 'NONE', #6991, #8561, #24868, .T. ) ;
#45398=LINE ( 'NONE', #2005, #36888 ) ;
#45399=DIRECTION ( 'NONE',  ( 0.000000000000000000, 0.000000000000000000, 1.000000000000000000 ) ) ;
#45400=CARTESIAN_POINT ( 'NONE',  ( -330.4913330509368166, -64.99044476834247064, -7.608018572113060429 ) ) ;
#45402=ADVANCED_FACE ( 'NONE', ( #37472 ), #21187, .F. ) ;
#45405=ORIENTED_EDGE ( 'NONE', *, *, #19267, .F. ) ;
#45414=VERTEX_POINT ( 'NONE', #21445 ) ;
#45415=EDGE_CURVE ( 'NONE', #23609, #31967, #18703, .T. ) ;
#45417=DIRECTION ( 'NONE',  ( -0.000000000000000000, -0.7485107481710953081, 0.6631226582408016323 ) ) ;
#45420=VERTEX_POINT ( 'NONE', #36958 ) ;
#45421=ORIENTED_EDGE ( 'NONE', *, *, #45845, .T. ) ;
#45423=CARTESIAN_POINT ( 'NONE',  ( -332.3517673607765914, -182.3871109312487420, -4.498567634386014369 ) ) ;
#45429=ORIENTED_EDGE ( 'NONE', *, *, #18289, .F. ) ;
#45436=FACE_OUTER_BOUND ( 'NONE', #43759, .T. ) ;
#45444=PLANE ( 'NONE',  #22983 ) ;
#45445=CARTESIAN_POINT ( 'NONE',  ( -332.3517673607765914, -81.08339623743702873, -41.09453333279329712 ) ) ;
#45447=DIRECTION ( 'NONE',  ( 0.000000000000000000, 0.000000000000000000, 1.000000000000000000 ) ) ;
#45448=CARTESIAN_POINT ( 'NONE',  ( -336.3521761649654422, -72.48138011061176655, -29.74944317415788930 ) ) ;
#45451=EDGE_CURVE ( 'NONE', #13962, #6134, #33539, .T. ) ;
#45453=FACE_OUTER_BOUND ( 'NONE', #38373, .T. ) ;
#45454=ORIENTED_EDGE ( 'NONE', *, *, #47561, .F. ) ;
#45463=VECTOR ( 'NONE', #15130, 999.9999999999998863 ) ;
#45466=VECTOR ( 'NONE', #27848, 1000.000000000000000 ) ;
#45467=CARTESIAN_POINT ( 'NONE',  ( -365.0000000000001137, -168.5000000000000284, 0.000000000000000000 ) ) ;
#45470=ORIENTED_EDGE ( 'NONE', *, *, #13002, .T. ) ;
#45472=EDGE_CURVE ( 'NONE', #30320, #1001, #29325, .T. ) ;
#45474=EDGE_CURVE ( 'NONE', #6061, #13689, #49576, .T. ) ;
#45476=FACE_OUTER_BOUND ( 'NONE', #39662, .T. ) ;
#45483=DIRECTION ( 'NONE',  ( 0.000000000000000000, 0.000000000000000000, 1.000000000000000000 ) ) ;
#45488=CARTESIAN_POINT ( 'NONE',  ( -339.1964088526558498, -68.51134412508183402, -21.38919645685240312 ) ) ;
#45494=DIRECTION ( 'NONE',  ( -0.000000000000000000, -0.1205366802553130001, 0.9927088740980551940 ) ) ;
#45498=ORIENTED_EDGE ( 'NONE', *, *, #40718, .F. ) ;
#45501=DIRECTION ( 'NONE',  ( 0.000000000000000000, 0.000000000000000000, -1.000000000000000000 ) ) ;
#45503=DIRECTION ( 'NONE',  ( 1.000000000000000000, -0.000000000000000000, -0.000000000000000000 ) ) ;
#45513=PLANE ( 'NONE',  #30262 ) ;
#45515=VECTOR ( 'NONE', #34265, 1000.000000000000000 ) ;
#45517=VECTOR ( 'NONE', #38050, 1000.000000000000000 ) ;
#45519=PLANE ( 'NONE',  #11899 ) ;
#45523=ORIENTED_EDGE ( 'NONE', *, *, #42350, .F. ) ;
#45535=DIRECTION ( 'NONE',  ( 0.000000000000000000, 1.989149585786738886E-13, -1.000000000000000000 ) ) ;
#45536=ORIENTED_EDGE ( 'NONE', *, *, #18191, .T. ) ;
#45540=CARTESIAN_POINT ( 'NONE',  ( -336.3521761649654422, -133.3383340306578759, -59.18789727217212970 ) ) ;
#45542=EDGE_CURVE ( 'NONE', #9916, #27018, #23719, .T. ) ;
#45545=VERTEX_POINT ( 'NONE', #46154 ) ;
#45546=LINE ( 'NONE', #17943, #40617 ) ;
#45547=ORIENTED_EDGE ( 'NONE', *, *, #4403, .T. ) ;
#45551=PLANE ( 'NONE',  #34945 ) ;
#45554=ADVANCED_FACE ( 'NONE', ( #34049 ), #34308, .F. ) ;
#45559=FACE_OUTER_BOUND ( 'NONE', #10348, .T. ) ;
#45564=EDGE_CURVE ( 'NONE', #49548, #51496, #18538, .T. ) ;
#45575=VECTOR ( 'NONE', #30354, 1000.000000000000114 ) ;
#45585=ORIENTED_EDGE ( 'NONE', *, *, #42175, .T. ) ;
#45586=DIRECTION ( 'NONE',  ( 0.000000000000000000, -0.5680647467311596976, -0.8229838658936536877 ) ) ;
#45587=CARTESIAN_POINT ( 'NONE',  ( -305.0000000000000568, -137.3729703655834840, 58.37414404713479854 ) ) ;
#45588=EDGE_LOOP ( 'NONE', ( #20296, #34164, #17010, #48855 ) ) ;
#45593=EDGE_CURVE ( 'NONE', #30158, #32832, #17769, .T. ) ;
#45611=DIRECTION ( 'NONE',  ( 0.000000000000000000, -0.6631226582407885317, 0.7485107481711069655 ) ) ;
#45612=LINE ( 'NONE', #17751, #12552 ) ;
#45613=DIRECTION ( 'NONE',  ( 0.000000000000000000, -0.7485107481711069655, -0.6631226582407885317 ) ) ;
#45614=PLANE ( 'NONE',  #25537 ) ;
#45619=ORIENTED_EDGE ( 'NONE', *, *, #24780, .F. ) ;
#45624=PLANE ( 'NONE',  #16568 ) ;
#45625=LINE ( 'NONE', #30094, #4007 ) ;
#45627=CARTESIAN_POINT ( 'NONE',  ( -330.4913330509368166, -123.5000000000000284, 0.000000000000000000 ) ) ;
#45631=VECTOR ( 'NONE', #31567, 1000.000000000000000 ) ;
#45632=ORIENTED_EDGE ( 'NONE', *, *, #18120, .F. ) ;
#45634=EDGE_LOOP ( 'NONE', ( #49385, #21796, #35814, #33463 ) ) ;
#45635=CARTESIAN_POINT ( 'NONE',  ( -336.3521761649654422, -72.01665693856799066, -28.86398714850468039 ) ) ;
#45638=VERTEX_POINT ( 'NONE', #12184 ) ;
#45641=PLANE ( 'NONE',  #1913 ) ;
#45642=CARTESIAN_POINT ( 'NONE',  ( -339.1964088526558498, -182.1300919119129560, -6.615309698014600670 ) ) ;
#45644=PLANE ( 'NONE',  #35349 ) ;
#45646=EDGE_LOOP ( 'NONE', ( #22152, #197, #7164, #16375 ) ) ;
#45659=EDGE_CURVE ( 'NONE', #18186, #33549, #51490, .T. ) ;
#45661=VECTOR ( 'NONE', #13862, 1000.000000000000227 ) ;
#45662=ORIENTED_EDGE ( 'NONE', *, *, #32495, .T. ) ;
#45671=DIRECTION ( 'NONE',  ( 0.000000000000000000, 0.5680647467311658039, 0.8229838658936494689 ) ) ;
#45677=ADVANCED_FACE ( 'NONE', ( #31134 ), #47948, .F. ) ;
#45679=DIRECTION ( 'NONE',  ( -1.000000000000000000, 0.000000000000000000, 0.000000000000000000 ) ) ;
#45680=CARTESIAN_POINT ( 'NONE',  ( 0.000000000000000000, -109.3803758070334737, 57.28556722813694080 ) ) ;
#45682=ORIENTED_EDGE ( 'NONE', *, *, #26231, .T. ) ;
#45690=EDGE_CURVE ( 'NONE', #43387, #16147, #33023, .T. ) ;
#45694=CARTESIAN_POINT ( 'NONE',  ( -336.3521761649653854, -63.52220716707010695, -1.632288850093980725 ) ) ;
#45696=ORIENTED_EDGE ( 'NONE', *, *, #45261, .T. ) ;
#45702=ORIENTED_EDGE ( 'NONE', *, *, #48310, .T. ) ;
#45704=PLANE ( 'NONE',  #16259 ) ;
#45705=DIRECTION ( 'NONE',  ( -0.000000000000000000, -0.2393156642875615969, -0.9709418174260511236 ) ) ;
#45706=LINE ( 'NONE', #18365, #40826 ) ;
#45708=EDGE_LOOP ( 'NONE', ( #8669, #23161, #33475, #13642 ) ) ;
#45713=VERTEX_POINT ( 'NONE', #47700 ) ;
#45715=CARTESIAN_POINT ( 'NONE',  ( -332.3517673607765914, -181.1761995186066088, -12.53476669029101842 ) ) ;
#45719=PLANE ( 'NONE',  #16573 ) ;
#45722=EDGE_LOOP ( 'NONE', ( #19610, #34325, #39486, #29969 ) ) ;
#45723=AXIS2_PLACEMENT_3D ( 'NONE', #48218, #32437, #4321 ) ;
#45731=CARTESIAN_POINT ( 'NONE',  ( -330.4913330509368166, -123.5000000000000284, 0.000000000000000000 ) ) ;
#45732=CARTESIAN_POINT ( 'NONE',  ( -336.3521761649654422, -165.9166037625627439, 41.09453333279358134 ) ) ;
#45733=ORIENTED_EDGE ( 'NONE', *, *, #35816, .F. ) ;
#45735=PLANE ( 'NONE',  #21407 ) ;
#45740=DIRECTION ( 'NONE',  ( -1.000000000000000000, 0.000000000000000000, 0.000000000000000000 ) ) ;
#45744=DIRECTION ( 'NONE',  ( 1.000000000000000000, 0.000000000000000000, 0.000000000000000000 ) ) ;
#45745=ORIENTED_EDGE ( 'NONE', *, *, #10889, .T. ) ;
#45749=AXIS2_PLACEMENT_3D ( 'NONE', #21255, #36481, #50163 ) ;
#45750=CARTESIAN_POINT ( 'NONE',  ( -330.4913330509368166, -123.5000000000000284, 0.000000000000000000 ) ) ;
#45751=VERTEX_POINT ( 'NONE', #3533 ) ;
#45753=DIRECTION ( 'NONE',  ( -1.000000000000000000, -0.000000000000000000, 0.000000000000000000 ) ) ;
#45757=VECTOR ( 'NONE', #23572, 999.9999999999998863 ) ;
#45760=LINE ( 'NONE', #29983, #5323 ) ;
#45764=ORIENTED_EDGE ( 'NONE', *, *, #24072, .F. ) ;
#45765=DIRECTION ( 'NONE',  ( -0.000000000000000000, -0.9709418174260534551, -0.2393156642875516327 ) ) ;
#45769=EDGE_CURVE ( 'NONE', #45837, #3041, #47295, .T. ) ;
#45770=VECTOR ( 'NONE', #38088, 1000.000000000000000 ) ;
#45771=DIRECTION ( 'NONE',  ( 0.000000000000000000, -0.5680647467311457088, 0.8229838658936634577 ) ) ;
#45772=ADVANCED_FACE ( 'NONE', ( #15635 ), #7995, .F. ) ;
#45781=EDGE_CURVE ( 'NONE', #37883, #37128, #45760, .T. ) ;
#45782=DIRECTION ( 'NONE',  ( -1.000000000000000000, -0.000000000000000000, 0.000000000000000000 ) ) ;
#45783=PLANE ( 'NONE',  #51372 ) ;
#45785=ORIENTED_EDGE ( 'NONE', *, *, #41082, .F. ) ;
#45787=AXIS2_PLACEMENT_3D ( 'NONE', #20274, #48671, #31851 ) ;
#45788=EDGE_LOOP ( 'NONE', ( #13399, #4884, #7956, #10984 ) ) ;
#45789=DIRECTION ( 'NONE',  ( 1.000000000000000000, -0.000000000000000000, -0.000000000000000000 ) ) ;
#45791=AXIS2_PLACEMENT_3D ( 'NONE', #47373, #6663, #6909 ) ;
#45792=DIRECTION ( 'NONE',  ( 1.000000000000000000, 0.000000000000000000, -0.000000000000000000 ) ) ;
#45795=DIRECTION ( 'NONE',  ( 0.000000000000000000, -0.5680647467311625842, -0.8229838658936516893 ) ) ;
#45802=EDGE_LOOP ( 'NONE', ( #30582, #95, #26924, #1054 ) ) ;
#45807=DIRECTION ( 'NONE',  ( -1.000000000000000000, 0.000000000000000000, 0.000000000000000000 ) ) ;
#45813=CARTESIAN_POINT ( 'NONE',  ( -339.1964088526558498, -79.00630452878473875, -38.74998146212148953 ) ) ;
#45815=LINE ( 'NONE', #17708, #13983 ) ;
#45816=ORIENTED_EDGE ( 'NONE', *, *, #24239, .T. ) ;
#45817=CARTESIAN_POINT ( 'NONE',  ( -170.0000000000000284, -123.5000000000000284, 0.000000000000000000 ) ) ;
#45818=DIRECTION ( 'NONE',  ( -1.000000000000000000, 0.000000000000000000, 0.000000000000000000 ) ) ;
#45819=ORIENTED_EDGE ( 'NONE', *, *, #23915, .T. ) ;
#45820=DIRECTION ( 'NONE',  ( 0.000000000000000000, 0.000000000000000000, -1.000000000000000000 ) ) ;
#45824=CARTESIAN_POINT ( 'NONE',  ( -305.0000000000000568, -157.9941932480467415, -49.09328500076569668 ) ) ;
#45826=ORIENTED_EDGE ( 'NONE', *, *, #13979, .T. ) ;
#45830=EDGE_CURVE ( 'NONE', #45025, #42517, #39676, .T. ) ;
#45831=DIRECTION ( 'NONE',  ( -1.000000000000000000, 0.000000000000000000, 0.000000000000000000 ) ) ;
#45833=EDGE_CURVE ( 'NONE', #15690, #15571, #2115, .T. ) ;
#45837=VERTEX_POINT ( 'NONE', #33915 ) ;
#45838=VECTOR ( 'NONE', #38226, 1000.000000000000000 ) ;
#45841=ORIENTED_EDGE ( 'NONE', *, *, #46629, .F. ) ;
#45842=EDGE_CURVE ( 'NONE', #33208, #3383, #50234, .T. ) ;
#45845=EDGE_CURVE ( 'NONE', #34872, #37919, #21592, .T. ) ;
#45852=FACE_OUTER_BOUND ( 'NONE', #9663, .T. ) ;
#45855=CARTESIAN_POINT ( 'NONE',  ( -339.1964088526558498, -90.39567187580880159, -48.84008046109142498 ) ) ;
#45862=LINE ( 'NONE', #25880, #27434 ) ;
#45864=AXIS2_PLACEMENT_3D ( 'NONE', #17778, #33792, #22505 ) ;
#45865=VECTOR ( 'NONE', #31453, 1000.000000000000000 ) ;
#45872=ORIENTED_EDGE ( 'NONE', *, *, #2699, .T. ) ;
#45875=VECTOR ( 'NONE', #19313, 1000.000000000000114 ) ;
#45877=VECTOR ( 'NONE', #4873, 1000.000000000000000 ) ;
#45878=CARTESIAN_POINT ( 'NONE',  ( -330.4913330509368166, -116.7644047441726656, 59.62073260661660612 ) ) ;
#45880=CIRCLE ( 'NONE', #50911, 60.00000000000000000 ) ;
#45882=CARTESIAN_POINT ( 'NONE',  ( -339.1964088526558498, -96.52406086224361559, 52.47426709956096147 ) ) ;
#45886=ORIENTED_EDGE ( 'NONE', *, *, #30512, .T. ) ;
#45887=AXIS2_PLACEMENT_3D ( 'NONE', #10570, #3211, #3451 ) ;
#45889=EDGE_LOOP ( 'NONE', ( #30704, #25622, #24786, #16205 ) ) ;
#45891=AXIS2_PLACEMENT_3D ( 'NONE', #23864, #7074, #19408 ) ;
#45897=EDGE_CURVE ( 'NONE', #24889, #46461, #21850, .T. ) ;
#45903=CARTESIAN_POINT ( 'NONE',  ( -305.0000000000000568, -183.3224719910990643, -4.612141029301910500 ) ) ;
#45905=EDGE_LOOP ( 'NONE', ( #14979, #1719, #37246, #32064 ) ) ;
#45909=LINE ( 'NONE', #17269, #33173 ) ;
#45910=ORIENTED_EDGE ( 'NONE', *, *, #4419, .F. ) ;
#45911=VECTOR ( 'NONE', #16109, 1000.000000000000114 ) ;
#45913=CARTESIAN_POINT ( 'NONE',  ( -330.4913330509368166, -123.5000000000000284, 0.000000000000000000 ) ) ;
#45919=ADVANCED_FACE ( 'NONE', ( #22871 ), #39402, .T. ) ;
#45924=VECTOR ( 'NONE', #50275, 1000.000000000000114 ) ;
#45925=AXIS2_PLACEMENT_3D ( 'NONE', #11865, #47115, #7437 ) ;
#45926=EDGE_CURVE ( 'NONE', #9084, #32451, #30749, .T. ) ;
#45927=AXIS2_PLACEMENT_3D ( 'NONE', #35055, #31359, #47148 ) ;
#45936=CARTESIAN_POINT ( 'NONE',  ( -330.4913330509368166, -78.25935320507895199, 39.41172259083835172 ) ) ;
#45937=CARTESIAN_POINT ( 'NONE',  ( -336.3521761649654422, -73.44864141332200802, 31.34948880313848107 ) ) ;
#45944=VERTEX_POINT ( 'NONE', #10518 ) ;
#45946=ORIENTED_EDGE ( 'NONE', *, *, #42916, .F. ) ;
#45948=ORIENTED_EDGE ( 'NONE', *, *, #3033, .T. ) ;
#45949=CIRCLE ( 'NONE', #50969, 60.00000000000000000 ) ;
#45950=ORIENTED_EDGE ( 'NONE', *, *, #42964, .F. ) ;
#45955=LINE ( 'NONE', #1779, #19615 ) ;
#45956=CARTESIAN_POINT ( 'NONE',  ( -332.3517673607765914, -67.40061919120938683, 18.46045550523129819 ) ) ;
#45957=ORIENTED_EDGE ( 'NONE', *, *, #13811, .T. ) ;
#45959=EDGE_LOOP ( 'NONE', ( #4665, #13365, #43734, #48844 ) ) ;
#45965=DIRECTION ( 'NONE',  ( -0.000000000000000000, -1.000000000000000000, -0.000000000000000000 ) ) ;
#45967=ORIENTED_EDGE ( 'NONE', *, *, #30472, .T. ) ;
#45968=AXIS2_PLACEMENT_3D ( 'NONE', #26461, #18587, #34605 ) ;
#45971=EDGE_CURVE ( 'NONE', #13962, #13126, #46799, .T. ) ;
#45973=CARTESIAN_POINT ( 'NONE',  ( -330.4913330509368166, -123.5000000000000284, 0.000000000000000000 ) ) ;
#45975=AXIS2_PLACEMENT_3D ( 'NONE', #14220, #26280, #42058 ) ;
#45976=ORIENTED_EDGE ( 'NONE', *, *, #5144, .F. ) ;
#45977=CARTESIAN_POINT ( 'NONE',  ( -330.4913330509368166, -156.6043281241916816, -48.84008046109114076 ) ) ;
#45980=VECTOR ( 'NONE', #19233, 1000.000000000000000 ) ;
#45982=CARTESIAN_POINT ( 'NONE',  ( -330.4913330509368166, -102.1108035431471279, 54.98865587491800255 ) ) ;
#45984=CARTESIAN_POINT ( 'NONE',  ( -332.3517673607765914, -123.5000000000000284, 0.000000000000000000 ) ) ;
#45988=ORIENTED_EDGE ( 'NONE', *, *, #18270, .F. ) ;
#45989=ORIENTED_EDGE ( 'NONE', *, *, #30393, .F. ) ;
#45992=LINE ( 'NONE', #1813, #31224 ) ;
#45995=CARTESIAN_POINT ( 'NONE',  ( -339.1964088526558498, -79.66942718702493664, 39.49849221029193558 ) ) ;
#45998=EDGE_CURVE ( 'NONE', #17654, #43748, #26550, .T. ) ;
#46000=ORIENTED_EDGE ( 'NONE', *, *, #30039, .T. ) ;
#46001=DIRECTION ( 'NONE',  ( -0.000000000000000000, -0.7485107481710953081, 0.6631226582408016323 ) ) ;
#46002=VECTOR ( 'NONE', #35051, 999.9999999999998863 ) ;
#46003=VERTEX_POINT ( 'NONE', #15004 ) ;
#46007=CARTESIAN_POINT ( 'NONE',  ( -365.0000000000001137, -78.50000000000002842, -10.00000000000000711 ) ) ;
#46008=DIRECTION ( 'NONE',  ( -0.000000000000000000, -0.7485107481711046340, -0.6631226582407911962 ) ) ;
#46009=ORIENTED_EDGE ( 'NONE', *, *, #39678, .F. ) ;
#46013=PLANE ( 'NONE',  #21456 ) ;
#46014=VERTEX_POINT ( 'NONE', #7103 ) ;
#46016=ORIENTED_EDGE ( 'NONE', *, *, #17258, .F. ) ;
#46018=CARTESIAN_POINT ( 'NONE',  ( -330.4913330509368166, -64.50000000000000000, -0.4999999999999549249 ) ) ;
#46019=DIRECTION ( 'NONE',  ( 1.043714542225393381E-14, -0.4647231720437695057, -0.8854560256532093554 ) ) ;
#46025=DIRECTION ( 'NONE',  ( 0.000000000000000000, -0.9350162426854181641, -0.3546048870425267951 ) ) ;
#46026=CONICAL_SURFACE ( 'NONE', #9922, 10.00000000000000711, 0.03490658503988659789 ) ;
#46027=CARTESIAN_POINT ( 'NONE',  ( -339.1964088526558498, -78.92247586331968989, 40.16023333900940173 ) ) ;
#46028=ORIENTED_EDGE ( 'NONE', *, *, #19716, .F. ) ;
#46030=CARTESIAN_POINT ( 'NONE',  ( -330.4913330509368166, -90.39567187580801999, 48.84008046109089918 ) ) ;
#46031=CARTESIAN_POINT ( 'NONE',  ( -336.3521761649654422, -100.1170788342122080, 54.23253582808833073 ) ) ;
#46034=DIRECTION ( 'NONE',  ( -8.718379230999708359E-17, 0.5680647467311569221, 0.8229838658936556861 ) ) ;
#46042=VECTOR ( 'NONE', #2853, 1000.000000000000000 ) ;
#46044=PLANE ( 'NONE',  #21932 ) ;
#46047=DIRECTION ( 'NONE',  ( -0.000000000000000000, -0.8229838658936516893, 0.5680647467311626952 ) ) ;
#46053=ORIENTED_EDGE ( 'NONE', *, *, #2576, .F. ) ;
#46054=DIRECTION ( 'NONE',  ( 1.000000000000000000, -0.000000000000000000, -0.000000000000000000 ) ) ;
#46056=CARTESIAN_POINT ( 'NONE',  ( -339.1964088526558498, -179.4217241332784454, -21.74306257088698757 ) ) ;
#46058=AXIS2_PLACEMENT_3D ( 'NONE', #631, #27702, #47945 ) ;
#46062=DIRECTION ( 'NONE',  ( 0.000000000000000000, 0.000000000000000000, -1.000000000000000000 ) ) ;
#46063=VECTOR ( 'NONE', #5467, 1000.000000000000000 ) ;
#46067=ORIENTED_EDGE ( 'NONE', *, *, #38812, .F. ) ;
#46069=DIRECTION ( 'NONE',  ( 0.000000000000000000, 0.000000000000000000, -1.000000000000000000 ) ) ;
#46071=DIRECTION ( 'NONE',  ( 0.000000000000000000, 0.7485107481711046340, 0.6631226582407911962 ) ) ;
#46072=ORIENTED_EDGE ( 'NONE', *, *, #29214, .F. ) ;
#46075=ORIENTED_EDGE ( 'NONE', *, *, #47814, .T. ) ;
#46077=ORIENTED_EDGE ( 'NONE', *, *, #26485, .F. ) ;
#46088=PLANE ( 'NONE',  #23214 ) ;
#46090=EDGE_CURVE ( 'NONE', #18701, #20460, #12587, .T. ) ;
#46092=EDGE_CURVE ( 'NONE', #903, #37560, #16555, .T. ) ;
#46094=EDGE_LOOP ( 'NONE', ( #26469, #29479 ) ) ;
#46095=DIRECTION ( 'NONE',  ( 0.000000000000000000, 0.000000000000000000, 1.000000000000000000 ) ) ;
#46097=EDGE_CURVE ( 'NONE', #39066, #22193, #24676, .T. ) ;
#46105=DIRECTION ( 'NONE',  ( -8.718379230999707126E-17, 1.000000000000000000, -3.491481338843133355E-15 ) ) ;
#46106=CARTESIAN_POINT ( 'NONE',  ( -339.1964088526558498, -115.8919814278862503, 58.50955523165745831 ) ) ;
#46108=CARTESIAN_POINT ( 'NONE',  ( -336.3521761649654422, -163.8460225846223466, -43.07972642080364523 ) ) ;
#46113=CARTESIAN_POINT ( 'NONE',  ( -336.3521761649654422, -154.8494888031386836, 50.05135858667791382 ) ) ;
#46114=ORIENTED_EDGE ( 'NONE', *, *, #26313, .T. ) ;
#46115=ORIENTED_EDGE ( 'NONE', *, *, #22895, .F. ) ;
#46119=DIRECTION ( 'NONE',  ( -1.000000000000000000, 2.497772389992407926E-15, -1.013386094502326665E-14 ) ) ;
#46132=CIRCLE ( 'NONE', #43593, 60.00000000000000000 ) ;
#46134=CARTESIAN_POINT ( 'NONE',  ( -336.3521761649653854, -90.77207769297352513, -50.28800156563429624 ) ) ;
#46135=ORIENTED_EDGE ( 'NONE', *, *, #5033, .T. ) ;
#46140=EDGE_LOOP ( 'NONE', ( #44357, #3161, #29252, #39041 ) ) ;
#46142=ORIENTED_EDGE ( 'NONE', *, *, #11005, .F. ) ;
#46143=DIRECTION ( 'NONE',  ( 0.000000000000000000, 0.5680647467311656929, 0.8229838658936495799 ) ) ;
#46144=DIRECTION ( 'NONE',  ( 1.000000000000000000, -0.000000000000000000, -0.000000000000000000 ) ) ;
#46146=LINE ( 'NONE', #10129, #27638 ) ;
#46147=ORIENTED_EDGE ( 'NONE', *, *, #30745, .F. ) ;
#46151=ADVANCED_FACE ( 'NONE', ( #233 ), #7866, .F. ) ;
#46154=CARTESIAN_POINT ( 'NONE',  ( -332.3517673607765914, -64.61288906875131488, 4.498567634385603142 ) ) ;
#46155=EDGE_CURVE ( 'NONE', #50347, #3155, #43614, .T. ) ;
#46156=DIRECTION ( 'NONE',  ( -1.000000000000000000, 0.000000000000000000, 0.000000000000000000 ) ) ;
#46166=VECTOR ( 'NONE', #46054, 1000.000000000000000 ) ;
#46168=ORIENTED_EDGE ( 'NONE', *, *, #46865, .T. ) ;
#46170=CARTESIAN_POINT ( 'NONE',  ( -305.0000000000000568, -116.7644047441726656, 59.62073260661660612 ) ) ;
#46172=PRODUCT_DEFINITION_SHAPE ( 'NONE', 'NONE',  #19619 ) ;
#46178=CARTESIAN_POINT ( 'NONE',  ( -336.3521761649654422, -65.24746378767824240, -9.724760635741734660 ) ) ;
#46181=EDGE_LOOP ( 'NONE', ( #12926, #44577 ) ) ;
#46182=VERTEX_POINT ( 'NONE', #44131 ) ;
#46185=DIRECTION ( 'NONE',  ( -0.000000000000000000, 0.9350162426854181641, 0.3546048870425267951 ) ) ;
#46187=ADVANCED_FACE ( 'NONE', ( #32289 ), #24174, .T. ) ;
#46189=LINE ( 'NONE', #10168, #50510 ) ;
#46192=EDGE_CURVE ( 'NONE', #12138, #10791, #36490, .T. ) ;
#46194=EDGE_CURVE ( 'NONE', #32451, #44682, #39752, .T. ) ;
#46195=ADVANCED_FACE ( 'NONE', ( #21785 ), #45704, .F. ) ;
#46196=LINE ( 'NONE', #26722, #7256 ) ;
#46202=EDGE_CURVE ( 'NONE', #8114, #10774, #13633, .T. ) ;
#46205=PLANE ( 'NONE',  #46773 ) ;
#46211=CARTESIAN_POINT ( 'NONE',  ( -305.0000000000000568, -78.92247586331968989, 40.16023333900940884 ) ) ;
#46217=ADVANCED_FACE ( 'NONE', ( #41479 ), #25978, .T. ) ;
#46219=DIRECTION ( 'NONE',  ( 0.000000000000000000, -0.9350162426854181641, -0.3546048870425267951 ) ) ;
#46220=ORIENTED_EDGE ( 'NONE', *, *, #28920, .F. ) ;
#46223=EDGE_CURVE ( 'NONE', #11668, #3041, #33604, .T. ) ;
#46226=ORIENTED_EDGE ( 'NONE', *, *, #20266, .F. ) ;
#46229=EDGE_CURVE ( 'NONE', #40642, #16896, #28869, .T. ) ;
#46230=AXIS2_PLACEMENT_3D ( 'NONE', #27620, #39437, #43128 ) ;
#46231=AXIS2_PLACEMENT_3D ( 'NONE', #30555, #10857, #34252 ) ;
#46233=EDGE_LOOP ( 'NONE', ( #26456, #25177, #22015, #14950 ) ) ;
#46236=ORIENTED_EDGE ( 'NONE', *, *, #31394, .T. ) ;
#46238=ORIENTED_EDGE ( 'NONE', *, *, #30039, .F. ) ;
#46240=LINE ( 'NONE', #10214, #7485 ) ;
#46246=ORIENTED_EDGE ( 'NONE', *, *, #38489, .F. ) ;
#46255=ADVANCED_FACE ( 'NONE', ( #13112 ), #49644, .T. ) ;
#46256=EDGE_CURVE ( 'NONE', #19012, #34105, #29681, .T. ) ;
#46257=EDGE_CURVE ( 'NONE', #47856, #34569, #771, .T. ) ;
#46258=CIRCLE ( 'NONE', #44555, 20.00000000000001776 ) ;
#46260=DIRECTION ( 'NONE',  ( -1.000000000000000000, 0.000000000000000000, -0.000000000000000000 ) ) ;
#46262=DIRECTION ( 'NONE',  ( -0.000000000000000000, -0.4647231720437724478, -0.8854560256532078011 ) ) ;
#46264=ORIENTED_EDGE ( 'NONE', *, *, #552, .T. ) ;
#46265=DIRECTION ( 'NONE',  ( 1.000000000000000000, -0.000000000000000000, -0.000000000000000000 ) ) ;
#46267=DIRECTION ( 'NONE',  ( 0.000000000000000000, 0.000000000000000000, 1.000000000000000000 ) ) ;
#46268=EDGE_LOOP ( 'NONE', ( #10871, #36912, #47795, #13573 ) ) ;
#46269=DIRECTION ( 'NONE',  ( 1.000000000000000000, 0.000000000000000000, -0.000000000000000000 ) ) ;
#46270=CARTESIAN_POINT ( 'NONE',  ( -339.1964088526558498, -144.8891964568517778, 54.98865587491845730 ) ) ;
#46280=ORIENTED_EDGE ( 'NONE', *, *, #26945, .F. ) ;
#46283=CARTESIAN_POINT ( 'NONE',  ( -339.1964088526558498, -68.15673923803930734, -20.45418021416698551 ) ) ;
#46285=DIRECTION ( 'NONE',  ( -1.000000000000000000, 0.000000000000000000, 0.000000000000000000 ) ) ;
#46296=AXIS2_PLACEMENT_3D ( 'NONE', #50104, #34563, #42729 ) ;
#46299=CIRCLE ( 'NONE', #957, 60.00000000000000000 ) ;
#46300=CARTESIAN_POINT ( 'NONE',  ( -336.3521761649654422, -74.01670616005314685, 32.17247266903214609 ) ) ;
#46301=CARTESIAN_POINT ( 'NONE',  ( -336.3521761649654422, -67.40061919120938683, 18.46045550523129819 ) ) ;
#46302=DIRECTION ( 'NONE',  ( -0.000000000000000000, -0.9927088740980548609, -0.1205366802553164696 ) ) ;
#46305=LINE ( 'NONE', #30260, #4213 ) ;
#46307=CARTESIAN_POINT ( 'NONE',  ( -336.3521761649654422, -126.1322888500942270, -59.00000000000001421 ) ) ;
#46309=ORIENTED_EDGE ( 'NONE', *, *, #46490, .T. ) ;
#46313=LINE ( 'NONE', #2662, #26720 ) ;
#46314=ADVANCED_FACE ( 'NONE', ( #34122 ), #6790, .F. ) ;
#46318=VERTEX_POINT ( 'NONE', #50174 ) ;
#46319=CARTESIAN_POINT ( 'NONE',  ( -339.1964088526558498, -109.8658467157464571, 57.40522506028071348 ) ) ;
#46321=DIRECTION ( 'NONE',  ( -0.000000000000000000, 0.4647231720437789981, 0.8854560256532044704 ) ) ;
#46328=CARTESIAN_POINT ( 'NONE',  ( -336.3521761649654422, -120.8677111499054320, 59.00000000000000000 ) ) ;
#46329=CARTESIAN_POINT ( 'NONE',  ( -305.0000000000000568, -74.40671499923389831, 34.49419324804615172 ) ) ;
#46332=VECTOR ( 'NONE', #40508, 1000.000000000000000 ) ;
#46333=ORIENTED_EDGE ( 'NONE', *, *, #38339, .T. ) ;
#46337=EDGE_CURVE ( 'NONE', #23338, #31250, #2335, .T. ) ;
#46338=CARTESIAN_POINT ( 'NONE',  ( -330.4913330509368166, -66.33409060400650503, 14.60509510167813474 ) ) ;
#46341=FACE_BOUND ( 'NONE', #40040, .T. ) ;
#46343=PLANE ( 'NONE',  #40732 ) ;
#46354=LINE ( 'NONE', #22168, #11254 ) ;
#46355=FACE_OUTER_BOUND ( 'NONE', #43711, .T. ) ;
#46357=DIRECTION ( 'NONE',  ( 0.000000000000000000, 0.9709418174260553425, 0.2393156642875448881 ) ) ;
#46361=CARTESIAN_POINT ( 'NONE',  ( -339.1964088526558498, -122.9999999999993747, 59.00000000000002132 ) ) ;
#46371=ORIENTED_EDGE ( 'NONE', *, *, #42403, .F. ) ;
#46372=CARTESIAN_POINT ( 'NONE',  ( -339.1964088526558498, -178.4886558749184076, -21.38919645685194837 ) ) ;
#46375=CARTESIAN_POINT ( 'NONE',  ( -339.1964088526558498, -182.1300919119128423, 6.615309698015510165 ) ) ;
#46379=VECTOR ( 'NONE', #20592, 1000.000000000000000 ) ;
#46380=ORIENTED_EDGE ( 'NONE', *, *, #18683, .F. ) ;
#46387=CARTESIAN_POINT ( 'NONE',  ( -339.1964088526558498, -181.6348283828473029, -14.84391218300937432 ) ) ;
#46391=ORIENTED_EDGE ( 'NONE', *, *, #37041, .T. ) ;
#46394=ADVANCED_FACE ( 'NONE', ( #27000 ), #18096, .T. ) ;
#46398=LINE ( 'NONE', #42712, #43022 ) ;
#46402=AXIS2_PLACEMENT_3D ( 'NONE', #5581, #44734, #8721 ) ;
#46405=CARTESIAN_POINT ( 'NONE',  ( -339.1964088526558498, -156.6043281241909426, 48.84008046109164525 ) ) ;
#46411=DIRECTION ( 'NONE',  ( 0.000000000000000000, 0.9927088740980535286, -0.1205366802553268502 ) ) ;
#46412=VECTOR ( 'NONE', #24134, 1000.000000000000000 ) ;
#46413=DIRECTION ( 'NONE',  ( -1.000000000000000000, 4.850383327712019318E-15, 9.241633304753524009E-15 ) ) ;
#46416=FACE_OUTER_BOUND ( 'NONE', #37438, .T. ) ;
#46417=EDGE_LOOP ( 'NONE', ( #5547, #24099, #11845, #39726 ) ) ;
#46419=EDGE_LOOP ( 'NONE', ( #43248, #29908, #7037, #34497 ) ) ;
#46420=LINE ( 'NONE', #35351, #6990 ) ;
#46421=ORIENTED_EDGE ( 'NONE', *, *, #33616, .T. ) ;
#46424=ORIENTED_EDGE ( 'NONE', *, *, #34955, .F. ) ;
#46427=ORIENTED_EDGE ( 'NONE', *, *, #2238, .T. ) ;
#46428=DIRECTION ( 'NONE',  ( 1.000000000000000000, -0.000000000000000000, 0.000000000000000000 ) ) ;
#46434=ORIENTED_EDGE ( 'NONE', *, *, #1879, .F. ) ;
#46437=VECTOR ( 'NONE', #32379, 1000.000000000000000 ) ;
#46438=ORIENTED_EDGE ( 'NONE', *, *, #18425, .F. ) ;
#46439=DIRECTION ( 'NONE',  ( 0.000000000000000000, -0.9927088740980553050, -0.1205366802553130001 ) ) ;
#46440=DIRECTION ( 'NONE',  ( -0.000000000000000000, 0.000000000000000000, 1.000000000000000000 ) ) ;
#46442=CARTESIAN_POINT ( 'NONE',  ( -336.3521761649654422, -180.1556192733800117, 16.67542351306693149 ) ) ;
#46445=AXIS2_PLACEMENT_3D ( 'NONE', #20005, #20133, #20387 ) ;
#46447=ORIENTED_EDGE ( 'NONE', *, *, #5328, .F. ) ;
#46454=DIRECTION ( 'NONE',  ( -1.000000000000000000, 0.000000000000000000, 0.000000000000000000 ) ) ;
#46455=EDGE_LOOP ( 'NONE', ( #7436, #41556, #11766, #19108 ) ) ;
#46458=DIRECTION ( 'NONE',  ( -1.000000000000000000, 0.000000000000000000, -0.000000000000000000 ) ) ;
#46459=VERTEX_POINT ( 'NONE', #48280 ) ;
#46461=VERTEX_POINT ( 'NONE', #35662 ) ;
#46465=DIRECTION ( 'NONE',  ( 0.000000000000000000, -0.000000000000000000, 1.000000000000000000 ) ) ;
#46469=CARTESIAN_POINT ( 'NONE',  ( -336.3521761649654422, -170.5607375887735770, 35.68215131113770155 ) ) ;
#46474=CARTESIAN_POINT ( 'NONE',  ( -332.3517673607765914, -88.08538291676191534, 48.43351006119235080 ) ) ;
#46478=DIRECTION ( 'NONE',  ( -1.000000000000000000, 6.921107616850682476E-15, -7.812315528781957664E-15 ) ) ;
#46482=VERTEX_POINT ( 'NONE', #43805 ) ;
#46490=EDGE_CURVE ( 'NONE', #44016, #40473, #27522, .T. ) ;
#46496=CARTESIAN_POINT ( 'NONE',  ( -339.1964088526558498, -123.5000000000000284, 0.000000000000000000 ) ) ;
#46497=ORIENTED_EDGE ( 'NONE', *, *, #49090, .T. ) ;
#46499=EDGE_CURVE ( 'NONE', #26309, #35813, #4142, .T. ) ;
#46502=CIRCLE ( 'NONE', #7882, 60.00000000000000000 ) ;
#46503=EDGE_CURVE ( 'NONE', #43725, #23668, #12000, .T. ) ;
#46506=DIRECTION ( 'NONE',  ( -0.000000000000000000, 0.9927088740980538617, -0.1205366802553232974 ) ) ;
#46509=LINE ( 'NONE', #43331, #47686 ) ;
#46510=CARTESIAN_POINT ( 'NONE',  ( -339.1964088526558498, -143.9541802141672235, -55.34326076196065003 ) ) ;
#46511=ORIENTED_EDGE ( 'NONE', *, *, #42988, .F. ) ;
#46515=VERTEX_POINT ( 'NONE', #12530 ) ;
#46519=VERTEX_POINT ( 'NONE', #28028 ) ;
#46520=AXIS2_PLACEMENT_3D ( 'NONE', #6508, #30390, #2021 ) ;
#46521=EDGE_CURVE ( 'NONE', #28174, #51399, #40124, .T. ) ;
#46523=DIRECTION ( 'NONE',  ( -0.000000000000000000, 0.6631226582408039638, 0.7485107481710934207 ) ) ;
#46524=ORIENTED_EDGE ( 'NONE', *, *, #1927, .F. ) ;
#46527=ORIENTED_EDGE ( 'NONE', *, *, #42745, .F. ) ;
#46530=DIRECTION ( 'NONE',  ( 0.000000000000000000, -0.000000000000000000, 1.000000000000000000 ) ) ;
#46531=DIRECTION ( 'NONE',  ( -1.000000000000000000, 0.000000000000000000, 0.000000000000000000 ) ) ;
#46532=CARTESIAN_POINT ( 'NONE',  ( -305.0000000000000568, -181.6348283828471608, 14.84391218300993209 ) ) ;
#46536=FACE_OUTER_BOUND ( 'NONE', #40086, .T. ) ;
#46538=DIRECTION ( 'NONE',  ( 0.000000000000000000, 0.000000000000000000, -1.000000000000000000 ) ) ;
#46541=DIRECTION ( 'NONE',  ( -0.000000000000000000, 0.8229838658936494689, -0.5680647467311658039 ) ) ;
#46544=EDGE_CURVE ( 'NONE', #14073, #15388, #51711, .T. ) ;
#46551=ADVANCED_FACE ( 'NONE', ( #19383 ), #3874, .F. ) ;
#46558=AXIS2_PLACEMENT_3D ( 'NONE', #24848, #40869, #36939 ) ;
#46566=LINE ( 'NONE', #10549, #29235 ) ;
#46567=EDGE_CURVE ( 'NONE', #6623, #4319, #46502, .T. ) ;
#46571=EDGE_CURVE ( 'NONE', #27996, #37301, #20673, .T. ) ;
#46578=LINE ( 'NONE', #14001, #4605 ) ;
#46579=VECTOR ( 'NONE', #30531, 1000.000000000000000 ) ;
#46580=ORIENTED_EDGE ( 'NONE', *, *, #30880, .F. ) ;
#46581=CARTESIAN_POINT ( 'NONE',  ( -336.3521761649654422, -123.5000000000000284, 0.000000000000000000 ) ) ;
#46583=VECTOR ( 'NONE', #12131, 1000.000000000000227 ) ;
#46585=LINE ( 'NONE', #42882, #26324 ) ;
#46591=VERTEX_POINT ( 'NONE', #17004 ) ;
#46595=DIRECTION ( 'NONE',  ( -0.000000000000000000, -0.9350162426854121689, 0.3546048870425426158 ) ) ;
#46607=CARTESIAN_POINT ( 'NONE',  ( -330.4913330509368166, -95.63860483659048839, 52.00954392751722111 ) ) ;
#46610=ADVANCED_FACE ( 'NONE', ( #13313 ), #44851, .F. ) ;
#46612=CARTESIAN_POINT ( 'NONE',  ( -332.3517673607765914, -118.0087234915157381, -58.76657425099333665 ) ) ;
#46616=DIRECTION ( 'NONE',  ( -0.000000000000000000, -0.3546048870425396182, -0.9350162426854132791 ) ) ;
#46619=ORIENTED_EDGE ( 'NONE', *, *, #21697, .T. ) ;
#46623=DIRECTION ( 'NONE',  ( -1.000000000000000000, -0.000000000000000000, 0.000000000000000000 ) ) ;
#46624=VECTOR ( 'NONE', #4392, 1000.000000000000000 ) ;
#46626=ORIENTED_EDGE ( 'NONE', *, *, #43645, .F. ) ;
#46627=CARTESIAN_POINT ( 'NONE',  ( 0.000000000000000000, -175.7419055135392227, 27.41866715058277038 ) ) ;
#46629=EDGE_CURVE ( 'NONE', #42654, #26038, #39754, .T. ) ;
#46630=ORIENTED_EDGE ( 'NONE', *, *, #22506, .T. ) ;
#46633=AXIS2_PLACEMENT_3D ( 'NONE', #17862, #18119, #26246 ) ;
#46635=VECTOR ( 'NONE', #46265, 1000.000000000000000 ) ;
#46637=ORIENTED_EDGE ( 'NONE', *, *, #3190, .F. ) ;
#46646=EDGE_LOOP ( 'NONE', ( #506, #20756, #45702, #26589 ) ) ;
#46648=DIRECTION ( 'NONE',  ( -1.000000000000000000, 0.000000000000000000, 0.000000000000000000 ) ) ;
#46649=EDGE_LOOP ( 'NONE', ( #965, #47672, #42735, #27147 ) ) ;
#46650=VERTEX_POINT ( 'NONE', #607 ) ;
#46659=ORIENTED_EDGE ( 'NONE', *, *, #42330, .F. ) ;
#46662=LINE ( 'NONE', #5698, #988 ) ;
#46670=DIRECTION ( 'NONE',  ( -1.000000000000000000, 0.000000000000000000, 0.000000000000000000 ) ) ;
#46671=VECTOR ( 'NONE', #19328, 1000.000000000000000 ) ;
#46681=ORIENTED_EDGE ( 'NONE', *, *, #49713, .T. ) ;
#46682=FACE_OUTER_BOUND ( 'NONE', #41200, .T. ) ;
#46683=CARTESIAN_POINT ( 'NONE',  ( -336.3521761649654422, -81.08339623743702873, -41.09453333279329712 ) ) ;
#46689=DIRECTION ( 'NONE',  ( 0.000000000000000000, 0.9927088740980534176, -0.1205366802553268502 ) ) ;
#46690=DIRECTION ( 'NONE',  ( 0.000000000000000000, 0.000000000000000000, 1.000000000000000000 ) ) ;
#46691=ORIENTED_EDGE ( 'NONE', *, *, #7912, .F. ) ;
#46693=ORIENTED_EDGE ( 'NONE', *, *, #24061, .T. ) ;
#46694=DIRECTION ( 'NONE',  ( 0.000000000000000000, 6.846375318521798245E-14, 1.000000000000000000 ) ) ;
#46700=LINE ( 'NONE', #43255, #33729 ) ;
#46703=ORIENTED_EDGE ( 'NONE', *, *, #34041, .T. ) ;
#46704=ADVANCED_FACE ( 'NONE', ( #44762 ), #12433, .F. ) ;
#46706=VECTOR ( 'NONE', #36093, 1000.000000000000000 ) ;
#46710=VERTEX_POINT ( 'NONE', #20062 ) ;
#46715=DIRECTION ( 'NONE',  ( -1.000000000000000000, 0.000000000000000000, 0.000000000000000000 ) ) ;
#46716=ORIENTED_EDGE ( 'NONE', *, *, #7285, .T. ) ;
#46719=EDGE_CURVE ( 'NONE', #25876, #30123, #28454, .T. ) ;
#46720=ORIENTED_EDGE ( 'NONE', *, *, #6, .F. ) ;
#46729=PLANE ( 'NONE',  #44050 ) ;
#46730=VECTOR ( 'NONE', #31258, 1000.000000000000000 ) ;
#46734=ORIENTED_EDGE ( 'NONE', *, *, #24780, .T. ) ;
#46735=DIRECTION ( 'NONE',  ( 0.000000000000000000, -0.9350162426854107256, 0.3546048870425463906 ) ) ;
#46737=ADVANCED_FACE ( 'NONE', ( #19543 ), #24517, .F. ) ;
#46743=LINE ( 'NONE', #10982, #34813 ) ;
#46747=ORIENTED_EDGE ( 'NONE', *, *, #34656, .T. ) ;
#46748=CARTESIAN_POINT ( 'NONE',  ( -339.1964088526558498, -65.36517161715264024, 14.84391218300897108 ) ) ;
#46750=ORIENTED_EDGE ( 'NONE', *, *, #18120, .T. ) ;
#46751=DIRECTION ( 'NONE',  ( -0.000000000000000000, 0.8854560256532043594, -0.4647231720437789981 ) ) ;
#46756=LINE ( 'NONE', #43824, #27718 ) ;
#46757=ORIENTED_EDGE ( 'NONE', *, *, #49119, .T. ) ;
#46762=ORIENTED_EDGE ( 'NONE', *, *, #38670, .T. ) ;
#46767=ORIENTED_EDGE ( 'NONE', *, *, #25418, .F. ) ;
#46768=CARTESIAN_POINT ( 'NONE',  ( -330.4913330509368166, -96.52406086224361559, 52.47426709956096147 ) ) ;
#46770=EDGE_LOOP ( 'NONE', ( #34389, #35893, #35329, #2774 ) ) ;
#46771=VECTOR ( 'NONE', #22197, 1000.000000000000114 ) ;
#46773=AXIS2_PLACEMENT_3D ( 'NONE', #10181, #17815, #38562 ) ;
#46782=DIRECTION ( 'NONE',  ( -8.718379230999705894E-17, -0.9350162426854181641, -0.3546048870425267951 ) ) ;
#46784=EDGE_LOOP ( 'NONE', ( #41396, #6189, #39711, #25611 ) ) ;
#46789=DIRECTION ( 'NONE',  ( -0.000000000000000000, 0.000000000000000000, -1.000000000000000000 ) ) ;
#46792=CARTESIAN_POINT ( 'NONE',  ( -339.1964088526558498, -90.39567187580880159, -48.84008046109142498 ) ) ;
#46795=PLANE ( 'NONE',  #6681 ) ;
#46799=LINE ( 'NONE', #10788, #2785 ) ;
#46803=ORIENTED_EDGE ( 'NONE', *, *, #7688, .F. ) ;
#46804=CIRCLE ( 'NONE', #21627, 60.00000000000000000 ) ;
#46806=ADVANCED_FACE ( 'NONE', ( #37121 ), #14003, .T. ) ;
#46809=DIRECTION ( 'NONE',  ( -0.000000000000000000, 0.6631226582407937498, -0.7485107481711024136 ) ) ;
#46813=CARTESIAN_POINT ( 'NONE',  ( -332.3517673607765914, -175.8491356171901145, 29.31839013542587224 ) ) ;
#46817=CIRCLE ( 'NONE', #6530, 60.00000000000000000 ) ;
#46820=DIRECTION ( 'NONE',  ( 1.000000000000000000, -0.000000000000000000, -0.000000000000000000 ) ) ;
#46822=CARTESIAN_POINT ( 'NONE',  ( -332.3517673607765914, -66.60506506233235768, -15.70448169564047092 ) ) ;
#46823=AXIS2_PLACEMENT_3D ( 'NONE', #9216, #49676, #12618 ) ;
#46825=ORIENTED_EDGE ( 'NONE', *, *, #21789, .T. ) ;
#46826=ORIENTED_EDGE ( 'NONE', *, *, #7986, .F. ) ;
#46828=CARTESIAN_POINT ( 'NONE',  ( -305.0000000000000568, -165.2193480479701293, -43.12187378178659714 ) ) ;
#46830=CARTESIAN_POINT ( 'NONE',  ( -339.1964088526558498, -131.1080185721133660, -58.50955523165751515 ) ) ;
#46833=FACE_OUTER_BOUND ( 'NONE', #35416, .T. ) ;
#46836=LINE ( 'NONE', #3200, #20775 ) ;
#46843=VECTOR ( 'NONE', #44226, 1000.000000000000000 ) ;
#46848=DIRECTION ( 'NONE',  ( -0.000000000000000000, -0.9350162426854121689, 0.3546048870425426158 ) ) ;
#46849=FACE_OUTER_BOUND ( 'NONE', #38712, .T. ) ;
#46852=EDGE_CURVE ( 'NONE', #23160, #3747, #9798, .T. ) ;
#46855=DIRECTION ( 'NONE',  ( -1.000000000000000000, -0.000000000000000000, -0.000000000000000000 ) ) ;
#46856=FACE_OUTER_BOUND ( 'NONE', #4133, .T. ) ;
#46860=FACE_OUTER_BOUND ( 'NONE', #40885, .T. ) ;
#46862=FACE_BOUND ( 'NONE', #26373, .T. ) ;
#46865=EDGE_CURVE ( 'NONE', #13250, #8786, #25059, .T. ) ;
#46866=AXIS2_PLACEMENT_3D ( 'NONE', #30226, #46269, #26267 ) ;
#46869=ORIENTED_EDGE ( 'NONE', *, *, #27610, .T. ) ;
#46870=EDGE_CURVE ( 'NONE', #42377, #23944, #9537, .T. ) ;
#46873=ORIENTED_EDGE ( 'NONE', *, *, #17371, .T. ) ;
#46874=EDGE_CURVE ( 'NONE', #12363, #27774, #45546, .T. ) ;
#46876=DIRECTION ( 'NONE',  ( -0.000000000000000000, 0.000000000000000000, 1.000000000000000000 ) ) ;
#46880=DIRECTION ( 'NONE',  ( -0.000000000000000000, -0.6631226582407989678, -0.7485107481710977506 ) ) ;
#46882=VECTOR ( 'NONE', #15898, 1000.000000000000000 ) ;
#46889=EDGE_LOOP ( 'NONE', ( #22069, #301, #38889, #17464 ) ) ;
#46891=ADVANCED_FACE ( 'NONE', ( #9281 ), #17443, .F. ) ;
#46894=VERTEX_POINT ( 'NONE', #29490 ) ;
#46895=FACE_OUTER_BOUND ( 'NONE', #42469, .T. ) ;
#46905=LINE ( 'NONE', #10885, #5671 ) ;
#46906=DIRECTION ( 'NONE',  ( -1.000000000000000000, 0.000000000000000000, 0.000000000000000000 ) ) ;
#46913=EDGE_CURVE ( 'NONE', #31214, #41614, #49230, .T. ) ;
#46914=CARTESIAN_POINT ( 'NONE',  ( -336.3521761649654422, -166.5797264208035244, 40.34602258462248159 ) ) ;
#46919=VERTEX_POINT ( 'NONE', #18974 ) ;
#46922=CARTESIAN_POINT ( 'NONE',  ( -332.3517673607765914, -81.08339623743702873, -41.09453333279329712 ) ) ;
#46924=LINE ( 'NONE', #23255, #22497 ) ;
#46927=DIRECTION ( 'NONE',  ( 0.000000000000000000, 0.3546048870425300148, -0.9350162426854169428 ) ) ;
#46928=CARTESIAN_POINT ( 'NONE',  ( -339.1964088526558498, -123.9999999999993747, 59.00000000000002132 ) ) ;
#46931=VERTEX_POINT ( 'NONE', #38673 ) ;
#46937=LINE ( 'NONE', #27185, #31409 ) ;
#46941=CIRCLE ( 'NONE', #15873, 60.00000000000000000 ) ;
#46955=ORIENTED_EDGE ( 'NONE', *, *, #36497, .T. ) ;
#46958=EDGE_CURVE ( 'NONE', #49907, #34582, #6246, .T. ) ;
#46959=DIRECTION ( 'NONE',  ( 1.000000000000000000, -0.000000000000000000, -0.000000000000000000 ) ) ;
#46963=ORIENTED_EDGE ( 'NONE', *, *, #2010, .T. ) ;
#46966=DIRECTION ( 'NONE',  ( 1.000000000000000000, -0.000000000000000000, -0.000000000000000000 ) ) ;
#46969=VERTEX_POINT ( 'NONE', #30797 ) ;
#46970=ADVANCED_FACE ( 'NONE', ( #34477 ), #2435, .F. ) ;
#46979=DIRECTION ( 'NONE',  ( 0.000000000000000000, -0.6631226582408016323, -0.7485107481710953081 ) ) ;
#46984=EDGE_LOOP ( 'NONE', ( #21677, #27195, #16112, #21440 ) ) ;
#47007=ORIENTED_EDGE ( 'NONE', *, *, #49191, .F. ) ;
#47013=CARTESIAN_POINT ( 'NONE',  ( -330.4913330509368166, -181.8741440471346493, 13.87297036558422825 ) ) ;
#47018=CIRCLE ( 'NONE', #9250, 60.00000000000000000 ) ;
#47019=VERTEX_POINT ( 'NONE', #2161 ) ;
#47022=ADVANCED_FACE ( 'NONE', ( #31047 ), #14784, .F. ) ;
#47024=CARTESIAN_POINT ( 'NONE',  ( -332.3517673607765914, -154.8494888031386836, 50.05135858667791382 ) ) ;
#47029=EDGE_CURVE ( 'NONE', #35813, #23503, #14522, .T. ) ;
#47031=EDGE_LOOP ( 'NONE', ( #2022, #44505, #19533, #12749 ) ) ;
#47032=LINE ( 'NONE', #14461, #23047 ) ;
#47033=EDGE_LOOP ( 'NONE', ( #51171, #34456, #40940, #7078 ) ) ;
#47034=EDGE_CURVE ( 'NONE', #1525, #23565, #27097, .T. ) ;
#47035=CARTESIAN_POINT ( 'NONE',  ( -330.4913330509368166, -175.9742670995611036, 26.97593913775620678 ) ) ;
#47037=CARTESIAN_POINT ( 'NONE',  ( -339.1964088526558498, -181.6348283828470755, 14.84391218301028026 ) ) ;
#47048=EDGE_CURVE ( 'NONE', #28063, #12334, #35763, .T. ) ;
#47051=DIRECTION ( 'NONE',  ( 1.000000000000000000, -0.000000000000000000, -0.000000000000000000 ) ) ;
#47053=ORIENTED_EDGE ( 'NONE', *, *, #681, .T. ) ;
#47059=VECTOR ( 'NONE', #12017, 1000.000000000000000 ) ;
#47062=CARTESIAN_POINT ( 'NONE',  ( -332.3517673607765914, -123.5000000000000284, 0.000000000000000000 ) ) ;
#47063=LINE ( 'NONE', #51021, #31944 ) ;
#47064=CARTESIAN_POINT ( 'NONE',  ( -340.0000000000000568, -168.5000000000000284, -5.000000000000001776 ) ) ;
#47076=AXIS2_PLACEMENT_3D ( 'NONE', #47838, #11808, #27837 ) ;
#47077=DIRECTION ( 'NONE',  ( -1.000000000000000000, 0.000000000000000000, 0.000000000000000000 ) ) ;
#47078=ORIENTED_EDGE ( 'NONE', *, *, #39408, .F. ) ;
#47080=VERTEX_POINT ( 'NONE', #11324 ) ;
#47084=ORIENTED_EDGE ( 'NONE', *, *, #1576, .F. ) ;
#47085=ADVANCED_FACE ( 'NONE', ( #39688 ), #16595, .F. ) ;
#47088=LINE ( 'NONE', #11064, #4015 ) ;
#47089=CARTESIAN_POINT ( 'NONE',  ( -305.0000000000000568, -162.0508476703726330, 45.97643030831914501 ) ) ;
#47090=ORIENTED_EDGE ( 'NONE', *, *, #45012, .F. ) ;
#47093=LINE ( 'NONE', #35760, #39026 ) ;
#47095=CARTESIAN_POINT ( 'NONE',  ( -332.3517673607765914, -180.1556192733800117, 16.67542351306693149 ) ) ;
#47099=DIRECTION ( 'NONE',  ( -1.000000000000000000, 0.000000000000000000, -0.000000000000000000 ) ) ;
#47101=ORIENTED_EDGE ( 'NONE', *, *, #43259, .T. ) ;
#47102=PLANE ( 'NONE',  #32354 ) ;
#47107=DIRECTION ( 'NONE',  ( -0.000000000000000000, 0.3546048870425463906, 0.9350162426854107256 ) ) ;
#47109=DIRECTION ( 'NONE',  ( 1.000000000000000000, 0.000000000000000000, 0.000000000000000000 ) ) ;
#47111=FACE_OUTER_BOUND ( 'NONE', #44438, .T. ) ;
#47115=DIRECTION ( 'NONE',  ( -1.000000000000000000, 0.000000000000000000, 0.000000000000000000 ) ) ;
#47118=DIRECTION ( 'NONE',  ( -0.000000000000000000, 0.000000000000000000, 1.000000000000000000 ) ) ;
#47122=FACE_OUTER_BOUND ( 'NONE', #43267, .T. ) ;
#47124=DIRECTION ( 'NONE',  ( -1.000000000000000000, 0.000000000000000000, -0.000000000000000000 ) ) ;
#47127=CARTESIAN_POINT ( 'NONE',  ( -332.3517673607765914, -87.81784868886214213, 47.06073758877343494 ) ) ;
#47132=EDGE_CURVE ( 'NONE', #9298, #50508, #39443, .T. ) ;
#47133=ADVANCED_FACE ( 'NONE', ( #51548 ), #12367, .F. ) ;
#47138=EDGE_LOOP ( 'NONE', ( #1646, #20718, #17643, #44323 ) ) ;
#47140=EDGE_CURVE ( 'NONE', #14358, #49982, #27628, .T. ) ;
#47145=VECTOR ( 'NONE', #26936, 1000.000000000000000 ) ;
#47146=ADVANCED_FACE ( 'NONE', ( #4496 ), #23439, .F. ) ;
#47148=DIRECTION ( 'NONE',  ( 0.000000000000000000, 0.6631226582408039638, 0.7485107481710934207 ) ) ;
#47149=CIRCLE ( 'NONE', #35386, 60.00000000000000000 ) ;
#47150=ORIENTED_EDGE ( 'NONE', *, *, #2093, .F. ) ;
#47151=ORIENTED_EDGE ( 'NONE', *, *, #16722, .F. ) ;
#47155=EDGE_CURVE ( 'NONE', #14073, #21253, #19730, .T. ) ;
#47156=CARTESIAN_POINT ( 'NONE',  ( -330.4913330509368166, -123.0000000000002700, -59.00000000000002132 ) ) ;
#47161=FACE_BOUND ( 'NONE', #36278, .T. ) ;
#47164=DIRECTION ( 'NONE',  ( 1.043714542225393381E-14, -0.7485107481710977506, 0.6631226582407989678 ) ) ;
#47172=FACE_OUTER_BOUND ( 'NONE', #45588, .T. ) ;
#47180=DIRECTION ( 'NONE',  ( -1.000000000000000000, 0.000000000000000000, 0.000000000000000000 ) ) ;
#47182=AXIS2_PLACEMENT_3D ( 'NONE', #42827, #30481, #26536 ) ;
#47190=EDGE_CURVE ( 'NONE', #32138, #48781, #45237, .T. ) ;
#47192=CARTESIAN_POINT ( 'NONE',  ( -339.1964088526558498, -115.7716958700755470, -59.50019592636139265 ) ) ;
#47197=VERTEX_POINT ( 'NONE', #1839 ) ;
#47202=AXIS2_PLACEMENT_3D ( 'NONE', #11047, #23157, #3181 ) ;
#47205=CARTESIAN_POINT ( 'NONE',  ( -305.0000000000000568, -151.8251501453684682, -52.89315522109013301 ) ) ;
#47210=CARTESIAN_POINT ( 'NONE',  ( -330.4913330509368166, -178.4886558749180949, 21.38919645685269444 ) ) ;
#47211=ORIENTED_EDGE ( 'NONE', *, *, #19492, .F. ) ;
#47214=DIRECTION ( 'NONE',  ( -0.000000000000000000, -0.2393156642875482742, 0.9709418174260544543 ) ) ;
#47220=CARTESIAN_POINT ( 'NONE',  ( -336.3521761649654422, -123.5000000000000284, 0.000000000000000000 ) ) ;
#47223=DIRECTION ( 'NONE',  ( 0.000000000000000000, 0.8854560256532093554, -0.4647231720437695057 ) ) ;
#47225=CARTESIAN_POINT ( 'NONE',  ( -330.4913330509368166, -66.09477493971917283, -13.63415328425296202 ) ) ;
#47226=VECTOR ( 'NONE', #17064, 1000.000000000000000 ) ;
#47232=ORIENTED_EDGE ( 'NONE', *, *, #42625, .T. ) ;
#47249=CARTESIAN_POINT ( 'NONE',  ( -339.1964088526558498, -109.8658467157473666, -57.40522506028092664 ) ) ;
#47250=VECTOR ( 'NONE', #33739, 999.9999999999998863 ) ;
#47259=CARTESIAN_POINT ( 'NONE',  ( -330.4913330509368166, -144.8891964568525452, -54.98865587491815177 ) ) ;
#47260=DIRECTION ( 'NONE',  ( -0.000000000000000000, -0.3546048870425363986, -0.9350162426854146114 ) ) ;
#47261=VERTEX_POINT ( 'NONE', #1323 ) ;
#47265=ADVANCED_FACE ( 'NONE', ( #37598 ), #28647, .F. ) ;
#47267=EDGE_CURVE ( 'NONE', #38315, #46519, #47032, .T. ) ;
#47270=AXIS2_PLACEMENT_3D ( 'NONE', #1953, #3252, #15333 ) ;
#47271=DIRECTION ( 'NONE',  ( 1.000000000000000000, 0.000000000000000000, 0.000000000000000000 ) ) ;
#47279=VERTEX_POINT ( 'NONE', #22328 ) ;
#47287=FACE_OUTER_BOUND ( 'NONE', #46455, .T. ) ;
#47289=PLANE ( 'NONE',  #36763 ) ;
#47291=ORIENTED_EDGE ( 'NONE', *, *, #35933, .F. ) ;
#47292=CARTESIAN_POINT ( 'NONE',  ( -339.1964088526558498, -115.8919814278871598, -58.50955523165758621 ) ) ;
#47295=CIRCLE ( 'NONE', #27126, 60.00000000000000000 ) ;
#47298=EDGE_LOOP ( 'NONE', ( #18465, #21013, #15685, #10371 ) ) ;
#47300=DIRECTION ( 'NONE',  ( 0.000000000000000000, -0.3546048870425300148, 0.9350162426854169428 ) ) ;
#47305=DIRECTION ( 'NONE',  ( 1.000000000000000000, -0.000000000000000000, -0.000000000000000000 ) ) ;
#47308=DIRECTION ( 'NONE',  ( -1.000000000000000000, -0.000000000000000000, 0.000000000000000000 ) ) ;
#47309=CARTESIAN_POINT ( 'NONE',  ( -336.3521761649654422, -123.5000000000000284, 0.000000000000000000 ) ) ;
#47319=VECTOR ( 'NONE', #39334, 1000.000000000000000 ) ;
#47321=CARTESIAN_POINT ( 'NONE',  ( -339.1964088526558498, -74.65991953890826949, 33.10432812419072945 ) ) ;
#47323=LINE ( 'NONE', #19205, #22413 ) ;
#47333=CARTESIAN_POINT ( 'NONE',  ( -305.0000000000000568, -138.3439121830097633, -58.13482838284718923 ) ) ;
#47334=AXIS2_PLACEMENT_3D ( 'NONE', #15712, #28542, #20152 ) ;
#47335=ORIENTED_EDGE ( 'NONE', *, *, #45131, .F. ) ;
#47338=EDGE_CURVE ( 'NONE', #16187, #1636, #38614, .T. ) ;
#47339=DIRECTION ( 'NONE',  ( 1.000000000000000000, 0.000000000000000000, 0.000000000000000000 ) ) ;
#47343=DIRECTION ( 'NONE',  ( -8.718379230999705894E-17, -0.9350162426854107256, 0.3546048870425463906 ) ) ;
#47344=CARTESIAN_POINT ( 'NONE',  ( -332.3517673607765914, -146.2946350401741711, -55.50139289590186564 ) ) ;
#47353=LINE ( 'NONE', #51300, #15428 ) ;
#47357=PLANE ( 'NONE',  #20622 ) ;
#47363=CARTESIAN_POINT ( 'NONE',  ( -339.1964088526558498, -137.1341532842523065, 57.40522506028101901 ) ) ;
#47364=VECTOR ( 'NONE', #8127, 1000.000000000000000 ) ;
#47367=CARTESIAN_POINT ( 'NONE',  ( -330.4913330509368166, -123.9999999999993747, 59.00000000000002132 ) ) ;
#47373=CARTESIAN_POINT ( 'NONE',  ( -339.1964088526558498, -123.5000000000000284, 0.000000000000000000 ) ) ;
#47374=CARTESIAN_POINT ( 'NONE',  ( -339.1964088526558498, -130.1153096980144426, 58.63009191191295599 ) ) ;
#47382=ADVANCED_FACE ( 'NONE', ( #6308 ), #42042, .F. ) ;
#47390=ORIENTED_EDGE ( 'NONE', *, *, #7681, .F. ) ;
#47392=LINE ( 'NONE', #11120, #12207 ) ;
#47393=ORIENTED_EDGE ( 'NONE', *, *, #51670, .T. ) ;
#47394=EDGE_CURVE ( 'NONE', #12850, #21974, #34419, .T. ) ;
#47395=CARTESIAN_POINT ( 'NONE',  ( -332.3517673607765914, -88.64083255475578937, 47.62880233550460218 ) ) ;
#47397=AXIS2_PLACEMENT_3D ( 'NONE', #1598, #45740, #10003 ) ;
#47402=ORIENTED_EDGE ( 'NONE', *, *, #10225, .T. ) ;
#47407=CARTESIAN_POINT ( 'NONE',  ( -330.4913330509368166, -75.22798428563987727, -33.92731199008506593 ) ) ;
#47411=AXIS2_PLACEMENT_3D ( 'NONE', #21095, #37119, #25302 ) ;
#47423=DIRECTION ( 'NONE',  ( -0.000000000000000000, -0.8854560256532062468, 0.4647231720437755564 ) ) ;
#47424=ORIENTED_EDGE ( 'NONE', *, *, #24215, .T. ) ;
#47429=VECTOR ( 'NONE', #22159, 1000.000000000000000 ) ;
#47439=VECTOR ( 'NONE', #19335, 1000.000000000000114 ) ;
#47441=PLANE ( 'NONE',  #30323 ) ;
#47443=EDGE_LOOP ( 'NONE', ( #7591, #28027, #46438, #44921 ) ) ;
#47447=FACE_OUTER_BOUND ( 'NONE', #50382, .T. ) ;
#47449=CIRCLE ( 'NONE', #12994, 60.00000000000000000 ) ;
#47450=EDGE_CURVE ( 'NONE', #35955, #44388, #16371, .T. ) ;
#47461=CARTESIAN_POINT ( 'NONE',  ( -330.4913330509368166, -175.9742670995615015, -26.97593913775547136 ) ) ;
#47463=ORIENTED_EDGE ( 'NONE', *, *, #4774, .F. ) ;
#47465=ORIENTED_EDGE ( 'NONE', *, *, #9538, .T. ) ;
#47468=VECTOR ( 'NONE', #16340, 1000.000000000000000 ) ;
#47481=ORIENTED_EDGE ( 'NONE', *, *, #13450, .F. ) ;
#47484=PLANE ( 'NONE',  #35025 ) ;
#47488=ADVANCED_FACE ( 'NONE', ( #7351 ), #3918, .F. ) ;
#47499=LINE ( 'NONE', #40553, #9651 ) ;
#47502=PLANE ( 'NONE',  #1285 ) ;
#47508=LINE ( 'NONE', #43559, #27382 ) ;
#47510=DIRECTION ( 'NONE',  ( 0.000000000000000000, -0.4647231720437573488, 0.8854560256532157947 ) ) ;
#47517=CARTESIAN_POINT ( 'NONE',  ( -336.3521761649654422, -160.6539403396202772, 45.90766452162722544 ) ) ;
#47521=VERTEX_POINT ( 'NONE', #216 ) ;
#47527=ORIENTED_EDGE ( 'NONE', *, *, #24142, .F. ) ;
#47528=VECTOR ( 'NONE', #30304, 1000.000000000000000 ) ;
#47532=EDGE_CURVE ( 'NONE', #23663, #28688, #51489, .T. ) ;
#47535=ORIENTED_EDGE ( 'NONE', *, *, #13800, .T. ) ;
#47538=VERTEX_POINT ( 'NONE', #51754 ) ;
#47540=CARTESIAN_POINT ( 'NONE',  ( 0.000000000000000000, -172.0560480877254861, 33.51582005713859758 ) ) ;
#47544=CARTESIAN_POINT ( 'NONE',  ( -339.1964088526558498, -178.4886558749184076, -21.38919645685194837 ) ) ;
#47545=EDGE_LOOP ( 'NONE', ( #40557, #28533, #8236, #37848 ) ) ;
#47546=VECTOR ( 'NONE', #8841, 1000.000000000000000 ) ;
#47551=ORIENTED_EDGE ( 'NONE', *, *, #2231, .T. ) ;
#47552=VECTOR ( 'NONE', #8443, 1000.000000000000000 ) ;
#47556=VERTEX_POINT ( 'NONE', #40410 ) ;
#47558=CARTESIAN_POINT ( 'NONE',  ( -336.3521761649654422, -182.5000000000000568, 2.632288850093980503 ) ) ;
#47559=ORIENTED_EDGE ( 'NONE', *, *, #22482, .F. ) ;
#47560=ADVANCED_FACE ( 'NONE', ( #31499 ), #15228, .F. ) ;
#47561=EDGE_CURVE ( 'NONE', #26366, #4036, #12571, .T. ) ;
#47563=ORIENTED_EDGE ( 'NONE', *, *, #3741, .T. ) ;
#47567=AXIS2_PLACEMENT_3D ( 'NONE', #39143, #46530, #3153 ) ;
#47568=DIRECTION ( 'NONE',  ( 0.000000000000000000, 0.000000000000000000, 1.000000000000000000 ) ) ;
#47574=VERTEX_POINT ( 'NONE', #17311 ) ;
#47579=LINE ( 'NONE', #11562, #41366 ) ;
#47581=DIRECTION ( 'NONE',  ( -0.000000000000000000, 0.5680647467311656929, 0.8229838658936495799 ) ) ;
#47587=VERTEX_POINT ( 'NONE', #13608 ) ;
#47594=LINE ( 'NONE', #44146, #29578 ) ;
#47595=LINE ( 'NONE', #18439, #21196 ) ;
#47600=AXIS2_PLACEMENT_3D ( 'NONE', #21160, #37186, #45611 ) ;
#47602=VECTOR ( 'NONE', #8233, 1000.000000000000000 ) ;
#47607=PLANE ( 'NONE',  #21986 ) ;
#47610=AXIS2_PLACEMENT_3D ( 'NONE', #1842, #37327, #17885 ) ;
#47611=DIRECTION ( 'NONE',  ( -1.000000000000000000, 0.000000000000000000, -0.000000000000000000 ) ) ;
#47612=DIRECTION ( 'NONE',  ( 0.000000000000000000, -0.8229838658936596829, -0.5680647467311510379 ) ) ;
#47614=DIRECTION ( 'NONE',  ( 1.000000000000000000, -8.151826190875865775E-17, 3.091579882402733311E-17 ) ) ;
#47617=ORIENTED_EDGE ( 'NONE', *, *, #35796, .T. ) ;
#47618=CARTESIAN_POINT ( 'NONE',  ( -339.1964088526558498, -150.4759391377552618, 52.47426709956155122 ) ) ;
#47623=PLANE ( 'NONE',  #10652 ) ;
#47624=CARTESIAN_POINT ( 'NONE',  ( -330.4913330509368166, -167.9936954712156023, -38.74998146212117689 ) ) ;
#47625=ORIENTED_EDGE ( 'NONE', *, *, #38496, .F. ) ;
#47627=DIRECTION ( 'NONE',  ( -0.000000000000000000, 0.4647231720437789981, 0.8854560256532044704 ) ) ;
#47628=AXIS2_PLACEMENT_3D ( 'NONE', #25794, #42073, #21603 ) ;
#47633=EDGE_LOOP ( 'NONE', ( #51506, #18217, #26164, #46391 ) ) ;
#47635=PLANE ( 'NONE',  #35674 ) ;
#47636=FACE_OUTER_BOUND ( 'NONE', #47298, .T. ) ;
#47645=ADVANCED_FACE ( 'NONE', ( #5484 ), #5225, .T. ) ;
#47649=CARTESIAN_POINT ( 'NONE',  ( -332.3517673607765914, -132.3499116637027271, -59.34373651485605450 ) ) ;
#47652=CIRCLE ( 'NONE', #3969, 60.00000000000000000 ) ;
#47653=CARTESIAN_POINT ( 'NONE',  ( -332.3517673607765914, -119.0014323656137947, -58.88711093124865670 ) ) ;
#47654=CARTESIAN_POINT ( 'NONE',  ( -330.4913330509368166, -167.3305728129743102, 39.49849221029282376 ) ) ;
#47657=EDGE_LOOP ( 'NONE', ( #40922, #27855, #9907, #35636 ) ) ;
#47658=DIRECTION ( 'NONE',  ( -1.000000000000000000, 0.000000000000000000, -0.000000000000000000 ) ) ;
#47661=ORIENTED_EDGE ( 'NONE', *, *, #12101, .T. ) ;
#47664=EDGE_LOOP ( 'NONE', ( #51960, #30594, #5667, #4699 ) ) ;
#47668=DIRECTION ( 'NONE',  ( -0.000000000000000000, 0.8229838658936634577, 0.5680647467311457088 ) ) ;
#47672=ORIENTED_EDGE ( 'NONE', *, *, #18012, .F. ) ;
#47674=EDGE_LOOP ( 'NONE', ( #9105, #33536, #25444, #38134 ) ) ;
#47676=DIRECTION ( 'NONE',  ( 0.000000000000000000, 0.000000000000000000, -1.000000000000000000 ) ) ;
#47678=LINE ( 'NONE', #23742, #12316 ) ;
#47681=VERTEX_POINT ( 'NONE', #20719 ) ;
#47683=EDGE_CURVE ( 'NONE', #21742, #23268, #39010, .T. ) ;
#47686=VECTOR ( 'NONE', #7342, 1000.000000000000000 ) ;
#47694=LINE ( 'NONE', #19052, #37583 ) ;
#47695=CARTESIAN_POINT ( 'NONE',  ( -336.3521761649654422, -164.5945333327934463, -42.41660376256285048 ) ) ;
#47697=ORIENTED_EDGE ( 'NONE', *, *, #48310, .F. ) ;
#47700=CARTESIAN_POINT ( 'NONE',  ( -339.1964088526558498, -130.1153096980153236, -58.63009191191284941 ) ) ;
#47704=ADVANCED_FACE ( 'NONE', ( #32546 ), #48851, .F. ) ;
#47707=LINE ( 'NONE', #7745, #36595 ) ;
#47708=PLANE ( 'NONE',  #51565 ) ;
#47714=ORIENTED_EDGE ( 'NONE', *, *, #40547, .T. ) ;
#47721=DIRECTION ( 'NONE',  ( -1.000000000000000000, 0.000000000000000000, -1.043714542225393381E-14 ) ) ;
#47724=ORIENTED_EDGE ( 'NONE', *, *, #42332, .F. ) ;
#47725=FACE_OUTER_BOUND ( 'NONE', #35345, .T. ) ;
#47726=CARTESIAN_POINT ( 'NONE',  ( -330.4913330509368166, -95.63860483659122735, -52.00954392751761191 ) ) ;
#47727=VERTEX_POINT ( 'NONE', #28846 ) ;
#47730=ADVANCED_FACE ( 'NONE', ( #24927 ), #17573, .F. ) ;
#47731=EDGE_CURVE ( 'NONE', #13383, #40543, #33056, .T. ) ;
#47735=ORIENTED_EDGE ( 'NONE', *, *, #36557, .T. ) ;
#47740=CARTESIAN_POINT ( 'NONE',  ( -339.1964088526558498, -123.5000000000000284, 0.000000000000000000 ) ) ;
#47741=DIRECTION ( 'NONE',  ( 0.000000000000000000, 0.6631226582408039638, 0.7485107481710934207 ) ) ;
#47744=AXIS2_PLACEMENT_3D ( 'NONE', #19403, #24143, #27794 ) ;
#47745=ADVANCED_FACE ( 'NONE', ( #20450 ), #36470, .F. ) ;
#47746=EDGE_CURVE ( 'NONE', #48787, #4433, #28091, .T. ) ;
#47748=ORIENTED_EDGE ( 'NONE', *, *, #14943, .F. ) ;
#47752=ORIENTED_EDGE ( 'NONE', *, *, #36497, .F. ) ;
#47754=DIRECTION ( 'NONE',  ( -0.000000000000000000, -1.000000000000000000, -0.000000000000000000 ) ) ;
#47755=PLANE ( 'NONE',  #10719 ) ;
#47761=VERTEX_POINT ( 'NONE', #19553 ) ;
#47763=ORIENTED_EDGE ( 'NONE', *, *, #49747, .T. ) ;
#47765=FACE_OUTER_BOUND ( 'NONE', #2291, .T. ) ;
#47766=PLANE ( 'NONE',  #16372 ) ;
#47773=EDGE_LOOP ( 'NONE', ( #32181, #9423, #34067, #14506 ) ) ;
#47774=AXIS2_PLACEMENT_3D ( 'NONE', #38332, #10987, #26497 ) ;
#47782=CARTESIAN_POINT ( 'NONE',  ( -339.1964088526558498, -68.15673923803930734, -20.45418021416698551 ) ) ;
#47789=PLANE ( 'NONE',  #16830 ) ;
#47790=ORIENTED_EDGE ( 'NONE', *, *, #6, .T. ) ;
#47795=ORIENTED_EDGE ( 'NONE', *, *, #21076, .F. ) ;
#47799=LINE ( 'NONE', #4169, #41437 ) ;
#47807=ORIENTED_EDGE ( 'NONE', *, *, #9274, .F. ) ;
#47808=EDGE_CURVE ( 'NONE', #19701, #30167, #42949, .T. ) ;
#47810=CARTESIAN_POINT ( 'NONE',  ( -336.3521761649654422, -65.12692710742291524, -8.732051761643681687 ) ) ;
#47814=EDGE_CURVE ( 'NONE', #35764, #12660, #15545, .T. ) ;
#47819=ORIENTED_EDGE ( 'NONE', *, *, #15703, .F. ) ;
#47823=LINE ( 'NONE', #32281, #42170 ) ;
#47834=VECTOR ( 'NONE', #37764, 1000.000000000000000 ) ;
#47838=CARTESIAN_POINT ( 'NONE',  ( -336.3521761649654422, -123.5000000000000284, 0.000000000000000000 ) ) ;
#47841=ORIENTED_EDGE ( 'NONE', *, *, #34001, .F. ) ;
#47842=ORIENTED_EDGE ( 'NONE', *, *, #26832, .T. ) ;
#47847=CARTESIAN_POINT ( 'NONE',  ( -339.1964088526558498, -123.5000000000000284, 0.000000000000000000 ) ) ;
#47848=CARTESIAN_POINT ( 'NONE',  ( -336.3521761649654422, -128.1121410293017391, 59.82247199109905011 ) ) ;
#47849=DIRECTION ( 'NONE',  ( 1.000000000000000000, -0.000000000000000000, -0.000000000000000000 ) ) ;
#47853=EDGE_CURVE ( 'NONE', #16896, #2635, #28203, .T. ) ;
#47856=VERTEX_POINT ( 'NONE', #32412 ) ;
#47859=DIRECTION ( 'NONE',  ( -0.000000000000000000, -0.2393156642875482742, 0.9709418174260544543 ) ) ;
#47866=DIRECTION ( 'NONE',  ( 0.000000000000000000, -0.6631226582407989678, -0.7485107481710977506 ) ) ;
#47867=EDGE_LOOP ( 'NONE', ( #12352, #27416, #16641, #504 ) ) ;
#47869=DIRECTION ( 'NONE',  ( -1.000000000000000000, -0.000000000000000000, 0.000000000000000000 ) ) ;
#47872=ORIENTED_EDGE ( 'NONE', *, *, #46499, .T. ) ;
#47874=DIRECTION ( 'NONE',  ( 0.000000000000000000, -0.9350162426854194964, -0.3546048870425235200 ) ) ;
#47880=CARTESIAN_POINT ( 'NONE',  ( -339.1964088526558498, -90.39567187580880159, -48.84008046109142498 ) ) ;
#47882=VECTOR ( 'NONE', #23088, 1000.000000000000000 ) ;
#47883=ORIENTED_EDGE ( 'NONE', *, *, #8354, .F. ) ;
#47889=CARTESIAN_POINT ( 'NONE',  ( -339.1964088526558498, -64.86990808808704401, 6.615309698014191220 ) ) ;
#47890=ORIENTED_EDGE ( 'NONE', *, *, #27888, .F. ) ;
#47896=LINE ( 'NONE', #39473, #36506 ) ;
#47897=LINE ( 'NONE', #16351, #39976 ) ;
#47899=VECTOR ( 'NONE', #8142, 1000.000000000000000 ) ;
#47901=CARTESIAN_POINT ( 'NONE',  ( -330.4913330509368166, -123.5000000000000284, 0.000000000000000000 ) ) ;
#47906=ADVANCED_FACE ( 'NONE', ( #873 ), #12441, .F. ) ;
#47910=VERTEX_POINT ( 'NONE', #35840 ) ;
#47915=DIRECTION ( 'NONE',  ( -1.000000000000000000, 0.000000000000000000, 0.000000000000000000 ) ) ;
#47919=EDGE_LOOP ( 'NONE', ( #32522, #49828, #21772, #23902 ) ) ;
#47920=ORIENTED_EDGE ( 'NONE', *, *, #41098, .F. ) ;
#47932=LINE ( 'NONE', #20857, #18165 ) ;
#47934=AXIS2_PLACEMENT_3D ( 'NONE', #48287, #28303, #31982 ) ;
#47936=EDGE_LOOP ( 'NONE', ( #23960, #20086, #50181, #25673 ) ) ;
#47937=ORIENTED_EDGE ( 'NONE', *, *, #5735, .T. ) ;
#47941=FACE_OUTER_BOUND ( 'NONE', #893, .T. ) ;
#47942=CARTESIAN_POINT ( 'NONE',  ( -339.1964088526558498, -167.3305728129742249, 39.49849221029288060 ) ) ;
#47943=CARTESIAN_POINT ( 'NONE',  ( -336.3521761649654422, -94.63601285149479736, 51.48334306143172512 ) ) ;
#47945=DIRECTION ( 'NONE',  ( 0.000000000000000000, 0.000000000000000000, -1.000000000000000000 ) ) ;
#47946=ORIENTED_EDGE ( 'NONE', *, *, #5318, .T. ) ;
#47948=PLANE ( 'NONE',  #7813 ) ;
#47952=DIRECTION ( 'NONE',  ( -1.000000000000000000, -0.000000000000000000, 0.000000000000000000 ) ) ;
#47957=ORIENTED_EDGE ( 'NONE', *, *, #13820, .F. ) ;
#47960=ORIENTED_EDGE ( 'NONE', *, *, #11988, .F. ) ;
#47974=PLANE ( 'NONE',  #178 ) ;
#47975=ORIENTED_EDGE ( 'NONE', *, *, #12422, .F. ) ;
#47976=CARTESIAN_POINT ( 'NONE',  ( -340.0000000000000568, -78.50000000000002842, 0.000000000000000000 ) ) ;
#47980=VERTEX_POINT ( 'NONE', #36619 ) ;
#47982=EDGE_LOOP ( 'NONE', ( #45300, #37769, #19138, #7401 ) ) ;
#47983=ORIENTED_EDGE ( 'NONE', *, *, #559, .F. ) ;
#47984=DIRECTION ( 'NONE',  ( -0.000000000000000000, 0.2393156642875547968, -0.9709418174260527890 ) ) ;
#47985=DIRECTION ( 'NONE',  ( 0.000000000000000000, -0.4647231720437725033, -0.8854560256532079121 ) ) ;
#47986=CIRCLE ( 'NONE', #27820, 5.000000000000001776 ) ;
#47990=LINE ( 'NONE', #44317, #356 ) ;
#47994=DIRECTION ( 'NONE',  ( 0.000000000000000000, -0.7485107481710934207, 0.6631226582408039638 ) ) ;
#47998=DIRECTION ( 'NONE',  ( 0.000000000000000000, -0.3546048870425396182, -0.9350162426854132791 ) ) ;
#48001=FACE_OUTER_BOUND ( 'NONE', #43826, .T. ) ;
#48005=ORIENTED_EDGE ( 'NONE', *, *, #44570, .T. ) ;
#48007=ORIENTED_EDGE ( 'NONE', *, *, #11964, .T. ) ;
#48014=EDGE_LOOP ( 'NONE', ( #44151, #15803, #5189, #9337 ) ) ;
#48017=VECTOR ( 'NONE', #25342, 1000.000000000000114 ) ;
#48021=AXIS2_PLACEMENT_3D ( 'NONE', #6105, #10294, #6355 ) ;
#48022=AXIS2_PLACEMENT_3D ( 'NONE', #18517, #2491, #11388 ) ;
#48026=DIRECTION ( 'NONE',  ( 1.000000000000000000, 4.051632851310703470E-17, 7.719741424018482920E-17 ) ) ;
#48029=EDGE_CURVE ( 'NONE', #2635, #186, #13487, .T. ) ;
#48035=ORIENTED_EDGE ( 'NONE', *, *, #37704, .T. ) ;
#48040=ORIENTED_EDGE ( 'NONE', *, *, #45542, .T. ) ;
#48042=ORIENTED_EDGE ( 'NONE', *, *, #38224, .T. ) ;
#48044=CARTESIAN_POINT ( 'NONE',  ( -336.3521761649654422, -69.26746417191145611, -23.38292116578723068 ) ) ;
#48049=ORIENTED_EDGE ( 'NONE', *, *, #20803, .F. ) ;
#48057=VERTEX_POINT ( 'NONE', #49238 ) ;
#48058=DIRECTION ( 'NONE',  ( 1.000000000000000000, -0.000000000000000000, -0.000000000000000000 ) ) ;
#48063=DIRECTION ( 'NONE',  ( 0.000000000000000000, -0.4647231720437789981, -0.8854560256532044704 ) ) ;
#48073=LINE ( 'NONE', #20466, #38975 ) ;
#48075=ADVANCED_FACE ( 'NONE', ( #45559 ), #21897, .F. ) ;
#48081=AXIS2_PLACEMENT_3D ( 'NONE', #43384, #7390, #44422 ) ;
#48083=ORIENTED_EDGE ( 'NONE', *, *, #27561, .T. ) ;
#48087=LINE ( 'NONE', #8402, #48450 ) ;
#48089=ORIENTED_EDGE ( 'NONE', *, *, #34978, .T. ) ;
#48090=EDGE_CURVE ( 'NONE', #26719, #15605, #5618, .T. ) ;
#48091=VECTOR ( 'NONE', #16031, 1000.000000000000227 ) ;
#48092=EDGE_LOOP ( 'NONE', ( #41737, #46142, #41057, #11383 ) ) ;
#48093=VECTOR ( 'NONE', #2848, 1000.000000000000000 ) ;
#48094=EDGE_CURVE ( 'NONE', #15388, #33963, #35717, .T. ) ;
#48102=EDGE_LOOP ( 'NONE', ( #24773, #9501, #28082, #47890 ) ) ;
#48103=VECTOR ( 'NONE', #17018, 1000.000000000000000 ) ;
#48108=ORIENTED_EDGE ( 'NONE', *, *, #29462, .F. ) ;
#48114=LINE ( 'NONE', #39681, #30062 ) ;
#48115=CARTESIAN_POINT ( 'NONE',  ( -336.3521761649654422, -85.59754891220836726, -45.24454186338619621 ) ) ;
#48117=PLANE ( 'NONE',  #17416 ) ;
#48124=LINE ( 'NONE', #35767, #28821 ) ;
#48129=EDGE_CURVE ( 'NONE', #21574, #30158, #12952, .T. ) ;
#48131=VECTOR ( 'NONE', #15697, 1000.000000000000000 ) ;
#48138=EDGE_CURVE ( 'NONE', #40953, #978, #19249, .T. ) ;
#48144=LINE ( 'NONE', #12115, #10504 ) ;
#48146=ORIENTED_EDGE ( 'NONE', *, *, #32332, .T. ) ;
#48159=DIRECTION ( 'NONE',  ( 1.000000000000000000, -0.000000000000000000, -0.000000000000000000 ) ) ;
#48160=EDGE_CURVE ( 'NONE', #47261, #16316, #50789, .T. ) ;
#48164=VERTEX_POINT ( 'NONE', #18466 ) ;
#48171=ORIENTED_EDGE ( 'NONE', *, *, #33962, .T. ) ;
#48175=CARTESIAN_POINT ( 'NONE',  ( -330.4913330509368166, -150.4759391377553186, 52.47426709956150859 ) ) ;
#48176=FACE_OUTER_BOUND ( 'NONE', #27154, .T. ) ;
#48178=EDGE_LOOP ( 'NONE', ( #36267, #7598, #11900, #41919 ) ) ;
#48185=CARTESIAN_POINT ( 'NONE',  ( -330.4913330509368166, -182.0095552316575152, 7.608018572113473432 ) ) ;
#48186=LINE ( 'NONE', #12156, #14497 ) ;
#48191=VECTOR ( 'NONE', #49635, 1000.000000000000000 ) ;
#48194=CARTESIAN_POINT ( 'NONE',  ( -339.1964088526558498, -123.5000000000000284, 0.000000000000000000 ) ) ;
#48196=EDGE_LOOP ( 'NONE', ( #20965, #13853, #50661, #15266 ) ) ;
#48198=VERTEX_POINT ( 'NONE', #6893 ) ;
#48206=EDGE_CURVE ( 'NONE', #37592, #13526, #10573, .T. ) ;
#48208=CARTESIAN_POINT ( 'NONE',  ( -339.1964088526558498, -182.0095552316575152, 7.608018572113563138 ) ) ;
#48218=CARTESIAN_POINT ( 'NONE',  ( -332.3517673607765914, -120.8677111499054320, 59.00000000000000000 ) ) ;
#48220=DIRECTION ( 'NONE',  ( -1.000000000000000000, 0.000000000000000000, -0.000000000000000000 ) ) ;
#48221=ORIENTED_EDGE ( 'NONE', *, *, #35267, .T. ) ;
#48222=DIRECTION ( 'NONE',  ( 0.000000000000000000, 0.000000000000000000, 1.000000000000000000 ) ) ;
#48223=VERTEX_POINT ( 'NONE', #18985 ) ;
#48229=AXIS2_PLACEMENT_3D ( 'NONE', #47618, #15820, #28124 ) ;
#48232=CARTESIAN_POINT ( 'NONE',  ( -330.4913330509368166, -172.3400804610915031, -33.10432812419114157 ) ) ;
#48236=ORIENTED_EDGE ( 'NONE', *, *, #29562, .T. ) ;
#48237=LINE ( 'NONE', #28246, #50794 ) ;
#48250=FACE_BOUND ( 'NONE', #1930, .T. ) ;
#48252=VERTEX_POINT ( 'NONE', #8702 ) ;
#48255=ORIENTED_EDGE ( 'NONE', *, *, #50726, .F. ) ;
#48267=ORIENTED_EDGE ( 'NONE', *, *, #43952, .T. ) ;
#48272=LINE ( 'NONE', #43288, #16087 ) ;
#48280=CARTESIAN_POINT ( 'NONE',  ( -330.4913330509368166, -123.5000000000000142, 60.00000000000000000 ) ) ;
#48282=VECTOR ( 'NONE', #34412, 1000.000000000000000 ) ;
#48284=EDGE_LOOP ( 'NONE', ( #47714, #18099, #13950, #3319 ) ) ;
#48287=CARTESIAN_POINT ( 'NONE',  ( 0.000000000000000000, -89.98417994286192823, -48.55604808772582004 ) ) ;
#48290=ORIENTED_EDGE ( 'NONE', *, *, #47683, .F. ) ;
#48297=EDGE_CURVE ( 'NONE', #51884, #17654, #33246, .T. ) ;
#48298=CARTESIAN_POINT ( 'NONE',  ( -332.3517673607765914, -159.1821513111375452, -47.06073758877369073 ) ) ;
#48305=VECTOR ( 'NONE', #35376, 999.9999999999998863 ) ;
#48310=EDGE_CURVE ( 'NONE', #33612, #4373, #1335, .T. ) ;
#48311=CIRCLE ( 'NONE', #19752, 60.00000000000000000 ) ;
#48313=LINE ( 'NONE', #12294, #39028 ) ;
#48316=CARTESIAN_POINT ( 'NONE',  ( -332.3517673607765914, -106.8245764869328980, 56.65561927337994064 ) ) ;
#48319=LINE ( 'NONE', #16795, #7195 ) ;
#48322=ORIENTED_EDGE ( 'NONE', *, *, #49101, .F. ) ;
#48327=DIRECTION ( 'NONE',  ( 1.043714542225393223E-14, -0.9927088740980544168, -0.1205366802553199113 ) ) ;
#48328=EDGE_LOOP ( 'NONE', ( #42931, #7344, #46371, #9512 ) ) ;
#48336=CARTESIAN_POINT ( 'NONE',  ( -330.4913330509368166, -68.15673923803900891, 20.45418021416622878 ) ) ;
#48338=VECTOR ( 'NONE', #40747, 999.9999999999998863 ) ;
#48340=VECTOR ( 'NONE', #47581, 1000.000000000000114 ) ;
#48342=CARTESIAN_POINT ( 'NONE',  ( 0.000000000000000000, -68.33404168156053515, -20.92168833550964990 ) ) ;
#48348=EDGE_CURVE ( 'NONE', #44602, #38839, #16863, .T. ) ;
#48354=VECTOR ( 'NONE', #7362, 1000.000000000000000 ) ;
#48370=ADVANCED_FACE ( 'NONE', ( #41019 ), #4769, .F. ) ;
#48377=CIRCLE ( 'NONE', #9903, 60.00000000000000000 ) ;
#48378=AXIS2_PLACEMENT_3D ( 'NONE', #21403, #45339, #37426 ) ;
#48379=VECTOR ( 'NONE', #13835, 1000.000000000000000 ) ;
#48384=EDGE_LOOP ( 'NONE', ( #51621, #35476, #1835, #30549 ) ) ;
#48387=VECTOR ( 'NONE', #670, 1000.000000000000000 ) ;
#48388=DIRECTION ( 'NONE',  ( -0.000000000000000000, -0.9709418174260502354, 0.2393156642875652051 ) ) ;
#48393=VECTOR ( 'NONE', #47099, 1000.000000000000000 ) ;
#48394=LINE ( 'NONE', #28403, #18161 ) ;
#48400=FACE_OUTER_BOUND ( 'NONE', #5552, .T. ) ;
#48406=CARTESIAN_POINT ( 'NONE',  ( -332.3517673607765914, -163.8460225846223466, -43.07972642080364523 ) ) ;
#48408=CARTESIAN_POINT ( 'NONE',  ( -305.0000000000000568, -157.9941932480463436, 49.09328500076600221 ) ) ;
#48417=CARTESIAN_POINT ( 'NONE',  ( -336.3521761649654422, -180.1556192733800117, 16.67542351306693149 ) ) ;
#48420=CIRCLE ( 'NONE', #11448, 60.00000000000000000 ) ;
#48423=LINE ( 'NONE', #20550, #23656 ) ;
#48427=FACE_OUTER_BOUND ( 'NONE', #14370, .T. ) ;
#48429=VECTOR ( 'NONE', #50469, 1000.000000000000000 ) ;
#48430=EDGE_CURVE ( 'NONE', #40405, #22679, #48665, .T. ) ;
#48435=PLANE ( 'NONE',  #21672 ) ;
#48438=ADVANCED_FACE ( 'NONE', ( #43087 ), #2884, .T. ) ;
#48449=VERTEX_POINT ( 'NONE', #46027 ) ;
#48450=VECTOR ( 'NONE', #15795, 1000.000000000000000 ) ;
#48463=ORIENTED_EDGE ( 'NONE', *, *, #39737, .F. ) ;
#48464=AXIS2_PLACEMENT_3D ( 'NONE', #31621, #44493, #47676 ) ;
#48468=DIRECTION ( 'NONE',  ( -1.000000000000000000, 0.000000000000000000, 1.043714542225393381E-14 ) ) ;
#48470=EDGE_LOOP ( 'NONE', ( #24263, #42131, #13241, #17768 ) ) ;
#48472=CIRCLE ( 'NONE', #45139, 60.00000000000000000 ) ;
#48476=DIRECTION ( 'NONE',  ( -0.000000000000000000, -0.9927088740980530845, 0.1205366802553303057 ) ) ;
#48481=ORIENTED_EDGE ( 'NONE', *, *, #35937, .T. ) ;
#48485=CARTESIAN_POINT ( 'NONE',  ( -336.3521761649654422, -159.1821513111375452, -47.06073758877369073 ) ) ;
#48490=DIRECTION ( 'NONE',  ( 0.000000000000000000, 0.6631226582407937498, -0.7485107481711024136 ) ) ;
#48493=FACE_OUTER_BOUND ( 'NONE', #5753, .T. ) ;
#48494=ORIENTED_EDGE ( 'NONE', *, *, #10450, .F. ) ;
#48496=AXIS2_PLACEMENT_3D ( 'NONE', #45045, #25835, #40810 ) ;
#48497=AXIS2_PLACEMENT_3D ( 'NONE', #16537, #44905, #20727 ) ;
#48498=CARTESIAN_POINT ( 'NONE',  ( -332.3517673607765914, -142.8954717479169574, 55.74477592174805096 ) ) ;
#48500=ORIENTED_EDGE ( 'NONE', *, *, #41879, .T. ) ;
#48501=VECTOR ( 'NONE', #11891, 999.9999999999998863 ) ;
#48502=ORIENTED_EDGE ( 'NONE', *, *, #368, .F. ) ;
#48505=DIRECTION ( 'NONE',  ( -0.000000000000000000, -0.4647231720437695057, -0.8854560256532093554 ) ) ;
#48508=DIRECTION ( 'NONE',  ( -1.000000000000000000, 0.000000000000000000, -0.000000000000000000 ) ) ;
#48509=ORIENTED_EDGE ( 'NONE', *, *, #25647, .F. ) ;
#48510=LINE ( 'NONE', #15926, #663 ) ;
#48514=ADVANCED_FACE ( 'NONE', ( #18150 ), #34177, .F. ) ;
#48515=CARTESIAN_POINT ( 'NONE',  ( -336.3521761649654422, -152.3639871485048900, -51.48334306143194539 ) ) ;
#48526=FACE_BOUND ( 'NONE', #27889, .T. ) ;
#48533=AXIS2_PLACEMENT_3D ( 'NONE', #11337, #32342, #19488 ) ;
#48537=DIRECTION ( 'NONE',  ( 1.043714542225393223E-14, -0.3546048870425363986, -0.9350162426854146114 ) ) ;
#48538=DIRECTION ( 'NONE',  ( -0.000000000000000000, 0.8229838658936556861, -0.5680647467311569221 ) ) ;
#48540=DIRECTION ( 'NONE',  ( 1.043714542225393223E-14, 0.5680647467311626952, 0.8229838658936516893 ) ) ;
#48541=DIRECTION ( 'NONE',  ( -1.000000000000000000, 0.000000000000000000, 0.000000000000000000 ) ) ;
#48551=CARTESIAN_POINT ( 'NONE',  ( -330.4913330509368166, -116.8846903019851311, -58.63009191191288494 ) ) ;
#48554=ORIENTED_EDGE ( 'NONE', *, *, #29964, .T. ) ;
#48556=DIRECTION ( 'NONE',  ( 0.000000000000000000, 0.2393156642875516049, -0.9709418174260534551 ) ) ;
#48559=ORIENTED_EDGE ( 'NONE', *, *, #34651, .T. ) ;
#48560=LINE ( 'NONE', #24616, #30649 ) ;
#48562=VERTEX_POINT ( 'NONE', #51253 ) ;
#48564=ORIENTED_EDGE ( 'NONE', *, *, #28772, .T. ) ;
#48566=CARTESIAN_POINT ( 'NONE',  ( -339.1964088526558498, -67.57827586672145515, 21.74306257088659677 ) ) ;
#48567=VECTOR ( 'NONE', #28214, 1000.000000000000000 ) ;
#48570=CARTESIAN_POINT ( 'NONE',  ( -330.4913330509368166, -65.36517161715283919, -14.84391218300977400 ) ) ;
#48573=EDGE_CURVE ( 'NONE', #6375, #19121, #8125, .T. ) ;
#48585=CARTESIAN_POINT ( 'NONE',  ( -336.3521761649653854, -164.4944191672036311, -43.81161486573634534 ) ) ;
#48589=DIRECTION ( 'NONE',  ( -1.000000000000000000, -0.000000000000000000, 0.000000000000000000 ) ) ;
#48590=ORIENTED_EDGE ( 'NONE', *, *, #13438, .T. ) ;
#48591=ORIENTED_EDGE ( 'NONE', *, *, #7030, .T. ) ;
#48601=LINE ( 'NONE', #36760, #49317 ) ;
#48605=LINE ( 'NONE', #19953, #36280 ) ;
#48606=CARTESIAN_POINT ( 'NONE',  ( -336.3521761649654422, -174.5186198893880771, 29.74944317415823392 ) ) ;
#48609=DIRECTION ( 'NONE',  ( -0.000000000000000000, 0.9350162426854146114, -0.3546048870425363986 ) ) ;
#48614=CARTESIAN_POINT ( 'NONE',  ( -339.1964088526558498, -162.9984922102927385, -43.83057281297435992 ) ) ;
#48617=FACE_OUTER_BOUND ( 'NONE', #37508, .T. ) ;
#48618=LINE ( 'NONE', #12591, #35806 ) ;
#48620=AXIS2_PLACEMENT_3D ( 'NONE', #9135, #20961, #49071 ) ;
#48627=ORIENTED_EDGE ( 'NONE', *, *, #30449, .T. ) ;
#48632=CARTESIAN_POINT ( 'NONE',  ( 0.000000000000000000, -79.33786585790457480, 39.12423683620640702 ) ) ;
#48636=ADVANCED_FACE ( 'NONE', ( #7365 ), #52035, .T. ) ;
#48642=EDGE_CURVE ( 'NONE', #36663, #2925, #23387, .T. ) ;
#48648=CARTESIAN_POINT ( 'NONE',  ( -305.0000000000000568, -116.7644047441732340, -59.62073260661667717 ) ) ;
#48649=CARTESIAN_POINT ( 'NONE',  ( -339.1964088526558498, -64.86990808808704401, 6.615309698014191220 ) ) ;
#48650=LINE ( 'NONE', #20779, #35883 ) ;
#48651=ORIENTED_EDGE ( 'NONE', *, *, #33863, .T. ) ;
#48653=FACE_OUTER_BOUND ( 'NONE', #4589, .T. ) ;
#48657=ORIENTED_EDGE ( 'NONE', *, *, #30693, .F. ) ;
#48658=PLANE ( 'NONE',  #14030 ) ;
#48664=DIRECTION ( 'NONE',  ( -1.000000000000000000, 0.000000000000000000, -0.000000000000000000 ) ) ;
#48665=LINE ( 'NONE', #28658, #49206 ) ;
#48667=DIRECTION ( 'NONE',  ( 0.000000000000000000, 0.000000000000000000, 1.000000000000000000 ) ) ;
#48671=DIRECTION ( 'NONE',  ( 1.000000000000000000, 0.000000000000000000, 0.000000000000000000 ) ) ;
#48677=DIRECTION ( 'NONE',  ( 0.000000000000000000, -7.193320013717159664E-14, 1.000000000000000000 ) ) ;
#48678=DIRECTION ( 'NONE',  ( 0.000000000000000000, 0.000000000000000000, -1.000000000000000000 ) ) ;
#48680=DIRECTION ( 'NONE',  ( -1.000000000000000000, 0.000000000000000000, -0.000000000000000000 ) ) ;
#48683=CARTESIAN_POINT ( 'NONE',  ( -332.3517673607765914, -65.58448481710581746, 11.56382487286456140 ) ) ;
#48686=ORIENTED_EDGE ( 'NONE', *, *, #31065, .T. ) ;
#48688=FACE_OUTER_BOUND ( 'NONE', #29386, .T. ) ;
#48692=CIRCLE ( 'NONE', #26025, 60.00000000000000000 ) ;
#48696=EDGE_CURVE ( 'NONE', #3020, #13909, #24018, .T. ) ;
#48697=ORIENTED_EDGE ( 'NONE', *, *, #5775, .T. ) ;
#48698=CARTESIAN_POINT ( 'NONE',  ( -336.3521761649654422, -111.9361751271348879, -57.91551518289410438 ) ) ;
#48699=DIRECTION ( 'NONE',  ( 0.000000000000000000, 0.2393156642875685913, 0.9709418174260493473 ) ) ;
#48700=DIRECTION ( 'NONE',  ( -1.000000000000000000, 9.758900497077185133E-15, 3.701062773504781726E-15 ) ) ;
#48701=ORIENTED_EDGE ( 'NONE', *, *, #17622, .T. ) ;
#48706=ORIENTED_EDGE ( 'NONE', *, *, #20569, .F. ) ;
#48711=DIRECTION ( 'NONE',  ( -1.000000000000000000, 0.000000000000000000, 0.000000000000000000 ) ) ;
#48712=ORIENTED_EDGE ( 'NONE', *, *, #45472, .T. ) ;
#48713=CARTESIAN_POINT ( 'NONE',  ( -332.3517673607765914, -70.03480886230919111, 25.08789112700620194 ) ) ;
#48716=ORIENTED_EDGE ( 'NONE', *, *, #11333, .F. ) ;
#48723=VERTEX_POINT ( 'NONE', #48606 ) ;
#48725=DIRECTION ( 'NONE',  ( 0.000000000000000000, -0.9350162426854181641, -0.3546048870425267951 ) ) ;
#48729=CARTESIAN_POINT ( 'NONE',  ( -330.4913330509368166, -115.8919814278863356, 58.50955523165747252 ) ) ;
#48731=CARTESIAN_POINT ( 'NONE',  ( -336.3521761649654422, -139.2044816956407089, -56.89493493766761389 ) ) ;
#48733=EDGE_LOOP ( 'NONE', ( #34305, #39932, #27650, #14873 ) ) ;
#48734=ADVANCED_FACE ( 'NONE', ( #13102 ), #40955, .F. ) ;
#48736=ADVANCED_FACE ( 'NONE', ( #45436 ), #20732, .F. ) ;
#48739=EDGE_CURVE ( 'NONE', #8885, #34018, #49382, .T. ) ;
#48741=EDGE_CURVE ( 'NONE', #41226, #18084, #41468, .T. ) ;
#48742=ORIENTED_EDGE ( 'NONE', *, *, #12429, .F. ) ;
#48746=AXIS2_PLACEMENT_3D ( 'NONE', #4099, #16964, #32970 ) ;
#48751=EDGE_CURVE ( 'NONE', #38969, #42568, #17323, .T. ) ;
#48753=FACE_OUTER_BOUND ( 'NONE', #34828, .T. ) ;
#48756=DIRECTION ( 'NONE',  ( -1.000000000000000000, -5.928974370888873265E-15, 8.589602288500856790E-15 ) ) ;
#48761=DIRECTION ( 'NONE',  ( 0.000000000000000000, 0.000000000000000000, 1.000000000000000000 ) ) ;
#48768=ORIENTED_EDGE ( 'NONE', *, *, #11459, .F. ) ;
#48771=DIRECTION ( 'NONE',  ( -0.000000000000000000, 0.5680647467311540355, -0.8229838658936575735 ) ) ;
#48774=FACE_BOUND ( 'NONE', #10940, .T. ) ;
#48778=EDGE_LOOP ( 'NONE', ( #17601, #9107, #5480, #32517 ) ) ;
#48781=VERTEX_POINT ( 'NONE', #16808 ) ;
#48787=VERTEX_POINT ( 'NONE', #4977 ) ;
#48791=EDGE_LOOP ( 'NONE', ( #15621, #17973, #5538, #7094 ) ) ;
#48792=DIRECTION ( 'NONE',  ( -0.000000000000000000, 0.2393156642875547968, -0.9709418174260527890 ) ) ;
#48798=ADVANCED_FACE ( 'NONE', ( #20462 ), #25200, .F. ) ;
#48804=ORIENTED_EDGE ( 'NONE', *, *, #43198, .T. ) ;
#48807=EDGE_CURVE ( 'NONE', #1947, #36354, #38043, .T. ) ;
#48811=VERTEX_POINT ( 'NONE', #29904 ) ;
#48817=DIRECTION ( 'NONE',  ( -0.000000000000000000, -0.4647231720437604574, 0.8854560256532141294 ) ) ;
#48822=DIRECTION ( 'NONE',  ( -1.000000000000000000, 0.000000000000000000, 0.000000000000000000 ) ) ;
#48824=EDGE_CURVE ( 'NONE', #27774, #39327, #42240, .T. ) ;
#48825=DIRECTION ( 'NONE',  ( -1.000000000000000000, -0.000000000000000000, 0.000000000000000000 ) ) ;
#48828=EDGE_CURVE ( 'NONE', #6831, #21096, #17830, .T. ) ;
#48829=DIRECTION ( 'NONE',  ( 1.000000000000000000, -0.000000000000000000, -0.000000000000000000 ) ) ;
#48837=CARTESIAN_POINT ( 'NONE',  ( -339.1964088526558498, -102.1108035431478811, -54.98865587491830809 ) ) ;
#48842=DIRECTION ( 'NONE',  ( 0.000000000000000000, -0.8229838658936494689, 0.5680647467311658039 ) ) ;
#48844=ORIENTED_EDGE ( 'NONE', *, *, #11455, .T. ) ;
#48850=ORIENTED_EDGE ( 'NONE', *, *, #11459, .T. ) ;
#48851=PLANE ( 'NONE',  #12143 ) ;
#48855=ORIENTED_EDGE ( 'NONE', *, *, #8938, .T. ) ;
#48857=CARTESIAN_POINT ( 'NONE',  ( -330.4913330509368166, -123.5000000000000284, 0.000000000000000000 ) ) ;
#48862=CIRCLE ( 'NONE', #48021, 10.00000000000000711 ) ;
#48864=VECTOR ( 'NONE', #6507, 1000.000000000000000 ) ;
#48866=FACE_OUTER_BOUND ( 'NONE', #31406, .T. ) ;
#48874=DIRECTION ( 'NONE',  ( 1.000000000000000000, -0.000000000000000000, -0.000000000000000000 ) ) ;
#48882=VERTEX_POINT ( 'NONE', #10715 ) ;
#48883=ORIENTED_EDGE ( 'NONE', *, *, #9475, .T. ) ;
#48884=AXIS2_PLACEMENT_3D ( 'NONE', #47847, #35225, #15524 ) ;
#48890=ORIENTED_EDGE ( 'NONE', *, *, #17690, .F. ) ;
#48893=AXIS2_PLACEMENT_3D ( 'NONE', #32055, #47849, #3679 ) ;
#48894=CIRCLE ( 'NONE', #28712, 60.00000000000000000 ) ;
#48896=DIRECTION ( 'NONE',  ( 0.000000000000000000, 0.6631226582407989678, 0.7485107481710977506 ) ) ;
#48908=EDGE_LOOP ( 'NONE', ( #5631, #39556, #23476, #44793 ) ) ;
#48910=VECTOR ( 'NONE', #52034, 1000.000000000000000 ) ;
#48913=CARTESIAN_POINT ( 'NONE',  ( -332.3517673607765914, -177.7325358280884586, 23.38292116578760726 ) ) ;
#48917=VECTOR ( 'NONE', #24969, 1000.000000000000000 ) ;
#48920=DIRECTION ( 'NONE',  ( 1.000000000000000000, 0.000000000000000000, 0.000000000000000000 ) ) ;
#48922=DIRECTION ( 'NONE',  ( 0.000000000000000000, 0.000000000000000000, -1.000000000000000000 ) ) ;
#48923=FACE_OUTER_BOUND ( 'NONE', #28046, .T. ) ;
#48925=ADVANCED_FACE ( 'NONE', ( #34371 ), #50930, .T. ) ;
#48926=VECTOR ( 'NONE', #11760, 1000.000000000000000 ) ;
#48928=DIRECTION ( 'NONE',  ( 0.000000000000000000, -0.8229838658936516893, 0.5680647467311625842 ) ) ;
#48930=VECTOR ( 'NONE', #25216, 1000.000000000000227 ) ;
#48932=DIRECTION ( 'NONE',  ( -1.000000000000000000, -0.000000000000000000, -0.000000000000000000 ) ) ;
#48936=DIRECTION ( 'NONE',  ( -0.000000000000000000, 0.9927088740980553050, 0.1205366802553130001 ) ) ;
#48942=LINE ( 'NONE', #44212, #22839 ) ;
#48946=CARTESIAN_POINT ( 'NONE',  ( -305.0000000000000568, -101.7569374291128383, -55.92172413327835301 ) ) ;
#48949=ORIENTED_EDGE ( 'NONE', *, *, #14304, .T. ) ;
#48950=VERTEX_POINT ( 'NONE', #22802 ) ;
#48952=DIRECTION ( 'NONE',  ( 0.000000000000000000, 0.000000000000000000, -1.000000000000000000 ) ) ;
#48954=CARTESIAN_POINT ( 'NONE',  ( -330.4913330509368166, -123.5000000000000284, 0.000000000000000000 ) ) ;
#48956=ORIENTED_EDGE ( 'NONE', *, *, #5565, .F. ) ;
#48957=VECTOR ( 'NONE', #10410, 1000.000000000000114 ) ;
#48958=EDGE_LOOP ( 'NONE', ( #50567, #33843, #30657, #32920 ) ) ;
#48964=ORIENTED_EDGE ( 'NONE', *, *, #12058, .T. ) ;
#48965=DIRECTION ( 'NONE',  ( 1.043714542225393539E-14, 0.4647231720437755564, 0.8854560256532062468 ) ) ;
#48967=EDGE_CURVE ( 'NONE', #30801, #3547, #25708, .T. ) ;
#48968=AXIS2_PLACEMENT_3D ( 'NONE', #49592, #5190, #41427 ) ;
#48969=LINE ( 'NONE', #36878, #39992 ) ;
#48973=ORIENTED_EDGE ( 'NONE', *, *, #31065, .F. ) ;
#48976=CARTESIAN_POINT ( 'NONE',  ( -330.4913330509368166, -168.7406467949202806, 39.41172259083927543 ) ) ;
#48978=PLANE ( 'NONE',  #50082 ) ;
#48980=DIRECTION ( 'NONE',  ( -1.000000000000000000, 0.000000000000000000, 0.000000000000000000 ) ) ;
#48985=LINE ( 'NONE', #21116, #12268 ) ;
#48986=VECTOR ( 'NONE', #29389, 1000.000000000000000 ) ;
#48988=DIRECTION ( 'NONE',  ( 0.000000000000000000, 0.000000000000000000, -1.000000000000000000 ) ) ;
#48989=ORIENTED_EDGE ( 'NONE', *, *, #46097, .T. ) ;
#48993=ORIENTED_EDGE ( 'NONE', *, *, #50243, .F. ) ;
#48996=FACE_OUTER_BOUND ( 'NONE', #40779, .T. ) ;
#48998=DIRECTION ( 'NONE',  ( -1.000000000000000000, 0.000000000000000000, 0.000000000000000000 ) ) ;
#49000=LINE ( 'NONE', #17476, #7707 ) ;
#49002=ORIENTED_EDGE ( 'NONE', *, *, #37863, .F. ) ;
#49006=CARTESIAN_POINT ( 'NONE',  ( -332.3517673607765914, -98.41210887299327226, -53.46519113769058151 ) ) ;
#49008=ORIENTED_EDGE ( 'NONE', *, *, #48430, .F. ) ;
#49009=PLANE ( 'NONE',  #33261 ) ;
#49013=CARTESIAN_POINT ( 'NONE',  ( -340.0000000000000568, -168.5000000000000284, 0.000000000000000000 ) ) ;
#49014=VERTEX_POINT ( 'NONE', #47249 ) ;
#49020=ORIENTED_EDGE ( 'NONE', *, *, #822, .T. ) ;
#49023=VERTEX_POINT ( 'NONE', #43286 ) ;
#49027=FACE_BOUND ( 'NONE', #27360, .T. ) ;
#49040=CARTESIAN_POINT ( 'NONE',  ( -336.3521761649653854, -129.1091364105427033, 59.73723787327234191 ) ) ;
#49041=CARTESIAN_POINT ( 'NONE',  ( -330.4913330509368166, -123.5000000000000284, 0.000000000000000000 ) ) ;
#49044=CARTESIAN_POINT ( 'NONE',  ( -332.3517673607765914, -63.67752800890095699, 4.612141029301498385 ) ) ;
#49046=EDGE_CURVE ( 'NONE', #38839, #5823, #16368, .T. ) ;
#49048=FACE_OUTER_BOUND ( 'NONE', #16603, .T. ) ;
#49052=EDGE_CURVE ( 'NONE', #37318, #15638, #15445, .T. ) ;
#49053=VECTOR ( 'NONE', #45965, 1000.000000000000000 ) ;
#49054=LINE ( 'NONE', #1205, #23951 ) ;
#49062=EDGE_LOOP ( 'NONE', ( #30357, #26436, #20650, #4428 ) ) ;
#49063=DIRECTION ( 'NONE',  ( 1.000000000000000000, -0.000000000000000000, -0.000000000000000000 ) ) ;
#49064=EDGE_LOOP ( 'NONE', ( #43934, #6600, #1562, #34764 ) ) ;
#49065=FACE_OUTER_BOUND ( 'NONE', #12036, .T. ) ;
#49069=ORIENTED_EDGE ( 'NONE', *, *, #37166, .F. ) ;
#49071=DIRECTION ( 'NONE',  ( 0.000000000000000000, -3.393119119010634677E-13, 1.000000000000000000 ) ) ;
#49072=DIRECTION ( 'NONE',  ( -0.000000000000000000, 0.9709418174260519008, -0.2393156642875582940 ) ) ;
#49074=PLANE ( 'NONE',  #26889 ) ;
#49077=VERTEX_POINT ( 'NONE', #16682 ) ;
#49078=EDGE_CURVE ( 'NONE', #40382, #12661, #47499, .T. ) ;
#49079=DIRECTION ( 'NONE',  ( -1.000000000000000000, 0.000000000000000000, -0.000000000000000000 ) ) ;
#49081=VECTOR ( 'NONE', #38303, 1000.000000000000000 ) ;
#49089=ADVANCED_FACE ( 'NONE', ( #19629 ), #35653, .T. ) ;
#49090=EDGE_CURVE ( 'NONE', #22824, #23304, #20595, .T. ) ;
#49092=VECTOR ( 'NONE', #50035, 1000.000000000000000 ) ;
#49094=DIRECTION ( 'NONE',  ( 0.000000000000000000, -0.8854560256532141294, -0.4647231720437604574 ) ) ;
#49096=VERTEX_POINT ( 'NONE', #13496 ) ;
#49097=DIRECTION ( 'NONE',  ( 0.000000000000000000, 0.8854560256532062468, -0.4647231720437755564 ) ) ;
#49098=DIRECTION ( 'NONE',  ( 0.000000000000000000, -5.851800525628429686E-14, -1.000000000000000000 ) ) ;
#49100=EDGE_LOOP ( 'NONE', ( #5153, #42531, #21014, #32540 ) ) ;
#49101=EDGE_CURVE ( 'NONE', #25971, #33577, #50024, .T. ) ;
#49102=VECTOR ( 'NONE', #13413, 1000.000000000000000 ) ;
#49104=ORIENTED_EDGE ( 'NONE', *, *, #15989, .T. ) ;
#49105=DIRECTION ( 'NONE',  ( -0.000000000000000000, -0.9927088740980548609, -0.1205366802553164696 ) ) ;
#49117=LINE ( 'NONE', #24667, #14478 ) ;
#49119=EDGE_CURVE ( 'NONE', #44157, #36786, #48985, .T. ) ;
#49121=EDGE_LOOP ( 'NONE', ( #2722, #47975, #17569, #37231 ) ) ;
#49123=ADVANCED_FACE ( 'NONE', ( #21650 ), #41871, .F. ) ;
#49125=FACE_OUTER_BOUND ( 'NONE', #9073, .T. ) ;
#49129=EDGE_CURVE ( 'NONE', #31195, #15564, #17185, .T. ) ;
#49131=ORIENTED_EDGE ( 'NONE', *, *, #34958, .F. ) ;
#49132=AXIS2_PLACEMENT_3D ( 'NONE', #45680, #25698, #4691 ) ;
#49135=DIRECTION ( 'NONE',  ( -0.000000000000000000, -0.8854560256532126861, -0.4647231720437631775 ) ) ;
#49136=ORIENTED_EDGE ( 'NONE', *, *, #16276, .T. ) ;
#49137=ORIENTED_EDGE ( 'NONE', *, *, #32596, .T. ) ;
#49142=FACE_OUTER_BOUND ( 'NONE', #37595, .T. ) ;
#49146=CIRCLE ( 'NONE', #9710, 10.00000000000000711 ) ;
#49147=VERTEX_POINT ( 'NONE', #9815 ) ;
#49148=VECTOR ( 'NONE', #39628, 999.9999999999998863 ) ;
#49155=DIRECTION ( 'NONE',  ( 0.000000000000000000, 0.000000000000000000, 1.000000000000000000 ) ) ;
#49156=ADVANCED_FACE ( 'NONE', ( #33479 ), #49248, .F. ) ;
#49157=EDGE_CURVE ( 'NONE', #16904, #37128, #880, .T. ) ;
#49161=DIRECTION ( 'NONE',  ( 0.000000000000000000, -0.3546048870425396182, -0.9350162426854132791 ) ) ;
#49163=DIRECTION ( 'NONE',  ( 1.000000000000000000, 0.000000000000000000, 0.000000000000000000 ) ) ;
#49165=DIRECTION ( 'NONE',  ( 0.000000000000000000, 0.8854560256532079121, -0.4647231720437725033 ) ) ;
#49170=ORIENTED_EDGE ( 'NONE', *, *, #29022, .T. ) ;
#49171=VECTOR ( 'NONE', #42591, 1000.000000000000114 ) ;
#49179=EDGE_CURVE ( 'NONE', #42349, #42455, #13244, .T. ) ;
#49184=LINE ( 'NONE', #29449, #16747 ) ;
#49187=EDGE_LOOP ( 'NONE', ( #28982, #841, #40579, #33163 ) ) ;
#49189=CARTESIAN_POINT ( 'NONE',  ( -305.0000000000000568, -183.4979166304964622, 0.4999999999996888600 ) ) ;
#49191=EDGE_CURVE ( 'NONE', #21096, #6808, #25325, .T. ) ;
#49193=LINE ( 'NONE', #48408, #11498 ) ;
#49204=LINE ( 'NONE', #45276, #4385 ) ;
#49206=VECTOR ( 'NONE', #820, 1000.000000000000114 ) ;
#49208=ORIENTED_EDGE ( 'NONE', *, *, #36252, .T. ) ;
#49209=DIRECTION ( 'NONE',  ( 0.000000000000000000, 0.4647231720437664526, -0.8854560256532110207 ) ) ;
#49211=CARTESIAN_POINT ( 'NONE',  ( -336.3521761649654422, -165.2193480479701293, -43.12187378178660424 ) ) ;
#49212=ORIENTED_EDGE ( 'NONE', *, *, #26615, .F. ) ;
#49213=ORIENTED_EDGE ( 'NONE', *, *, #2411, .F. ) ;
#49214=VECTOR ( 'NONE', #7665, 1000.000000000000000 ) ;
#49215=ORIENTED_EDGE ( 'NONE', *, *, #617, .T. ) ;
#49218=CIRCLE ( 'NONE', #13120, 60.00000000000000000 ) ;
#49221=VECTOR ( 'NONE', #29871, 1000.000000000000114 ) ;
#49228=CARTESIAN_POINT ( 'NONE',  ( -332.3517673607765914, -133.3383340306578759, -59.18789727217212970 ) ) ;
#49230=LINE ( 'NONE', #13480, #15477 ) ;
#49231=VERTEX_POINT ( 'NONE', #5360 ) ;
#49238=CARTESIAN_POINT ( 'NONE',  ( -339.1964088526558498, -179.7763290203206452, 20.80804632820241906 ) ) ;
#49241=VERTEX_POINT ( 'NONE', #21378 ) ;
#49242=EDGE_CURVE ( 'NONE', #14193, #9248, #12186, .T. ) ;
#49244=VECTOR ( 'NONE', #13434, 1000.000000000000114 ) ;
#49247=FACE_BOUND ( 'NONE', #21694, .T. ) ;
#49248=PLANE ( 'NONE',  #38189 ) ;
#49249=EDGE_LOOP ( 'NONE', ( #21866, #41838, #35166, #44055 ) ) ;
#49250=DIRECTION ( 'NONE',  ( 0.000000000000000000, -0.8854560256532044704, 0.4647231720437789981 ) ) ;
#49256=VERTEX_POINT ( 'NONE', #19260 ) ;
#49260=CARTESIAN_POINT ( 'NONE',  ( -330.4913330509368166, -63.99980407363855761, 7.728304129923846411 ) ) ;
#49262=ADVANCED_FACE ( 'NONE', ( #6658 ), #50289, .F. ) ;
#49263=DIRECTION ( 'NONE',  ( -0.000000000000000000, -0.8229838658936596829, -0.5680647467311510379 ) ) ;
#49266=AXIS2_PLACEMENT_3D ( 'NONE', #46270, #46782, #2375 ) ;
#49267=ORIENTED_EDGE ( 'NONE', *, *, #24257, .T. ) ;
#49268=ORIENTED_EDGE ( 'NONE', *, *, #35036, .T. ) ;
#49270=CARTESIAN_POINT ( 'NONE',  ( -339.1964088526558498, -130.1153096980144426, 58.63009191191295599 ) ) ;
#49271=EDGE_LOOP ( 'NONE', ( #960, #2000, #49736, #35085 ) ) ;
#49272=EDGE_LOOP ( 'NONE', ( #8730, #12849, #6890, #27768 ) ) ;
#49273=CARTESIAN_POINT ( 'NONE',  ( -336.3521761649654422, -123.5000000000000284, 0.000000000000000000 ) ) ;
#49275=FACE_OUTER_BOUND ( 'NONE', #50022, .T. ) ;
#49276=FACE_OUTER_BOUND ( 'NONE', #38894, .T. ) ;
#49278=ORIENTED_EDGE ( 'NONE', *, *, #47450, .T. ) ;
#49286=CARTESIAN_POINT ( 'NONE',  ( -332.3517673607765914, -64.50000000000000000, -1.632288850093980725 ) ) ;
#49291=DIRECTION ( 'NONE',  ( 0.000000000000000000, 0.9709418174260544543, 0.2393156642875482742 ) ) ;
#49294=VECTOR ( 'NONE', #27623, 1000.000000000000000 ) ;
#49296=CARTESIAN_POINT ( 'NONE',  ( -336.3521761649654422, -180.1556192733800117, 16.67542351306693149 ) ) ;
#49298=ORIENTED_EDGE ( 'NONE', *, *, #44942, .F. ) ;
#49303=ORIENTED_EDGE ( 'NONE', *, *, #8678, .F. ) ;
#49306=ADVANCED_FACE ( 'NONE', ( #18475 ), #10329, .T. ) ;
#49313=VERTEX_POINT ( 'NONE', #51075 ) ;
#49315=DIRECTION ( 'NONE',  ( 0.000000000000000000, 0.000000000000000000, -1.000000000000000000 ) ) ;
#49316=VECTOR ( 'NONE', #7788, 1000.000000000000227 ) ;
#49317=VECTOR ( 'NONE', #222, 1000.000000000000114 ) ;
#49323=CARTESIAN_POINT ( 'NONE',  ( -330.4913330509368166, -182.1300919119129560, -6.615309698014691264 ) ) ;
#49326=FACE_OUTER_BOUND ( 'NONE', #39743, .T. ) ;
#49346=ADVANCED_FACE ( 'NONE', ( #26862 ), #46343, .F. ) ;
#49352=FACE_OUTER_BOUND ( 'NONE', #46181, .T. ) ;
#49354=CARTESIAN_POINT ( 'NONE',  ( -336.3521761649653854, -103.7577981350106313, -56.65902810251876787 ) ) ;
#49356=EDGE_CURVE ( 'NONE', #19121, #12363, #27378, .T. ) ;
#49357=ORIENTED_EDGE ( 'NONE', *, *, #49356, .F. ) ;
#49358=DIRECTION ( 'NONE',  ( 1.000000000000000000, -0.000000000000000000, -0.000000000000000000 ) ) ;
#49359=DIRECTION ( 'NONE',  ( -0.000000000000000000, 0.3546048870425235200, -0.9350162426854194964 ) ) ;
#49360=EDGE_LOOP ( 'NONE', ( #37689, #17490, #8219, #40848 ) ) ;
#49362=EDGE_CURVE ( 'NONE', #37884, #19283, #10583, .T. ) ;
#49366=CARTESIAN_POINT ( 'NONE',  ( -332.3517673607765914, -101.0520950768976149, 54.58714071513087873 ) ) ;
#49368=VERTEX_POINT ( 'NONE', #43429 ) ;
#49369=VECTOR ( 'NONE', #11375, 1000.000000000000000 ) ;
#49374=CARTESIAN_POINT ( 'NONE',  ( -330.4913330509368166, -138.1050951016791544, -57.16590939599326049 ) ) ;
#49376=ORIENTED_EDGE ( 'NONE', *, *, #38521, .T. ) ;
#49379=VECTOR ( 'NONE', #13168, 999.9999999999998863 ) ;
#49380=ORIENTED_EDGE ( 'NONE', *, *, #44001, .F. ) ;
#49382=LINE ( 'NONE', #16544, #50032 ) ;
#49383=DIRECTION ( 'NONE',  ( 0.000000000000000000, 0.000000000000000000, 1.000000000000000000 ) ) ;
#49385=ORIENTED_EDGE ( 'NONE', *, *, #19716, .T. ) ;
#49391=DIRECTION ( 'NONE',  ( -0.000000000000000000, 0.9350162426854194964, 0.3546048870425235200 ) ) ;
#49396=ORIENTED_EDGE ( 'NONE', *, *, #259, .T. ) ;
#49397=AXIS2_PLACEMENT_3D ( 'NONE', #45817, #37922, #13495 ) ;
#49401=CARTESIAN_POINT ( 'NONE',  ( -332.3517673607765914, -123.5000000000000284, 0.000000000000000000 ) ) ;
#49405=ADVANCED_FACE ( 'NONE', ( #23199 ), #31323, .F. ) ;
#49406=CARTESIAN_POINT ( 'NONE',  ( -332.3517673607765914, -106.5990858529439578, 57.57047073799066794 ) ) ;
#49408=ADVANCED_FACE ( 'NONE', ( #47 ), #32098, .F. ) ;
#49409=ADVANCED_FACE ( 'NONE', ( #51840 ), #8196, .F. ) ;
#49412=EDGE_CURVE ( 'NONE', #16981, #29431, #44195, .T. ) ;
#49416=ADVANCED_FACE ( 'NONE', ( #7674 ), #35518, .F. ) ;
#49418=DIRECTION ( 'NONE',  ( 0.000000000000000000, 0.6631226582407937498, -0.7485107481711024136 ) ) ;
#49420=CARTESIAN_POINT ( 'NONE',  ( -332.3517673607765914, -176.9651911376907094, -25.08789112700655721 ) ) ;
#49421=ORIENTED_EDGE ( 'NONE', *, *, #6108, .T. ) ;
#49422=ADVANCED_FACE ( 'NONE', ( #27648 ), #47635, .F. ) ;
#49429=DIRECTION ( 'NONE',  ( 0.000000000000000000, 0.9709418174260511236, -0.2393156642875615969 ) ) ;
#49430=EDGE_CURVE ( 'NONE', #43701, #3626, #48144, .T. ) ;
#49432=DIRECTION ( 'NONE',  ( 1.000000000000000000, -0.000000000000000000, -0.000000000000000000 ) ) ;
#49433=DIRECTION ( 'NONE',  ( 1.000000000000000000, 0.000000000000000000, 0.000000000000000000 ) ) ;
#49438=VERTEX_POINT ( 'NONE', #4252 ) ;
#49439=VECTOR ( 'NONE', #19494, 1000.000000000000114 ) ;
#49440=VECTOR ( 'NONE', #26256, 1000.000000000000000 ) ;
#49450=ADVANCED_FACE ( 'NONE', ( #36300 ), #39971, .F. ) ;
#49451=ORIENTED_EDGE ( 'NONE', *, *, #31055, .F. ) ;
#49459=CARTESIAN_POINT ( 'NONE',  ( -336.3521761649654422, -182.3871109312487420, -4.498567634386014369 ) ) ;
#49460=CARTESIAN_POINT ( 'NONE',  ( -339.1964088526558498, -74.65991953890876687, -33.10432812419148263 ) ) ;
#49465=EDGE_CURVE ( 'NONE', #8505, #21100, #27893, .T. ) ;
#49466=DIRECTION ( 'NONE',  ( -1.000000000000000000, 0.000000000000000000, 0.000000000000000000 ) ) ;
#49469=PLANE ( 'NONE',  #49621 ) ;
#49472=CARTESIAN_POINT ( 'NONE',  ( -339.1964088526558498, -171.7720157143598669, 33.92731199008546383 ) ) ;
#49473=EDGE_CURVE ( 'NONE', #20303, #35874, #36048, .T. ) ;
#49479=LINE ( 'NONE', #29468, #4408 ) ;
#49480=DIRECTION ( 'NONE',  ( -8.718379230999708359E-17, -0.9709418174260544543, -0.2393156642875482742 ) ) ;
#49483=ORIENTED_EDGE ( 'NONE', *, *, #15046, .F. ) ;
#49487=DIRECTION ( 'NONE',  ( 0.000000000000000000, 0.000000000000000000, -1.000000000000000000 ) ) ;
#49488=ORIENTED_EDGE ( 'NONE', *, *, #13450, .T. ) ;
#49489=ORIENTED_EDGE ( 'NONE', *, *, #48160, .T. ) ;
#49498=VECTOR ( 'NONE', #34686, 1000.000000000000000 ) ;
#49501=EDGE_LOOP ( 'NONE', ( #27381, #51433, #1560, #25184 ) ) ;
#49502=DIRECTION ( 'NONE',  ( 0.000000000000000000, 0.8229838658936575735, 0.5680647467311540355 ) ) ;
#49510=EDGE_LOOP ( 'NONE', ( #49517, #7636, #19840, #39237 ) ) ;
#49511=ORIENTED_EDGE ( 'NONE', *, *, #37704, .F. ) ;
#49517=ORIENTED_EDGE ( 'NONE', *, *, #23976, .T. ) ;
#49518=CARTESIAN_POINT ( 'NONE',  ( -339.1964088526558498, -167.3305728129742249, 39.49849221029288060 ) ) ;
#49519=DIRECTION ( 'NONE',  ( -1.000000000000000000, 0.000000000000000000, -0.000000000000000000 ) ) ;
#49534=CIRCLE ( 'NONE', #35237, 60.00000000000000000 ) ;
#49539=LINE ( 'NONE', #37422, #6901 ) ;
#49540=ORIENTED_EDGE ( 'NONE', *, *, #10535, .F. ) ;
#49541=EDGE_LOOP ( 'NONE', ( #42151, #32680, #17921, #7518 ) ) ;
#49544=ORIENTED_EDGE ( 'NONE', *, *, #35915, .T. ) ;
#49547=EDGE_CURVE ( 'NONE', #17630, #45109, #33916, .T. ) ;
#49548=VERTEX_POINT ( 'NONE', #49964 ) ;
#49554=ORIENTED_EDGE ( 'NONE', *, *, #33967, .F. ) ;
#49560=PLANE ( 'NONE',  #2879 ) ;
#49562=VECTOR ( 'NONE', #9275, 1000.000000000000114 ) ;
#49565=PLANE ( 'NONE',  #42411 ) ;
#49566=ORIENTED_EDGE ( 'NONE', *, *, #5233, .T. ) ;
#49570=CARTESIAN_POINT ( 'NONE',  ( -339.1964088526558498, -84.00150778970699150, 43.83057281297409702 ) ) ;
#49571=DIRECTION ( 'NONE',  ( -1.000000000000000000, -1.013386094502324141E-14, -2.497772389992512055E-15 ) ) ;
#49574=EDGE_LOOP ( 'NONE', ( #16243, #4002, #2415, #27344 ) ) ;
#49576=LINE ( 'NONE', #5170, #39647 ) ;
#49579=ORIENTED_EDGE ( 'NONE', *, *, #33329, .F. ) ;
#49583=EDGE_CURVE ( 'NONE', #36418, #35955, #21061, .T. ) ;
#49588=DIRECTION ( 'NONE',  ( -0.000000000000000000, -0.3546048870425396182, -0.9350162426854132791 ) ) ;
#49589=ORIENTED_EDGE ( 'NONE', *, *, #38478, .T. ) ;
#49592=CARTESIAN_POINT ( 'NONE',  ( 0.000000000000000000, -74.94395191227387443, 33.51582005713760282 ) ) ;
#49593=VERTEX_POINT ( 'NONE', #13959 ) ;
#49594=CIRCLE ( 'NONE', #26915, 60.00000000000000000 ) ;
#49597=PLANE ( 'NONE',  #19530 ) ;
#49598=EDGE_LOOP ( 'NONE', ( #34802, #1318, #3958, #590 ) ) ;
#49605=CARTESIAN_POINT ( 'NONE',  ( -336.3521761649653854, -79.68838513426354098, -40.99441916720346057 ) ) ;
#49606=AXIS2_PLACEMENT_3D ( 'NONE', #3260, #15343, #26897 ) ;
#49607=EDGE_LOOP ( 'NONE', ( #48005, #37309, #45819, #8552 ) ) ;
#49609=LINE ( 'NONE', #46442, #30345 ) ;
#49612=LINE ( 'NONE', #1769, #2419 ) ;
#49614=ORIENTED_EDGE ( 'NONE', *, *, #20569, .T. ) ;
#49616=ORIENTED_EDGE ( 'NONE', *, *, #31283, .F. ) ;
#49618=EDGE_LOOP ( 'NONE', ( #2962, #33456, #39762, #1759 ) ) ;
#49619=CARTESIAN_POINT ( 'NONE',  ( -336.3521761649654422, -141.9604555052315220, 56.09938080879057765 ) ) ;
#49620=DIRECTION ( 'NONE',  ( 0.000000000000000000, 0.6631226582407863113, -0.7485107481711089639 ) ) ;
#49621=AXIS2_PLACEMENT_3D ( 'NONE', #2399, #26293, #13447 ) ;
#49622=VERTEX_POINT ( 'NONE', #17403 ) ;
#49627=CARTESIAN_POINT ( 'NONE',  ( -365.0000000000001137, -168.5000000000000284, 0.000000000000000000 ) ) ;
#49629=AXIS2_PLACEMENT_3D ( 'NONE', #4151, #719, #29074 ) ;
#49635=DIRECTION ( 'NONE',  ( -0.000000000000000000, 0.3546048870425463906, 0.9350162426854107256 ) ) ;
#49638=DIRECTION ( 'NONE',  ( 0.000000000000000000, 0.000000000000000000, 1.000000000000000000 ) ) ;
#49641=CARTESIAN_POINT ( 'NONE',  ( -332.3517673607765914, -149.0257676989619142, 54.29949524055110999 ) ) ;
#49644=PLANE ( 'NONE',  #33057 ) ;
#49646=EDGE_CURVE ( 'NONE', #22837, #22268, #15583, .T. ) ;
#49655=CARTESIAN_POINT ( 'NONE',  ( -336.3521761649654422, -181.4155151828941825, -11.56382487286496463 ) ) ;
#49656=EDGE_LOOP ( 'NONE', ( #9330, #18848, #35044, #19446 ) ) ;
#49660=CARTESIAN_POINT ( 'NONE',  ( -336.3521761649654422, -118.0087234915157381, -58.76657425099333665 ) ) ;
#49661=CARTESIAN_POINT ( 'NONE',  ( 0.000000000000000000, -71.25809448646026567, 27.41866715058169390 ) ) ;
#49663=PLANE ( 'NONE',  #31886 ) ;
#49667=ORIENTED_EDGE ( 'NONE', *, *, #15006, .T. ) ;
#49668=FACE_OUTER_BOUND ( 'NONE', #49272, .T. ) ;
#49669=ORIENTED_EDGE ( 'NONE', *, *, #10754, .F. ) ;
#49674=FACE_OUTER_BOUND ( 'NONE', #46268, .T. ) ;
#49675=EDGE_LOOP ( 'NONE', ( #23277, #45547, #28873, #12473 ) ) ;
#49676=DIRECTION ( 'NONE',  ( 0.000000000000000000, 0.1205366802553338029, 0.9927088740980527515 ) ) ;
#49677=CARTESIAN_POINT ( 'NONE',  ( -332.3517673607765914, -93.75055682584159911, 51.01861988938794923 ) ) ;
#49695=CARTESIAN_POINT ( 'NONE',  ( -336.3521761649654422, -176.5004679656469477, -25.97334715265976612 ) ) ;
#49696=DIRECTION ( 'NONE',  ( -0.000000000000000000, -0.5680647467311510379, 0.8229838658936596829 ) ) ;
#49698=FACE_OUTER_BOUND ( 'NONE', #30230, .T. ) ;
#49700=PLANE ( 'NONE',  #522 ) ;
#49705=DIRECTION ( 'NONE',  ( -1.000000000000000000, 0.000000000000000000, -0.000000000000000000 ) ) ;
#49713=EDGE_CURVE ( 'NONE', #21438, #36520, #38112, .T. ) ;
#49714=CARTESIAN_POINT ( 'NONE',  ( -330.4913330509368166, -115.8919814278863356, 58.50955523165747252 ) ) ;
#49718=VECTOR ( 'NONE', #26058, 1000.000000000000000 ) ;
#49724=ORIENTED_EDGE ( 'NONE', *, *, #45542, .F. ) ;
#49728=ORIENTED_EDGE ( 'NONE', *, *, #48573, .F. ) ;
#49729=EDGE_CURVE ( 'NONE', #21286, #38437, #10027, .T. ) ;
#49736=ORIENTED_EDGE ( 'NONE', *, *, #33616, .F. ) ;
#49741=VERTEX_POINT ( 'NONE', #26040 ) ;
#49744=CARTESIAN_POINT ( 'NONE',  ( -339.1964088526558498, -75.22798428563942252, 33.92731199008440512 ) ) ;
#49746=ADVANCED_FACE ( 'NONE', ( #18677 ), #22358, .F. ) ;
#49747=EDGE_CURVE ( 'NONE', #37538, #33858, #34186, .T. ) ;
#49748=ADVANCED_FACE ( 'NONE', ( #46536 ), #6845, .F. ) ;
#49750=DIRECTION ( 'NONE',  ( -1.000000000000000000, 0.000000000000000000, 0.000000000000000000 ) ) ;
#49756=ORIENTED_EDGE ( 'NONE', *, *, #25671, .T. ) ;
#49758=EDGE_LOOP ( 'NONE', ( #6143, #25904, #47078, #4573 ) ) ;
#49761=ORIENTED_EDGE ( 'NONE', *, *, #14190, .F. ) ;
#49767=DIRECTION ( 'NONE',  ( 0.000000000000000000, -0.4647231720437573488, 0.8854560256532157947 ) ) ;
#49768=EDGE_CURVE ( 'NONE', #10964, #51141, #26287, .T. ) ;
#49771=ORIENTED_EDGE ( 'NONE', *, *, #51025, .F. ) ;
#49779=DIRECTION ( 'NONE',  ( 0.000000000000000000, 0.000000000000000000, -1.000000000000000000 ) ) ;
#49786=DIRECTION ( 'NONE',  ( 0.000000000000000000, -0.2393156642875448881, 0.9709418174260553425 ) ) ;
#49788=DIRECTION ( 'NONE',  ( 0.000000000000000000, 1.410908427127803051E-14, 1.000000000000000000 ) ) ;
#49794=EDGE_CURVE ( 'NONE', #47080, #42377, #4454, .T. ) ;
#49798=EDGE_LOOP ( 'NONE', ( #37334, #31899, #17592, #6996 ) ) ;
#49799=CARTESIAN_POINT ( 'NONE',  ( -339.1964088526558498, -115.8919814278871598, -58.50955523165758621 ) ) ;
#49801=DIRECTION ( 'NONE',  ( 0.000000000000000000, 0.000000000000000000, 1.000000000000000000 ) ) ;
#49802=CARTESIAN_POINT ( 'NONE',  ( -336.3521761649653854, -136.2687678316390532, 58.62557946887775273 ) ) ;
#49809=DIRECTION ( 'NONE',  ( -1.000000000000000000, 0.000000000000000000, 0.000000000000000000 ) ) ;
#49810=CARTESIAN_POINT ( 'NONE',  ( -339.1964088526558498, -74.65991953890876687, -33.10432812419148263 ) ) ;
#49811=DIRECTION ( 'NONE',  ( 0.000000000000000000, 0.000000000000000000, 1.000000000000000000 ) ) ;
#49814=ORIENTED_EDGE ( 'NONE', *, *, #26326, .T. ) ;
#49821=DIRECTION ( 'NONE',  ( 0.000000000000000000, 0.000000000000000000, -1.000000000000000000 ) ) ;
#49824=LINE ( 'NONE', #18018, #39206 ) ;
#49825=CARTESIAN_POINT ( 'NONE',  ( -332.3517673607765914, -100.1170788342122080, 54.23253582808833073 ) ) ;
#49828=ORIENTED_EDGE ( 'NONE', *, *, #25974, .T. ) ;
#49832=ORIENTED_EDGE ( 'NONE', *, *, #39470, .F. ) ;
#49835=DIRECTION ( 'NONE',  ( 0.000000000000000000, 1.249000902703301108E-14, 1.000000000000000000 ) ) ;
#49836=VERTEX_POINT ( 'NONE', #4199 ) ;
#49837=DIRECTION ( 'NONE',  ( 0.000000000000000000, -6.129356281784718821E-14, -1.000000000000000000 ) ) ;
#49838=DIRECTION ( 'NONE',  ( 1.043714542225393223E-14, -0.1205366802553164696, 0.9927088740980548609 ) ) ;
#49840=CARTESIAN_POINT ( 'NONE',  ( -332.3517673607765914, -100.7053649598255021, 55.50139289590170222 ) ) ;
#49841=ADVANCED_FACE ( 'NONE', ( #15509 ), #43615, .F. ) ;
#49846=VERTEX_POINT ( 'NONE', #12327 ) ;
#49854=DIRECTION ( 'NONE',  ( 0.000000000000000000, 1.688464183284092344E-14, -1.000000000000000000 ) ) ;
#49856=LINE ( 'NONE', #13851, #13477 ) ;
#49857=VECTOR ( 'NONE', #42868, 999.9999999999998863 ) ;
#49863=CARTESIAN_POINT ( 'NONE',  ( -339.1964088526558498, -89.57268800991514013, -48.27201571436026484 ) ) ;
#49866=DIRECTION ( 'NONE',  ( 1.000000000000000000, 8.151826190875911381E-17, 3.091579882402618064E-17 ) ) ;
#49870=EDGE_LOOP ( 'NONE', ( #50153, #4757, #1289, #29826 ) ) ;
#49871=FACE_OUTER_BOUND ( 'NONE', #19164, .T. ) ;
#49872=VERTEX_POINT ( 'NONE', #23395 ) ;
#49875=DIRECTION ( 'NONE',  ( 1.000000000000000000, -0.000000000000000000, -0.000000000000000000 ) ) ;
#49876=DIRECTION ( 'NONE',  ( 1.000000000000000000, -0.000000000000000000, -0.000000000000000000 ) ) ;
#49878=ORIENTED_EDGE ( 'NONE', *, *, #27919, .T. ) ;
#49880=CARTESIAN_POINT ( 'NONE',  ( -332.3517673607765914, -177.7994952405510389, -25.52576769896207409 ) ) ;
#49883=LINE ( 'NONE', #9420, #25821 ) ;
#49884=VERTEX_POINT ( 'NONE', #8395 ) ;
#49885=AXIS2_PLACEMENT_3D ( 'NONE', #35028, #10858, #6411 ) ;
#49888=DIRECTION ( 'NONE',  ( 1.000000000000000000, -8.465038975556376573E-17, 2.086444717177636171E-17 ) ) ;
#49901=DIRECTION ( 'NONE',  ( -0.000000000000000000, 0.3546048870425331789, -0.9350162426854158326 ) ) ;
#49906=CARTESIAN_POINT ( 'NONE',  ( -332.3517673607765914, -127.9985676343858501, 58.88711093124869222 ) ) ;
#49907=VERTEX_POINT ( 'NONE', #27321 ) ;
#49908=LINE ( 'NONE', #37564, #23751 ) ;
#49910=EDGE_LOOP ( 'NONE', ( #1965, #51242, #30729, #11666 ) ) ;
#49911=LINE ( 'NONE', #38067, #35156 ) ;
#49912=EDGE_CURVE ( 'NONE', #4457, #32311, #45002, .T. ) ;
#49916=AXIS2_PLACEMENT_3D ( 'NONE', #32031, #16026, #7862 ) ;
#49917=DIRECTION ( 'NONE',  ( 1.000000000000000000, -0.000000000000000000, -0.000000000000000000 ) ) ;
#49921=DIRECTION ( 'NONE',  ( 0.000000000000000000, 0.000000000000000000, 1.000000000000000000 ) ) ;
#49929=EDGE_CURVE ( 'NONE', #25876, #17256, #5507, .T. ) ;
#49934=ORIENTED_EDGE ( 'NONE', *, *, #38686, .T. ) ;
#49937=ORIENTED_EDGE ( 'NONE', *, *, #32348, .T. ) ;
#49943=LINE ( 'NONE', #42564, #11622 ) ;
#49944=CARTESIAN_POINT ( 'NONE',  ( -332.3517673607765914, -98.41210887299327226, -53.46519113769058151 ) ) ;
#49945=CARTESIAN_POINT ( 'NONE',  ( -340.0000000000000568, -78.50000000000002842, 5.000000000000001776 ) ) ;
#49946=ORIENTED_EDGE ( 'NONE', *, *, #44992, .T. ) ;
#49950=DIRECTION ( 'NONE',  ( 0.000000000000000000, 0.2393156642875547968, -0.9709418174260527890 ) ) ;
#49957=DIRECTION ( 'NONE',  ( 0.000000000000000000, -0.9927088740980538617, 0.1205366802553232974 ) ) ;
#49961=ORIENTED_EDGE ( 'NONE', *, *, #24072, .T. ) ;
#49963=EDGE_CURVE ( 'NONE', #46969, #16966, #9186, .T. ) ;
#49964=CARTESIAN_POINT ( 'NONE',  ( -336.3521761649654422, -77.59233547837267508, 37.15394033962009246 ) ) ;
#49969=FACE_OUTER_BOUND ( 'NONE', #36900, .T. ) ;
#49980=CARTESIAN_POINT ( 'NONE',  ( -339.1964088526558498, -171.7720157143598669, 33.92731199008546383 ) ) ;
#49982=VERTEX_POINT ( 'NONE', #772 ) ;
#49983=EDGE_CURVE ( 'NONE', #45638, #48223, #4988, .T. ) ;
#49986=LINE ( 'NONE', #41837, #49718 ) ;
#49988=ORIENTED_EDGE ( 'NONE', *, *, #42378, .T. ) ;
#49990=ORIENTED_EDGE ( 'NONE', *, *, #19201, .T. ) ;
#49993=AXIS2_PLACEMENT_3D ( 'NONE', #20279, #48932, #3728 ) ;
#49995=CARTESIAN_POINT ( 'NONE',  ( -330.4913330509368166, -138.1050951016791544, -57.16590939599326049 ) ) ;
#50003=ADVANCED_FACE ( 'NONE', ( #48617 ), #21527, .F. ) ;
#50007=ORIENTED_EDGE ( 'NONE', *, *, #4594, .F. ) ;
#50012=VECTOR ( 'NONE', #31841, 1000.000000000000227 ) ;
#50018=DIRECTION ( 'NONE',  ( 0.000000000000000000, 0.000000000000000000, 1.000000000000000000 ) ) ;
#50019=CARTESIAN_POINT ( 'NONE',  ( -336.3521761649654422, -123.5000000000000284, 0.000000000000000000 ) ) ;
#50020=VERTEX_POINT ( 'NONE', #1279 ) ;
#50021=DIRECTION ( 'NONE',  ( 0.000000000000000000, 0.000000000000000000, -1.000000000000000000 ) ) ;
#50022=EDGE_LOOP ( 'NONE', ( #11009, #21632, #13891, #30530 ) ) ;
#50023=FACE_BOUND ( 'NONE', #44971, .T. ) ;
#50024=LINE ( 'NONE', #41597, #3748 ) ;
#50025=VERTEX_POINT ( 'NONE', #28870 ) ;
#50031=EDGE_LOOP ( 'NONE', ( #51942, #37785, #11585, #46873 ) ) ;
#50032=VECTOR ( 'NONE', #28601, 999.9999999999998863 ) ;
#50033=AXIS2_PLACEMENT_3D ( 'NONE', #42643, #47109, #27375 ) ;
#50035=DIRECTION ( 'NONE',  ( 1.000000000000000000, -0.000000000000000000, -0.000000000000000000 ) ) ;
#50047=ADVANCED_FACE ( 'NONE', ( #8908 ), #21004, .F. ) ;
#50051=VECTOR ( 'NONE', #2013, 1000.000000000000000 ) ;
#50054=PLANE ( 'NONE',  #18746 ) ;
#50057=EDGE_CURVE ( 'NONE', #27843, #32868, #17840, .T. ) ;
#50059=DIRECTION ( 'NONE',  ( -1.000000000000000000, 0.000000000000000000, 0.000000000000000000 ) ) ;
#50063=CARTESIAN_POINT ( 'NONE',  ( -339.1964088526558498, -102.6919536717982737, -56.27632902032089390 ) ) ;
#50072=EDGE_CURVE ( 'NONE', #15026, #20985, #14670, .T. ) ;
#50073=DIRECTION ( 'NONE',  ( -0.9993908270190956511, 4.273955692857142571E-18, -0.03489949670250096919 ) ) ;
#50075=ORIENTED_EDGE ( 'NONE', *, *, #24061, .F. ) ;
#50077=ADVANCED_FACE ( 'NONE', ( #23073 ), #14169, .F. ) ;
#50082=AXIS2_PLACEMENT_3D ( 'NONE', #20075, #24533, #44258 ) ;
#50085=FACE_OUTER_BOUND ( 'NONE', #42880, .T. ) ;
#50091=CARTESIAN_POINT ( 'NONE',  ( -339.1964088526558498, -74.65991953890826949, 33.10432812419072945 ) ) ;
#50094=EDGE_CURVE ( 'NONE', #10964, #37735, #38581, .T. ) ;
#50098=LINE ( 'NONE', #30887, #43756 ) ;
#50103=LINE ( 'NONE', #21969, #36617 ) ;
#50104=CARTESIAN_POINT ( 'NONE',  ( -339.1964088526558498, -108.8949048983204051, 57.16590939599314680 ) ) ;
#50108=AXIS2_PLACEMENT_3D ( 'NONE', #20606, #36643, #16159 ) ;
#50120=DIRECTION ( 'NONE',  ( 1.000000000000000000, 0.000000000000000000, 0.000000000000000000 ) ) ;
#50122=LINE ( 'NONE', #26706, #22099 ) ;
#50128=LINE ( 'NONE', #37756, #30248 ) ;
#50129=CARTESIAN_POINT ( 'NONE',  ( -339.1964088526558498, -101.7569374291119857, 55.92172413327800484 ) ) ;
#50134=CARTESIAN_POINT ( 'NONE',  ( -332.3517673607765914, -141.9604555052315220, 56.09938080879057765 ) ) ;
#50144=ORIENTED_EDGE ( 'NONE', *, *, #13746, .F. ) ;
#50145=DIRECTION ( 'NONE',  ( 0.000000000000000000, -0.1205366802553303196, -0.9927088740980530845 ) ) ;
#50146=VERTEX_POINT ( 'NONE', #46474 ) ;
#50148=ORIENTED_EDGE ( 'NONE', *, *, #1573, .T. ) ;
#50150=LINE ( 'NONE', #12624, #39975 ) ;
#50151=VERTEX_POINT ( 'NONE', #28029 ) ;
#50152=FACE_OUTER_BOUND ( 'NONE', #21093, .T. ) ;
#50153=ORIENTED_EDGE ( 'NONE', *, *, #2157, .T. ) ;
#50154=AXIS2_PLACEMENT_3D ( 'NONE', #14435, #42536, #6558 ) ;
#50156=CARTESIAN_POINT ( 'NONE',  ( -336.3521761649654422, -159.7173995167596559, -47.83617848703447351 ) ) ;
#50158=DIRECTION ( 'NONE',  ( 0.000000000000000000, 0.000000000000000000, 1.000000000000000000 ) ) ;
#50162=VECTOR ( 'NONE', #34287, 1000.000000000000000 ) ;
#50163=DIRECTION ( 'NONE',  ( 0.000000000000000000, 0.000000000000000000, 1.000000000000000000 ) ) ;
#50165=CARTESIAN_POINT ( 'NONE',  ( -339.1964088526558498, -182.5000000000000568, 0.5000000000000457412 ) ) ;
#50167=EDGE_LOOP ( 'NONE', ( #51974, #19306, #15653, #15753 ) ) ;
#50174=CARTESIAN_POINT ( 'NONE',  ( -330.4913330509368166, -89.57268800991444380, 48.27201571435978877 ) ) ;
#50181=ORIENTED_EDGE ( 'NONE', *, *, #41552, .F. ) ;
#50182=ADVANCED_FACE ( 'NONE', ( #19900 ), #7304, .F. ) ;
#50184=EDGE_LOOP ( 'NONE', ( #50218, #36721, #39347, #19942 ) ) ;
#50189=AXIS2_PLACEMENT_3D ( 'NONE', #47558, #23619, #19175 ) ;
#50192=VECTOR ( 'NONE', #1440, 1000.000000000000000 ) ;
#50195=ORIENTED_EDGE ( 'NONE', *, *, #20205, .T. ) ;
#50204=DIRECTION ( 'NONE',  ( 0.000000000000000000, 0.000000000000000000, 1.000000000000000000 ) ) ;
#50210=CARTESIAN_POINT ( 'NONE',  ( -339.1964088526558498, -173.1613497474970700, -33.67120938215281001 ) ) ;
#50212=DIRECTION ( 'NONE',  ( -0.000000000000000000, -1.000000000000000000, -0.000000000000000000 ) ) ;
#50216=CARTESIAN_POINT ( 'NONE',  ( -339.1964088526558498, -79.66942718702493664, 39.49849221029193558 ) ) ;
#50217=ORIENTED_EDGE ( 'NONE', *, *, #28112, .F. ) ;
#50218=ORIENTED_EDGE ( 'NONE', *, *, #37934, .T. ) ;
#50220=AXIS2_PLACEMENT_3D ( 'NONE', #38936, #18216, #11083 ) ;
#50222=CARTESIAN_POINT ( 'NONE',  ( -332.3517673607765914, -72.48138011061176655, -29.74944317415788930 ) ) ;
#50224=DIRECTION ( 'NONE',  ( 0.000000000000000000, -1.047444401652940007E-14, -1.000000000000000000 ) ) ;
#50226=AXIS2_PLACEMENT_3D ( 'NONE', #30272, #15280, #43127 ) ;
#50228=CARTESIAN_POINT ( 'NONE',  ( -336.3521761649654422, -77.59233547837267508, 37.15394033962009246 ) ) ;
#50231=VECTOR ( 'NONE', #49429, 1000.000000000000000 ) ;
#50234=LINE ( 'NONE', #49189, #43076 ) ;
#50239=VECTOR ( 'NONE', #46001, 1000.000000000000114 ) ;
#50240=LINE ( 'NONE', #25021, #18104 ) ;
#50241=CARTESIAN_POINT ( 'NONE',  ( -339.1964088526558498, -103.0458197858333165, -55.34326076196084188 ) ) ;
#50243=EDGE_CURVE ( 'NONE', #21929, #46650, #12265, .T. ) ;
#50244=DIRECTION ( 'NONE',  ( 0.000000000000000000, 0.1205366802553199113, -0.9927088740980544168 ) ) ;
#50254=ORIENTED_EDGE ( 'NONE', *, *, #10665, .T. ) ;
#50255=VECTOR ( 'NONE', #42715, 1000.000000000000000 ) ;
#50259=EDGE_CURVE ( 'NONE', #19072, #6572, #15717, .T. ) ;
#50261=CIRCLE ( 'NONE', #24249, 60.00000000000000000 ) ;
#50264=ORIENTED_EDGE ( 'NONE', *, *, #18951, .T. ) ;
#50266=DIRECTION ( 'NONE',  ( -0.000000000000000000, -0.9709418174260526779, -0.2393156642875547968 ) ) ;
#50270=ORIENTED_EDGE ( 'NONE', *, *, #2527, .T. ) ;
#50273=DIRECTION ( 'NONE',  ( 1.000000000000000000, -0.000000000000000000, -0.000000000000000000 ) ) ;
#50275=DIRECTION ( 'NONE',  ( -0.000000000000000000, -0.1205366802553130001, 0.9927088740980551940 ) ) ;
#50277=DIRECTION ( 'NONE',  ( 1.000000000000000000, 0.000000000000000000, 0.000000000000000000 ) ) ;
#50280=ORIENTED_EDGE ( 'NONE', *, *, #23356, .F. ) ;
#50284=FACE_OUTER_BOUND ( 'NONE', #44326, .T. ) ;
#50285=DIRECTION ( 'NONE',  ( 0.000000000000000000, -0.9350162426854169428, -0.3546048870425300148 ) ) ;
#50289=PLANE ( 'NONE',  #36532 ) ;
#50291=CARTESIAN_POINT ( 'NONE',  ( -339.1964088526558498, -137.1341532842531876, -57.40522506028080585 ) ) ;
#50292=ORIENTED_EDGE ( 'NONE', *, *, #51004, .F. ) ;
#50303=ADVANCED_FACE ( 'NONE', ( #39592 ), #27523, .F. ) ;
#50304=EDGE_LOOP ( 'NONE', ( #45170, #16457, #7561, #44700 ) ) ;
#50305=CARTESIAN_POINT ( 'NONE',  ( 0.000000000000000000, -66.21443277186274656, 14.11962419296515137 ) ) ;
#50306=EDGE_LOOP ( 'NONE', ( #40820, #27721, #49724, #34768 ) ) ;
#50307=VECTOR ( 'NONE', #3559, 1000.000000000000000 ) ;
#50309=PLANE ( 'NONE',  #35352 ) ;
#50310=CARTESIAN_POINT ( 'NONE',  ( -332.3517673607765914, -160.6539403396202772, 45.90766452162722544 ) ) ;
#50313=ORIENTED_EDGE ( 'NONE', *, *, #43260, .F. ) ;
#50314=AXIS2_PLACEMENT_3D ( 'NONE', #43899, #7896, #7406 ) ;
#50315=PLANE ( 'NONE',  #51797 ) ;
#50319=PLANE ( 'NONE',  #4638 ) ;
#50327=ORIENTED_EDGE ( 'NONE', *, *, #39729, .T. ) ;
#50333=ORIENTED_EDGE ( 'NONE', *, *, #46202, .T. ) ;
#50334=AXIS2_PLACEMENT_3D ( 'NONE', #1050, #13666, #29686 ) ;
#50335=CARTESIAN_POINT ( 'NONE',  ( -336.3521761649654422, -174.9833430614318388, 28.86398714850502856 ) ) ;
#50337=ORIENTED_EDGE ( 'NONE', *, *, #33962, .F. ) ;
#50339=DIRECTION ( 'NONE',  ( 0.000000000000000000, 0.9350162426854132791, -0.3546048870425396182 ) ) ;
#50340=EDGE_CURVE ( 'NONE', #42116, #50802, #47508, .T. ) ;
#50341=PLANE ( 'NONE',  #42154 ) ;
#50343=ADVANCED_FACE ( 'NONE', ( #20156 ), #29065, .T. ) ;
#50347=VERTEX_POINT ( 'NONE', #45642 ) ;
#50348=EDGE_CURVE ( 'NONE', #2690, #6390, #711, .T. ) ;
#50353=VERTEX_POINT ( 'NONE', #37221 ) ;
#50362=ORIENTED_EDGE ( 'NONE', *, *, #7686, .T. ) ;
#50363=EDGE_CURVE ( 'NONE', #51994, #45030, #44155, .T. ) ;
#50365=DIRECTION ( 'NONE',  ( -0.000000000000000000, -0.8229838658936516893, 0.5680647467311626952 ) ) ;
#50369=LINE ( 'NONE', #42460, #36348 ) ;
#50381=ORIENTED_EDGE ( 'NONE', *, *, #3037, .F. ) ;
#50382=EDGE_LOOP ( 'NONE', ( #17308, #31855, #48322, #44696 ) ) ;
#50386=CARTESIAN_POINT ( 'NONE',  ( -332.3517673607765914, -69.63373947859463442, 26.42775013958025454 ) ) ;
#50387=DIRECTION ( 'NONE',  ( -0.000000000000000000, -0.3546048870425396182, -0.9350162426854132791 ) ) ;
#50391=DIRECTION ( 'NONE',  ( 0.000000000000000000, 0.000000000000000000, 1.000000000000000000 ) ) ;
#50400=CARTESIAN_POINT ( 'NONE',  ( -305.0000000000000568, -78.25935320507949200, -39.41172259083896279 ) ) ;
#50402=EDGE_CURVE ( 'NONE', #20303, #39961, #4921, .T. ) ;
#50413=CARTESIAN_POINT ( 'NONE',  ( -332.3517673607765914, -165.9166037625627439, 41.09453333279358134 ) ) ;
#50414=DIRECTION ( 'NONE',  ( -0.000000000000000000, -3.491481338843133355E-15, -1.000000000000000000 ) ) ;
#50416=ADVANCED_FACE ( 'NONE', ( #21195 ), #45384, .F. ) ;
#50417=DIRECTION ( 'NONE',  ( -0.000000000000000000, 0.4647231720437755564, 0.8854560256532062468 ) ) ;
#50436=EDGE_CURVE ( 'NONE', #16821, #16432, #22225, .T. ) ;
#50440=EDGE_CURVE ( 'NONE', #38472, #28072, #22748, .T. ) ;
#50443=DIRECTION ( 'NONE',  ( 1.000000000000000000, 0.000000000000000000, 0.000000000000000000 ) ) ;
#50445=PLANE ( 'NONE',  #50154 ) ;
#50450=ORIENTED_EDGE ( 'NONE', *, *, #27726, .F. ) ;
#50454=VECTOR ( 'NONE', #10794, 1000.000000000000000 ) ;
#50455=VECTOR ( 'NONE', #24683, 1000.000000000000114 ) ;
#50456=DIRECTION ( 'NONE',  ( -8.718379230999707126E-17, -0.6631226582408017434, -0.7485107481710954191 ) ) ;
#50461=VERTEX_POINT ( 'NONE', #42452 ) ;
#50463=ORIENTED_EDGE ( 'NONE', *, *, #6677, .T. ) ;
#50465=EDGE_LOOP ( 'NONE', ( #12388, #24528, #50217, #47151 ) ) ;
#50467=ADVANCED_FACE ( 'NONE', ( #14606 ), #42725, .F. ) ;
#50469=DIRECTION ( 'NONE',  ( -0.000000000000000000, 0.8854560256532157947, 0.4647231720437573488 ) ) ;
#50475=LINE ( 'NONE', #30235, #17804 ) ;
#50478=ORIENTED_EDGE ( 'NONE', *, *, #37537, .T. ) ;
#50481=CARTESIAN_POINT ( 'NONE',  ( -365.0000000000001137, -78.50000000000002842, 5.000000000000001776 ) ) ;
#50482=FACE_OUTER_BOUND ( 'NONE', #12689, .T. ) ;
#50491=DIRECTION ( 'NONE',  ( -0.000000000000000000, -0.9350162426854121689, 0.3546048870425426158 ) ) ;
#50493=VECTOR ( 'NONE', #18549, 1000.000000000000114 ) ;
#50496=EDGE_LOOP ( 'NONE', ( #27280, #40780, #42863, #17798 ) ) ;
#50498=ADVANCED_FACE ( 'NONE', ( #26692 ), #10141, .F. ) ;
#50508=VERTEX_POINT ( 'NONE', #49840 ) ;
#50510=VECTOR ( 'NONE', #34350, 1000.000000000000000 ) ;
#50512=DIRECTION ( 'NONE',  ( -0.000000000000000000, 0.9927088740980556381, 0.1205366802553095307 ) ) ;
#50516=FACE_OUTER_BOUND ( 'NONE', #2452, .T. ) ;
#50518=DIRECTION ( 'NONE',  ( -0.000000000000000000, -0.3546048870425396182, -0.9350162426854132791 ) ) ;
#50523=DIRECTION ( 'NONE',  ( 1.000000000000000000, 0.000000000000000000, 0.000000000000000000 ) ) ;
#50524=VECTOR ( 'NONE', #42574, 1000.000000000000000 ) ;
#50526=EDGE_CURVE ( 'NONE', #14314, #8372, #50103, .T. ) ;
#50527=FACE_OUTER_BOUND ( 'NONE', #22520, .T. ) ;
#50532=VERTEX_POINT ( 'NONE', #30893 ) ;
#50534=FACE_OUTER_BOUND ( 'NONE', #36681, .T. ) ;
#50539=DIRECTION ( 'NONE',  ( -1.000000000000000000, 0.000000000000000000, 0.000000000000000000 ) ) ;
#50546=VECTOR ( 'NONE', #9861, 1000.000000000000000 ) ;
#50547=CARTESIAN_POINT ( 'NONE',  ( -339.1964088526558498, -171.7720157143598669, 33.92731199008546383 ) ) ;
#50548=DIRECTION ( 'NONE',  ( 1.000000000000000000, -0.000000000000000000, -0.000000000000000000 ) ) ;
#50554=ORIENTED_EDGE ( 'NONE', *, *, #21689, .F. ) ;
#50557=LINE ( 'NONE', #6671, #43757 ) ;
#50559=CARTESIAN_POINT ( 'NONE',  ( -332.3517673607765914, -176.9651911376907094, -25.08789112700655721 ) ) ;
#50562=DIRECTION ( 'NONE',  ( -0.000000000000000000, 0.9927088740980553050, 0.1205366802553130001 ) ) ;
#50567=ORIENTED_EDGE ( 'NONE', *, *, #18546, .T. ) ;
#50572=LINE ( 'NONE', #26653, #43366 ) ;
#50574=ORIENTED_EDGE ( 'NONE', *, *, #9960, .T. ) ;
#50576=EDGE_LOOP ( 'NONE', ( #22085, #14056, #40341, #44898 ) ) ;
#50577=EDGE_CURVE ( 'NONE', #37919, #16257, #14100, .T. ) ;
#50582=FACE_OUTER_BOUND ( 'NONE', #13613, .T. ) ;
#50585=ADVANCED_FACE ( 'NONE', ( #30116 ), #25649, .T. ) ;
#50587=DIRECTION ( 'NONE',  ( -0.000000000000000000, 0.9350162426854194964, 0.3546048870425235200 ) ) ;
#50590=VERTEX_POINT ( 'NONE', #31141 ) ;
#50591=VERTEX_POINT ( 'NONE', #42969 ) ;
#50592=DIRECTION ( 'NONE',  ( 0.000000000000000000, -0.1205366802553268640, -0.9927088740980535286 ) ) ;
#50596=VECTOR ( 'NONE', #9364, 1000.000000000000000 ) ;
#50597=DIRECTION ( 'NONE',  ( 0.000000000000000000, 0.000000000000000000, 1.000000000000000000 ) ) ;
#50604=FACE_OUTER_BOUND ( 'NONE', #30409, .T. ) ;
#50605=EDGE_CURVE ( 'NONE', #4319, #45025, #31395, .T. ) ;
#50608=CARTESIAN_POINT ( 'NONE',  ( -336.3521761649654422, -73.44864141332200802, 31.34948880313848107 ) ) ;
#50617=ORIENTED_EDGE ( 'NONE', *, *, #37759, .F. ) ;
#50621=VERTEX_POINT ( 'NONE', #7748 ) ;
#50627=DIRECTION ( 'NONE',  ( 0.000000000000000000, 0.000000000000000000, -1.000000000000000000 ) ) ;
#50628=VECTOR ( 'NONE', #37343, 1000.000000000000114 ) ;
#50629=EDGE_CURVE ( 'NONE', #50821, #3974, #27457, .T. ) ;
#50631=DIRECTION ( 'NONE',  ( -1.000000000000000000, 0.000000000000000000, 0.000000000000000000 ) ) ;
#50640=DIRECTION ( 'NONE',  ( 1.000000000000000000, 0.000000000000000000, 0.000000000000000000 ) ) ;
#50643=EDGE_CURVE ( 'NONE', #16559, #38969, #3802, .T. ) ;
#50644=VECTOR ( 'NONE', #20259, 1000.000000000000000 ) ;
#50649=ORIENTED_EDGE ( 'NONE', *, *, #3186, .T. ) ;
#50656=EDGE_CURVE ( 'NONE', #18494, #37026, #29109, .T. ) ;
#50658=LINE ( 'NONE', #22271, #16706 ) ;
#50661=ORIENTED_EDGE ( 'NONE', *, *, #9737, .F. ) ;
#50668=AXIS2_PLACEMENT_3D ( 'NONE', #20470, #23891, #491 ) ;
#50676=AXIS2_PLACEMENT_3D ( 'NONE', #19131, #42781, #2831 ) ;
#50686=LINE ( 'NONE', #47782, #27613 ) ;
#50687=DIRECTION ( 'NONE',  ( -1.000000000000000000, 0.000000000000000000, 0.000000000000000000 ) ) ;
#50694=VERTEX_POINT ( 'NONE', #6977 ) ;
#50697=EDGE_LOOP ( 'NONE', ( #20170, #3085 ) ) ;
#50713=EDGE_CURVE ( 'NONE', #37730, #20241, #369, .T. ) ;
#50714=DIRECTION ( 'NONE',  ( 1.000000000000000000, -0.000000000000000000, -0.000000000000000000 ) ) ;
#50716=DIRECTION ( 'NONE',  ( -1.000000000000000000, 0.000000000000000000, 0.000000000000000000 ) ) ;
#50717=ORIENTED_EDGE ( 'NONE', *, *, #18270, .T. ) ;
#50726=EDGE_CURVE ( 'NONE', #45363, #40953, #17197, .T. ) ;
#50728=VERTEX_POINT ( 'NONE', #12196 ) ;
#50742=DIRECTION ( 'NONE',  ( 1.000000000000000000, 5.781354811211829468E-17, -6.525800561035010214E-17 ) ) ;
#50746=VECTOR ( 'NONE', #32608, 1000.000000000000000 ) ;
#50749=DIRECTION ( 'NONE',  ( -1.000000000000000000, -3.701062773504881123E-15, -9.758900497077147268E-15 ) ) ;
#50752=DIRECTION ( 'NONE',  ( 1.000000000000000000, 0.000000000000000000, 0.000000000000000000 ) ) ;
#50753=DIRECTION ( 'NONE',  ( 0.000000000000000000, 0.3546048870425235200, -0.9350162426854194964 ) ) ;
#50758=ADVANCED_FACE ( 'NONE', ( #36906 ), #20609, .F. ) ;
#50762=EDGE_CURVE ( 'NONE', #13489, #29626, #16423, .T. ) ;
#50765=ORIENTED_EDGE ( 'NONE', *, *, #25910, .F. ) ;
#50766=EDGE_LOOP ( 'NONE', ( #46693, #12003, #11262, #18918 ) ) ;
#50767=LINE ( 'NONE', #3192, #693 ) ;
#50769=DIRECTION ( 'NONE',  ( -1.000000000000000000, 0.000000000000000000, 0.000000000000000000 ) ) ;
#50771=FACE_OUTER_BOUND ( 'NONE', #11722, .T. ) ;
#50774=CARTESIAN_POINT ( 'NONE',  ( -339.1964088526558498, -123.5000000000000284, 0.000000000000000000 ) ) ;
#50775=ORIENTED_EDGE ( 'NONE', *, *, #27247, .T. ) ;
#50778=DIRECTION ( 'NONE',  ( -0.000000000000000000, 0.3546048870425463906, 0.9350162426854107256 ) ) ;
#50784=CARTESIAN_POINT ( 'NONE',  ( -332.3517673607765914, -105.0395444947681369, -56.09938080879045685 ) ) ;
#50787=ADVANCED_FACE ( 'NONE', ( #37154 ), #32440, .F. ) ;
#50789=LINE ( 'NONE', #6651, #40734 ) ;
#50794=VECTOR ( 'NONE', #20363, 1000.000000000000000 ) ;
#50795=CARTESIAN_POINT ( 'NONE',  ( -332.3517673607765914, -182.8437365148560616, 8.849911663702917153 ) ) ;
#50799=DIRECTION ( 'NONE',  ( 0.000000000000000000, -0.8854560256532157947, -0.4647231720437573488 ) ) ;
#50800=AXIS2_PLACEMENT_3D ( 'NONE', #25492, #33887, #22318 ) ;
#50802=VERTEX_POINT ( 'NONE', #12461 ) ;
#50805=CARTESIAN_POINT ( 'NONE',  ( 0.000000000000000000, -180.7855672281370119, 14.11962419296635396 ) ) ;
#50807=ORIENTED_EDGE ( 'NONE', *, *, #28215, .T. ) ;
#50811=EDGE_CURVE ( 'NONE', #19283, #40712, #31623, .T. ) ;
#50813=PLANE ( 'NONE',  #16175 ) ;
#50814=VECTOR ( 'NONE', #19751, 1000.000000000000000 ) ;
#50821=VERTEX_POINT ( 'NONE', #16694 ) ;
#50823=EDGE_CURVE ( 'NONE', #41662, #46894, #41351, .T. ) ;
#50828=DIRECTION ( 'NONE',  ( 0.000000000000000000, -6.753856733136369375E-14, -1.000000000000000000 ) ) ;
#50831=CARTESIAN_POINT ( 'NONE',  ( -330.4913330509368166, -73.83865025250280212, 33.67120938215256132 ) ) ;
#50833=AXIS2_PLACEMENT_3D ( 'NONE', #44949, #21025, #16577 ) ;
#50836=LINE ( 'NONE', #1704, #19060 ) ;
#50838=VERTEX_POINT ( 'NONE', #25335 ) ;
#50852=ORIENTED_EDGE ( 'NONE', *, *, #36982, .F. ) ;
#50853=FACE_OUTER_BOUND ( 'NONE', #51272, .T. ) ;
#50854=VECTOR ( 'NONE', #25463, 1000.000000000000000 ) ;
#50857=CARTESIAN_POINT ( 'NONE',  ( -330.4913330509368166, -124.0000000000001990, -59.00000000000002132 ) ) ;
#50858=VECTOR ( 'NONE', #32866, 1000.000000000000000 ) ;
#50859=VECTOR ( 'NONE', #46595, 1000.000000000000114 ) ;
#50863=DIRECTION ( 'NONE',  ( -0.000000000000000000, -0.7485107481710977506, 0.6631226582407989678 ) ) ;
#50869=VECTOR ( 'NONE', #25088, 1000.000000000000114 ) ;
#50872=CARTESIAN_POINT ( 'NONE',  ( -332.3517673607765914, -158.9146170832377720, -48.43351006119259949 ) ) ;
#50876=CARTESIAN_POINT ( 'NONE',  ( -339.1964088526558498, -90.39567187580801999, 48.84008046109089918 ) ) ;
#50880=LINE ( 'NONE', #23009, #969 ) ;
#50884=EDGE_CURVE ( 'NONE', #47574, #34020, #1939, .T. ) ;
#50887=EDGE_CURVE ( 'NONE', #23810, #9413, #3913, .T. ) ;
#50892=PLANE ( 'NONE',  #38022 ) ;
#50901=ORIENTED_EDGE ( 'NONE', *, *, #10035, .T. ) ;
#50903=CARTESIAN_POINT ( 'NONE',  ( -336.3521761649654422, -119.0014323656137947, -58.88711093124865670 ) ) ;
#50904=FACE_OUTER_BOUND ( 'NONE', #3629, .T. ) ;
#50907=EDGE_CURVE ( 'NONE', #28554, #8596, #17364, .T. ) ;
#50911=AXIS2_PLACEMENT_3D ( 'NONE', #18356, #26741, #34374 ) ;
#50912=DIRECTION ( 'NONE',  ( -0.000000000000000000, 0.9709418174260519008, -0.2393156642875582940 ) ) ;
#50913=ORIENTED_EDGE ( 'NONE', *, *, #27009, .F. ) ;
#50916=ORIENTED_EDGE ( 'NONE', *, *, #38870, .T. ) ;
#50928=FACE_OUTER_BOUND ( 'NONE', #9565, .T. ) ;
#50930=PLANE ( 'NONE',  #2104 ) ;
#50931=AXIS2_PLACEMENT_3D ( 'NONE', #8456, #4010, #20542 ) ;
#50934=ORIENTED_EDGE ( 'NONE', *, *, #10158, .T. ) ;
#50938=EDGE_CURVE ( 'NONE', #5668, #45033, #14010, .T. ) ;
#50942=ORIENTED_EDGE ( 'NONE', *, *, #44753, .T. ) ;
#50949=CARTESIAN_POINT ( 'NONE',  ( -336.3521761649654422, -92.15051119686104641, -50.05135858667769355 ) ) ;
#50953=ORIENTED_EDGE ( 'NONE', *, *, #3102, .T. ) ;
#50960=CARTESIAN_POINT ( 'NONE',  ( -332.3517673607765914, -93.75055682584159911, 51.01861988938794923 ) ) ;
#50961=EDGE_CURVE ( 'NONE', #13339, #29051, #25582, .T. ) ;
#50965=ORIENTED_EDGE ( 'NONE', *, *, #1293, .F. ) ;
#50967=CARTESIAN_POINT ( 'NONE',  ( -336.3521761649654422, -145.9479049231020440, -54.58714071513102795 ) ) ;
#50969=AXIS2_PLACEMENT_3D ( 'NONE', #51853, #22109, #25275 ) ;
#50978=ORIENTED_EDGE ( 'NONE', *, *, #4506, .T. ) ;
#50979=VECTOR ( 'NONE', #27156, 1000.000000000000000 ) ;
#50980=VECTOR ( 'NONE', #40531, 1000.000000000000000 ) ;
#50990=DIRECTION ( 'NONE',  ( 0.000000000000000000, -0.9350162426854169428, -0.3546048870425300148 ) ) ;
#50991=VERTEX_POINT ( 'NONE', #22878 ) ;
#51002=CARTESIAN_POINT ( 'NONE',  ( -365.0000000000001137, -168.5000000000000284, 0.000000000000000000 ) ) ;
#51004=EDGE_CURVE ( 'NONE', #13064, #46003, #50150, .T. ) ;
#51009=CARTESIAN_POINT ( 'NONE',  ( -339.1964088526558498, -66.09477493971894546, 13.63415328425207917 ) ) ;
#51010=EDGE_CURVE ( 'NONE', #21717, #1947, #32609, .T. ) ;
#51018=ADVANCED_FACE ( 'NONE', ( #40476 ), #16596, .F. ) ;
#51021=CARTESIAN_POINT ( 'NONE',  ( -305.0000000000000568, -70.60684477890951882, 28.32515014536777187 ) ) ;
#51025=EDGE_CURVE ( 'NONE', #16663, #5355, #45238, .T. ) ;
#51030=DIRECTION ( 'NONE',  ( -0.000000000000000000, 0.2393156642875685636, 0.9709418174260492362 ) ) ;
#51032=CARTESIAN_POINT ( 'NONE',  ( -339.1964088526558498, -75.22798428563991990, -33.92731199008514409 ) ) ;
#51033=AXIS2_PLACEMENT_3D ( 'NONE', #31641, #43988, #51898 ) ;
#51035=ORIENTED_EDGE ( 'NONE', *, *, #3115, .F. ) ;
#51036=DIRECTION ( 'NONE',  ( -1.000000000000000000, 0.000000000000000000, 0.000000000000000000 ) ) ;
#51040=VERTEX_POINT ( 'NONE', #16855 ) ;
#51042=CARTESIAN_POINT ( 'NONE',  ( -339.1964088526558498, -103.0458197858333165, -55.34326076196084188 ) ) ;
#51046=PLANE ( 'NONE',  #11598 ) ;
#51049=CARTESIAN_POINT ( 'NONE',  ( -339.1964088526558498, -172.3400804610915600, -33.10432812419107051 ) ) ;
#51055=VECTOR ( 'NONE', #16370, 1000.000000000000000 ) ;
#51057=FACE_OUTER_BOUND ( 'NONE', #41719, .T. ) ;
#51062=ADVANCED_FACE ( 'NONE', ( #2308 ), #21303, .F. ) ;
#51064=EDGE_LOOP ( 'NONE', ( #44761, #47424, #23980, #46072 ) ) ;
#51067=ORIENTED_EDGE ( 'NONE', *, *, #43483, .T. ) ;
#51075=CARTESIAN_POINT ( 'NONE',  ( -330.4913330509368166, -64.86990808808717190, -6.615309698015095385 ) ) ;
#51079=CARTESIAN_POINT ( 'NONE',  ( -332.3517673607765914, -176.5004679656469477, -25.97334715265976612 ) ) ;
#51080=ORIENTED_EDGE ( 'NONE', *, *, #39749, .T. ) ;
#51081=CARTESIAN_POINT ( 'NONE',  ( -340.0000000000000568, -78.50000000000002842, -5.000000000000001776 ) ) ;
#51089=VERTEX_POINT ( 'NONE', #14647 ) ;
#51094=VECTOR ( 'NONE', #12293, 1000.000000000000000 ) ;
#51097=CARTESIAN_POINT ( 'NONE',  ( -339.1964088526558498, -123.0000000000002700, -59.00000000000002132 ) ) ;
#51100=EDGE_CURVE ( 'NONE', #42455, #21438, #31438, .T. ) ;
#51101=EDGE_LOOP ( 'NONE', ( #16260, #2255, #21347, #7652 ) ) ;
#51106=AXIS2_PLACEMENT_3D ( 'NONE', #47220, #2792, #46694 ) ;
#51108=CARTESIAN_POINT ( 'NONE',  ( -336.3521761649654422, -181.1761995186066088, -12.53476669029101842 ) ) ;
#51110=CARTESIAN_POINT ( 'NONE',  ( -332.3517673607765914, -182.3871109312487420, -4.498567634386014369 ) ) ;
#51114=ORIENTED_EDGE ( 'NONE', *, *, #27684, .F. ) ;
#51116=ORIENTED_EDGE ( 'NONE', *, *, #40074, .T. ) ;
#51119=LINE ( 'NONE', #47156, #50979 ) ;
#51121=DIRECTION ( 'NONE',  ( -0.000000000000000000, 0.2393156642875582940, 0.9709418174260519008 ) ) ;
#51128=ORIENTED_EDGE ( 'NONE', *, *, #22174, .T. ) ;
#51134=CARTESIAN_POINT ( 'NONE',  ( -339.1964088526558498, -182.0095552316575152, 7.608018572113563138 ) ) ;
#51137=DIRECTION ( 'NONE',  ( 1.000000000000000000, -8.718379230999705894E-17, 9.132017516997905925E-31 ) ) ;
#51141=VERTEX_POINT ( 'NONE', #38800 ) ;
#51144=LINE ( 'NONE', #39007, #28666 ) ;
#51151=CARTESIAN_POINT ( 'NONE',  ( -339.1964088526558498, -157.4273119900845757, 48.27201571436049932 ) ) ;
#51152=VERTEX_POINT ( 'NONE', #19114 ) ;
#51154=CARTESIAN_POINT ( 'NONE',  ( -339.1964088526558498, -89.57268800991437274, 48.27201571435973904 ) ) ;
#51158=LINE ( 'NONE', #46170, #51480 ) ;
#51159=ORIENTED_EDGE ( 'NONE', *, *, #51573, .F. ) ;
#51171=ORIENTED_EDGE ( 'NONE', *, *, #33174, .F. ) ;
#51172=ORIENTED_EDGE ( 'NONE', *, *, #43323, .T. ) ;
#51177=CARTESIAN_POINT ( 'NONE',  ( -339.1964088526558498, -84.00150778970767362, -43.83057281297470098 ) ) ;
#51179=ORIENTED_EDGE ( 'NONE', *, *, #8938, .F. ) ;
#51187=DIRECTION ( 'NONE',  ( 0.000000000000000000, -0.9709418174260519008, 0.2393156642875582940 ) ) ;
#51190=DIRECTION ( 'NONE',  ( -1.000000000000000000, -8.589602288500793681E-15, 5.928974370888963984E-15 ) ) ;
#51194=ORIENTED_EDGE ( 'NONE', *, *, #48696, .F. ) ;
#51195=DIRECTION ( 'NONE',  ( -0.000000000000000000, 0.4647231720437789981, 0.8854560256532044704 ) ) ;
#51198=LINE ( 'NONE', #39842, #20273 ) ;
#51200=FACE_OUTER_BOUND ( 'NONE', #50766, .T. ) ;
#51202=DIRECTION ( 'NONE',  ( -0.000000000000000000, -0.9350162426854121689, 0.3546048870425426158 ) ) ;
#51226=EDGE_LOOP ( 'NONE', ( #7424, #15301, #16396, #34682 ) ) ;
#51231=LINE ( 'NONE', #6818, #44189 ) ;
#51233=DIRECTION ( 'NONE',  ( -1.000000000000000000, -7.812315528781839335E-15, 6.921107616850815004E-15 ) ) ;
#51241=DIRECTION ( 'NONE',  ( 0.000000000000000000, -0.1205366802553095168, 0.9927088740980556381 ) ) ;
#51242=ORIENTED_EDGE ( 'NONE', *, *, #36834, .F. ) ;
#51249=CARTESIAN_POINT ( 'NONE',  ( -339.1964088526558498, -123.5000000000000284, 0.000000000000000000 ) ) ;
#51250=ORIENTED_EDGE ( 'NONE', *, *, #22270, .F. ) ;
#51253=CARTESIAN_POINT ( 'NONE',  ( -330.4913330509368166, -123.5000000000000284, -60.00000000000000000 ) ) ;
#51256=CARTESIAN_POINT ( 'NONE',  ( -330.4913330509368166, -157.9941932480463436, 49.09328500076600932 ) ) ;
#51272=EDGE_LOOP ( 'NONE', ( #39385, #7924, #11930, #28714 ) ) ;
#51275=DIRECTION ( 'NONE',  ( -0.000000000000000000, -0.7485107481710953081, 0.6631226582408016323 ) ) ;
#51279=CARTESIAN_POINT ( 'NONE',  ( -332.3517673607765914, -66.84438072661991725, -16.67542351306652648 ) ) ;
#51284=EDGE_CURVE ( 'NONE', #6162, #14589, #20651, .T. ) ;
#51289=FACE_OUTER_BOUND ( 'NONE', #19803, .T. ) ;
#51291=CARTESIAN_POINT ( 'NONE',  ( -339.1964088526558498, -103.0458197858324496, 55.34326076196052213 ) ) ;
#51297=VERTEX_POINT ( 'NONE', #8556 ) ;
#51300=CARTESIAN_POINT ( 'NONE',  ( -339.1964088526558498, -115.8919814278862503, 58.50955523165745831 ) ) ;
#51302=PLANE ( 'NONE',  #20652 ) ;
#51308=ADVANCED_FACE ( 'NONE', ( #32485 ), #24095, .F. ) ;
#51316=FACE_BOUND ( 'NONE', #16424, .T. ) ;
#51317=DIRECTION ( 'NONE',  ( 1.043714542225393381E-14, 0.3546048870425235200, -0.9350162426854194964 ) ) ;
#51324=ORIENTED_EDGE ( 'NONE', *, *, #1266, .F. ) ;
#51335=ORIENTED_EDGE ( 'NONE', *, *, #25022, .T. ) ;
#51340=ORIENTED_EDGE ( 'NONE', *, *, #46544, .F. ) ;
#51341=ORIENTED_EDGE ( 'NONE', *, *, #15580, .F. ) ;
#51349=EDGE_CURVE ( 'NONE', #34284, #42517, #43786, .T. ) ;
#51366=EDGE_CURVE ( 'NONE', #20985, #43547, #49824, .T. ) ;
#51369=ADVANCED_FACE ( 'NONE', ( #37723 ), #45624, .F. ) ;
#51372=AXIS2_PLACEMENT_3D ( 'NONE', #33933, #18183, #49487 ) ;
#51378=DIRECTION ( 'NONE',  ( -0.000000000000000000, -3.491481338843133355E-15, -1.000000000000000000 ) ) ;
#51386=CARTESIAN_POINT ( 'NONE',  ( -330.4913330509368166, -123.5000000000000284, 0.000000000000000000 ) ) ;
#51388=ORIENTED_EDGE ( 'NONE', *, *, #4709, .T. ) ;
#51390=DIRECTION ( 'NONE',  ( 0.000000000000000000, -0.1205366802553337752, -0.9927088740980526405 ) ) ;
#51392=CARTESIAN_POINT ( 'NONE',  ( -336.3521761649654422, -123.5000000000000284, 0.000000000000000000 ) ) ;
#51399=VERTEX_POINT ( 'NONE', #9355 ) ;
#51407=DIRECTION ( 'NONE',  ( 1.000000000000000000, -0.000000000000000000, -0.000000000000000000 ) ) ;
#51410=ORIENTED_EDGE ( 'NONE', *, *, #30764, .T. ) ;
#51423=ADVANCED_FACE ( 'NONE', ( #17238 ), #33775, .F. ) ;
#51424=CARTESIAN_POINT ( 'NONE',  ( 0.000000000000000000, -157.0158200571378018, 48.55604808772604741 ) ) ;
#51425=CARTESIAN_POINT ( 'NONE',  ( -332.3517673607765914, -76.43926241122620979, -35.68215131113738181 ) ) ;
#51427=FACE_OUTER_BOUND ( 'NONE', #28764, .T. ) ;
#51430=ORIENTED_EDGE ( 'NONE', *, *, #25944, .T. ) ;
#51432=CARTESIAN_POINT ( 'NONE',  ( -490.0000000000001137, -168.5000000000000284, 14.36509618646847386 ) ) ;
#51433=ORIENTED_EDGE ( 'NONE', *, *, #38414, .F. ) ;
#51436=ORIENTED_EDGE ( 'NONE', *, *, #29985, .F. ) ;
#51440=CARTESIAN_POINT ( 'NONE',  ( -332.3517673607765914, -128.9912765084839066, 58.76657425099337928 ) ) ;
#51442=DIRECTION ( 'NONE',  ( 0.000000000000000000, 0.9350162426854157216, 0.3546048870425330679 ) ) ;
#51445=EDGE_CURVE ( 'NONE', #21618, #4514, #29828, .T. ) ;
#51450=CARTESIAN_POINT ( 'NONE',  ( -336.3521761649654422, -92.15051119686104641, -50.05135858667769355 ) ) ;
#51451=DIRECTION ( 'NONE',  ( 0.000000000000000000, 0.8854560256532062468, -0.4647231720437755564 ) ) ;
#51458=ORIENTED_EDGE ( 'NONE', *, *, #43976, .T. ) ;
#51461=DIRECTION ( 'NONE',  ( 1.043714542225393539E-14, 0.6631226582408017434, 0.7485107481710954191 ) ) ;
#51463=CARTESIAN_POINT ( 'NONE',  ( -339.1964088526558498, -150.4759391377560576, -52.47426709956116042 ) ) ;
#51464=ORIENTED_EDGE ( 'NONE', *, *, #12434, .T. ) ;
#51465=AXIS2_PLACEMENT_3D ( 'NONE', #6430, #26376, #14832 ) ;
#51466=LINE ( 'NONE', #15466, #30984 ) ;
#51474=ORIENTED_EDGE ( 'NONE', *, *, #1810, .T. ) ;
#51479=LINE ( 'NONE', #35174, #42710 ) ;
#51480=VECTOR ( 'NONE', #19080, 1000.000000000000000 ) ;
#51482=EDGE_LOOP ( 'NONE', ( #26127, #41976, #28274, #23543 ) ) ;
#51484=PRESENTATION_STYLE_ASSIGNMENT (( #35433 ) ) ;
#51488=ORIENTED_EDGE ( 'NONE', *, *, #37041, .F. ) ;
#51489=LINE ( 'NONE', #35185, #18874 ) ;
#51490=CIRCLE ( 'NONE', #10336, 14.36509618646847386 ) ;
#51492=CARTESIAN_POINT ( 'NONE',  ( -332.3517673607765914, -80.42027357919624819, -40.34602258462219027 ) ) ;
#51496=VERTEX_POINT ( 'NONE', #33528 ) ;
#51498=LINE ( 'NONE', #38880, #38283 ) ;
#51504=DIRECTION ( 'NONE',  ( -0.9063077870366494926, 0.000000000000000000, 0.4226182617407002740 ) ) ;
#51506=ORIENTED_EDGE ( 'NONE', *, *, #27175, .F. ) ;
#51509=CARTESIAN_POINT ( 'NONE',  ( 0.000000000000000000, -182.5000000000000568, 0.000000000000000000 ) ) ;
#51515=CARTESIAN_POINT ( 'NONE',  ( -330.4913330509368166, -89.00580675195269009, 49.09328500076528456 ) ) ;
#51516=DIRECTION ( 'NONE',  ( -1.000000000000000000, 0.000000000000000000, 0.000000000000000000 ) ) ;
#51519=EDGE_LOOP ( 'NONE', ( #36877, #40414, #17054, #40370 ) ) ;
#51523=LINE ( 'NONE', #7389, #45466 ) ;
#51527=ORIENTED_EDGE ( 'NONE', *, *, #3459, .T. ) ;
#51528=EDGE_CURVE ( 'NONE', #36042, #10996, #46804, .T. ) ;
#51529=CARTESIAN_POINT ( 'NONE',  ( -305.0000000000000568, -123.5000000000000284, 0.000000000000000000 ) ) ;
#51531=CIRCLE ( 'NONE', #6219, 60.00000000000000000 ) ;
#51532=ORIENTED_EDGE ( 'NONE', *, *, #22028, .F. ) ;
#51533=ORIENTED_EDGE ( 'NONE', *, *, #19897, .T. ) ;
#51539=VERTEX_POINT ( 'NONE', #26401 ) ;
#51541=FACE_OUTER_BOUND ( 'NONE', #25361, .T. ) ;
#51543=DIRECTION ( 'NONE',  ( 1.000000000000000000, -0.000000000000000000, -0.000000000000000000 ) ) ;
#51546=DIRECTION ( 'NONE',  ( -0.000000000000000000, -0.8229838658936536877, 0.5680647467311596976 ) ) ;
#51548=FACE_OUTER_BOUND ( 'NONE', #28963, .T. ) ;
#51551=DIRECTION ( 'NONE',  ( 1.000000000000000000, -0.000000000000000000, -0.000000000000000000 ) ) ;
#51553=CARTESIAN_POINT ( 'NONE',  ( -336.3521761649654422, -110.9652333097088217, -57.67619951860654481 ) ) ;
#51558=ORIENTED_EDGE ( 'NONE', *, *, #40096, .T. ) ;
#51565=AXIS2_PLACEMENT_3D ( 'NONE', #35588, #31660, #3540 ) ;
#51566=CARTESIAN_POINT ( 'NONE',  ( -336.3521761649654422, -82.40546666720629787, 42.41660376256258047 ) ) ;
#51570=FACE_OUTER_BOUND ( 'NONE', #46889, .T. ) ;
#51573=EDGE_CURVE ( 'NONE', #18899, #42898, #14591, .T. ) ;
#51578=DIRECTION ( 'NONE',  ( -0.000000000000000000, 0.000000000000000000, 1.000000000000000000 ) ) ;
#51581=DIRECTION ( 'NONE',  ( 0.000000000000000000, -0.9350162426854107256, 0.3546048870425463906 ) ) ;
#51587=CARTESIAN_POINT ( 'NONE',  ( -332.3517673607765914, -145.9479049231020440, -54.58714071513102795 ) ) ;
#51592=VERTEX_POINT ( 'NONE', #15119 ) ;
#51596=EDGE_CURVE ( 'NONE', #39834, #6765, #34795, .T. ) ;
#51597=AXIS2_PLACEMENT_3D ( 'NONE', #45192, #9180, #49638 ) ;
#51616=EDGE_LOOP ( 'NONE', ( #48883, #45010, #48742, #18025 ) ) ;
#51618=EDGE_LOOP ( 'NONE', ( #47393, #31802, #24583, #2880 ) ) ;
#51619=DIRECTION ( 'NONE',  ( 1.000000000000000000, -0.000000000000000000, 0.000000000000000000 ) ) ;
#51620=PLANE ( 'NONE',  #14089 ) ;
#51621=ORIENTED_EDGE ( 'NONE', *, *, #36096, .T. ) ;
#51623=CARTESIAN_POINT ( 'NONE',  ( -339.1964088526558498, -89.57268800991437274, 48.27201571435973904 ) ) ;
#51628=DIRECTION ( 'NONE',  ( -1.000000000000000000, -0.000000000000000000, -0.000000000000000000 ) ) ;
#51631=EDGE_CURVE ( 'NONE', #153, #43387, #46924, .T. ) ;
#51633=EDGE_LOOP ( 'NONE', ( #23301, #2075, #18220, #12819 ) ) ;
#51637=DIRECTION ( 'NONE',  ( -1.000000000000000000, -0.000000000000000000, 0.000000000000000000 ) ) ;
#51650=CIRCLE ( 'NONE', #11339, 14.36509618646847386 ) ;
#51652=DIRECTION ( 'NONE',  ( -1.000000000000000000, 0.000000000000000000, 0.000000000000000000 ) ) ;
#51654=EDGE_CURVE ( 'NONE', #20241, #14966, #31898, .T. ) ;
#51655=VECTOR ( 'NONE', #12989, 1000.000000000000114 ) ;
#51658=EDGE_CURVE ( 'NONE', #25920, #13751, #43729, .T. ) ;
#51661=VECTOR ( 'NONE', #13601, 1000.000000000000000 ) ;
#51667=ORIENTED_EDGE ( 'NONE', *, *, #9515, .T. ) ;
#51669=DIRECTION ( 'NONE',  ( 0.000000000000000000, -1.288321301492108820E-13, 1.000000000000000000 ) ) ;
#51670=EDGE_CURVE ( 'NONE', #46650, #19973, #44255, .T. ) ;
#51674=ORIENTED_EDGE ( 'NONE', *, *, #30676, .F. ) ;
#51677=CARTESIAN_POINT ( 'NONE',  ( -330.4913330509368166, -102.1108035431471279, 54.98865587491800255 ) ) ;
#51684=ORIENTED_EDGE ( 'NONE', *, *, #6044, .T. ) ;
#51685=CIRCLE ( 'NONE', #44085, 60.00000000000000000 ) ;
#51686=ADVANCED_FACE ( 'NONE', ( #12691 ), #51620, .F. ) ;
#51691=VERTEX_POINT ( 'NONE', #19555 ) ;
#51699=AXIS2_PLACEMENT_3D ( 'NONE', #45169, #40934, #24390 ) ;
#51703=DIRECTION ( 'NONE',  ( -0.000000000000000000, 0.9350162426854194964, 0.3546048870425235200 ) ) ;
#51704=CARTESIAN_POINT ( 'NONE',  ( -339.1964088526558498, -156.6043281241916816, -48.84008046109114076 ) ) ;
#51705=ADVANCED_FACE ( 'NONE', ( #20589 ), #31638, .F. ) ;
#51710=ORIENTED_EDGE ( 'NONE', *, *, #34702, .F. ) ;
#51711=LINE ( 'NONE', #27769, #43938 ) ;
#51716=VECTOR ( 'NONE', #7104, 1000.000000000000000 ) ;
#51723=CARTESIAN_POINT ( 'NONE',  ( -339.1964088526558498, -71.02573290043878274, -26.97593913775585506 ) ) ;
#51724=ORIENTED_EDGE ( 'NONE', *, *, #1089, .F. ) ;
#51726=EDGE_CURVE ( 'NONE', #11608, #44829, #40285, .T. ) ;
#51730=ORIENTED_EDGE ( 'NONE', *, *, #15412, .F. ) ;
#51733=VECTOR ( 'NONE', #46523, 1000.000000000000000 ) ;
#51734=CARTESIAN_POINT ( 'NONE',  ( -332.3517673607765914, -111.7106844931459761, -58.83036664750484590 ) ) ;
#51736=ADVANCED_FACE ( 'NONE', ( #28206 ), #24279, .F. ) ;
#51739=PLANE ( 'NONE',  #1564 ) ;
#51740=ORIENTED_EDGE ( 'NONE', *, *, #5701, .T. ) ;
#51742=LINE ( 'NONE', #48044, #49857 ) ;
#51754=CARTESIAN_POINT ( 'NONE',  ( -339.1964088526558498, -157.4273119900845757, 48.27201571436049932 ) ) ;
#51759=DIRECTION ( 'NONE',  ( -0.000000000000000000, -0.9350162426854169428, -0.3546048870425300148 ) ) ;
#51760=DIRECTION ( 'NONE',  ( -0.000000000000000000, -0.8854560256532110207, -0.4647231720437664526 ) ) ;
#51762=LINE ( 'NONE', #3653, #48354 ) ;
#51764=CARTESIAN_POINT ( 'NONE',  ( -330.4913330509368166, -131.2283041299240836, 59.50019592636143528 ) ) ;
#51765=VECTOR ( 'NONE', #37711, 1000.000000000000000 ) ;
#51772=CIRCLE ( 'NONE', #6462, 60.00000000000000000 ) ;
#51774=ORIENTED_EDGE ( 'NONE', *, *, #40606, .T. ) ;
#51775=EDGE_CURVE ( 'NONE', #16302, #23663, #5695, .T. ) ;
#51779=CARTESIAN_POINT ( 'NONE',  ( -336.3521761649654422, -67.75522407825191351, 19.39547174791671935 ) ) ;
#51781=VECTOR ( 'NONE', #44182, 1000.000000000000000 ) ;
#51784=LINE ( 'NONE', #43873, #5548 ) ;
#51786=DIRECTION ( 'NONE',  ( 0.000000000000000000, -2.775557561562891351E-15, 1.000000000000000000 ) ) ;
#51790=VECTOR ( 'NONE', #34318, 1000.000000000000227 ) ;
#51792=AXIS2_PLACEMENT_3D ( 'NONE', #13705, #41037, #21068 ) ;
#51793=DIRECTION ( 'NONE',  ( 1.000000000000000000, -0.000000000000000000, -0.000000000000000000 ) ) ;
#51794=EDGE_CURVE ( 'NONE', #19072, #8637, #20863, .T. ) ;
#51797=AXIS2_PLACEMENT_3D ( 'NONE', #26112, #22181, #10867 ) ;
#51799=DIRECTION ( 'NONE',  ( -0.000000000000000000, 0.000000000000000000, -1.000000000000000000 ) ) ;
#51800=ADVANCED_FACE ( 'NONE', ( #45307 ), #33715, .T. ) ;
#51803=ORIENTED_EDGE ( 'NONE', *, *, #36804, .T. ) ;
#51804=AXIS2_PLACEMENT_3D ( 'NONE', #48185, #32141, #13218 ) ;
#51808=AXIS2_PLACEMENT_3D ( 'NONE', #7678, #23702, #39712 ) ;
#51809=CIRCLE ( 'NONE', #38362, 60.00000000000000000 ) ;
#51810=ORIENTED_EDGE ( 'NONE', *, *, #857, .T. ) ;
#51811=VECTOR ( 'NONE', #38095, 1000.000000000000000 ) ;
#51813=DIRECTION ( 'NONE',  ( -0.000000000000000000, 0.2393156642875547968, -0.9709418174260527890 ) ) ;
#51827=CARTESIAN_POINT ( 'NONE',  ( -330.4913330509368166, -123.5000000000000284, 0.000000000000000000 ) ) ;
#51831=PLANE ( 'NONE',  #48533 ) ;
#51834=DIRECTION ( 'NONE',  ( 0.000000000000000000, 1.000000000000000000, -3.491481338843133355E-15 ) ) ;
#51840=FACE_OUTER_BOUND ( 'NONE', #4482, .T. ) ;
#51842=LINE ( 'NONE', #51079, #7311 ) ;
#51843=ORIENTED_EDGE ( 'NONE', *, *, #50259, .F. ) ;
#51847=VECTOR ( 'NONE', #39945, 1000.000000000000114 ) ;
#51853=CARTESIAN_POINT ( 'NONE',  ( -330.0000000000000568, -123.5000000000000284, 0.000000000000000000 ) ) ;
#51854=CIRCLE ( 'NONE', #35761, 60.00000000000000000 ) ;
#51855=DIRECTION ( 'NONE',  ( -1.000000000000000000, 0.000000000000000000, 0.000000000000000000 ) ) ;
#51857=CARTESIAN_POINT ( 'NONE',  ( -339.1964088526558498, -67.57827586672178199, -21.74306257088745298 ) ) ;
#51863=CARTESIAN_POINT ( 'NONE',  ( 0.000000000000000000, -68.33404168156025094, 20.92168833550889673 ) ) ;
#51865=ORIENTED_EDGE ( 'NONE', *, *, #50436, .F. ) ;
#51874=CARTESIAN_POINT ( 'NONE',  ( -332.3517673607765914, -141.9604555052315220, 56.09938080879057765 ) ) ;
#51875=ORIENTED_EDGE ( 'NONE', *, *, #20498, .F. ) ;
#51883=DIRECTION ( 'NONE',  ( 0.000000000000000000, 0.000000000000000000, 1.000000000000000000 ) ) ;
#51884=VERTEX_POINT ( 'NONE', #48976 ) ;
#51893=VERTEX_POINT ( 'NONE', #13488 ) ;
#51898=DIRECTION ( 'NONE',  ( 0.000000000000000000, 2.914335439641035919E-13, -1.000000000000000000 ) ) ;
#51900=DIRECTION ( 'NONE',  ( 0.000000000000000000, -0.1205366802553164696, 0.9927088740980548609 ) ) ;
#51901=ORIENTED_EDGE ( 'NONE', *, *, #31033, .T. ) ;
#51905=EDGE_CURVE ( 'NONE', #38530, #50508, #9294, .T. ) ;
#51907=DIRECTION ( 'NONE',  ( -0.000000000000000000, -0.4647231720437724478, -0.8854560256532078011 ) ) ;
#51910=AXIS2_PLACEMENT_3D ( 'NONE', #13301, #13818, #21182 ) ;
#51912=VECTOR ( 'NONE', #5017, 1000.000000000000000 ) ;
#51914=DIRECTION ( 'NONE',  ( 0.000000000000000000, 0.000000000000000000, -1.000000000000000000 ) ) ;
#51916=CIRCLE ( 'NONE', #13296, 60.00000000000000000 ) ;
#51917=DIRECTION ( 'NONE',  ( 0.000000000000000000, 0.000000000000000000, -1.000000000000000000 ) ) ;
#51919=DIRECTION ( 'NONE',  ( 0.000000000000000000, 0.000000000000000000, 1.000000000000000000 ) ) ;
#51924=ORIENTED_EDGE ( 'NONE', *, *, #1467, .T. ) ;
#51926=PLANE ( 'NONE',  #33679 ) ;
#51931=VECTOR ( 'NONE', #6251, 1000.000000000000000 ) ;
#51935=PLANE ( 'NONE',  #6907 ) ;
#51936=EDGE_LOOP ( 'NONE', ( #26230, #37468, #18731, #47291 ) ) ;
#51942=ORIENTED_EDGE ( 'NONE', *, *, #50440, .T. ) ;
#51944=CARTESIAN_POINT ( 'NONE',  ( -336.3521761649653854, -183.2372378732723632, -5.609136410542876483 ) ) ;
#51948=VECTOR ( 'NONE', #33320, 1000.000000000000000 ) ;
#51950=PLANE ( 'NONE',  #9389 ) ;
#51953=VECTOR ( 'NONE', #34410, 1000.000000000000000 ) ;
#51960=ORIENTED_EDGE ( 'NONE', *, *, #14983, .T. ) ;
#51964=ADVANCED_FACE ( 'NONE', ( #46856 ), #34239, .F. ) ;
#51969=ADVANCED_FACE ( 'NONE', ( #50534 ), #15058, .F. ) ;
#51970=LINE ( 'NONE', #44334, #34261 ) ;
#51971=EDGE_LOOP ( 'NONE', ( #18100, #27681, #48463, #4863 ) ) ;
#51973=VECTOR ( 'NONE', #20139, 1000.000000000000000 ) ;
#51974=ORIENTED_EDGE ( 'NONE', *, *, #46544, .T. ) ;
#51982=CARTESIAN_POINT ( 'NONE',  ( -332.3517673607765914, -123.5000000000000284, 0.000000000000000000 ) ) ;
#51987=ORIENTED_EDGE ( 'NONE', *, *, #10908, .T. ) ;
#51988=AXIS2_PLACEMENT_3D ( 'NONE', #14184, #25992, #30438 ) ;
#51991=CARTESIAN_POINT ( 'NONE',  ( -336.3521761649654422, -123.5000000000000284, 0.000000000000000000 ) ) ;
#51994=VERTEX_POINT ( 'NONE', #30288 ) ;
#52001=AXIS2_PLACEMENT_3D ( 'NONE', #49459, #51900, #3786 ) ;
#52002=ORIENTED_EDGE ( 'NONE', *, *, #12101, .F. ) ;
#52003=EDGE_CURVE ( 'NONE', #25203, #903, #35009, .T. ) ;
#52004=DIRECTION ( 'NONE',  ( 0.000000000000000000, 0.000000000000000000, 1.000000000000000000 ) ) ;
#52007=CARTESIAN_POINT ( 'NONE',  ( -336.3521761649654422, -83.15397741537739762, 43.07972642080338233 ) ) ;
#52012=EDGE_CURVE ( 'NONE', #13290, #47261, #7151, .T. ) ;
#52014=CARTESIAN_POINT ( 'NONE',  ( -330.4913330509368166, -68.15673923803900891, 20.45418021416622878 ) ) ;
#52028=ADVANCED_FACE ( 'NONE', ( #20013 ), #51831, .T. ) ;
#52030=DIRECTION ( 'NONE',  ( -1.000000000000000000, 0.000000000000000000, -0.000000000000000000 ) ) ;
#52033=ORIENTED_EDGE ( 'NONE', *, *, #11166, .T. ) ;
#52034=DIRECTION ( 'NONE',  ( -1.000000000000000000, 0.000000000000000000, 0.000000000000000000 ) ) ;
#52035=PLANE ( 'NONE',  #30720 ) ;
#52040=CARTESIAN_POINT ( 'NONE',  ( -332.3517673607765914, -88.64083255475578937, 47.62880233550460218 ) ) ;
ENDSEC;
END-ISO-10303-21;
